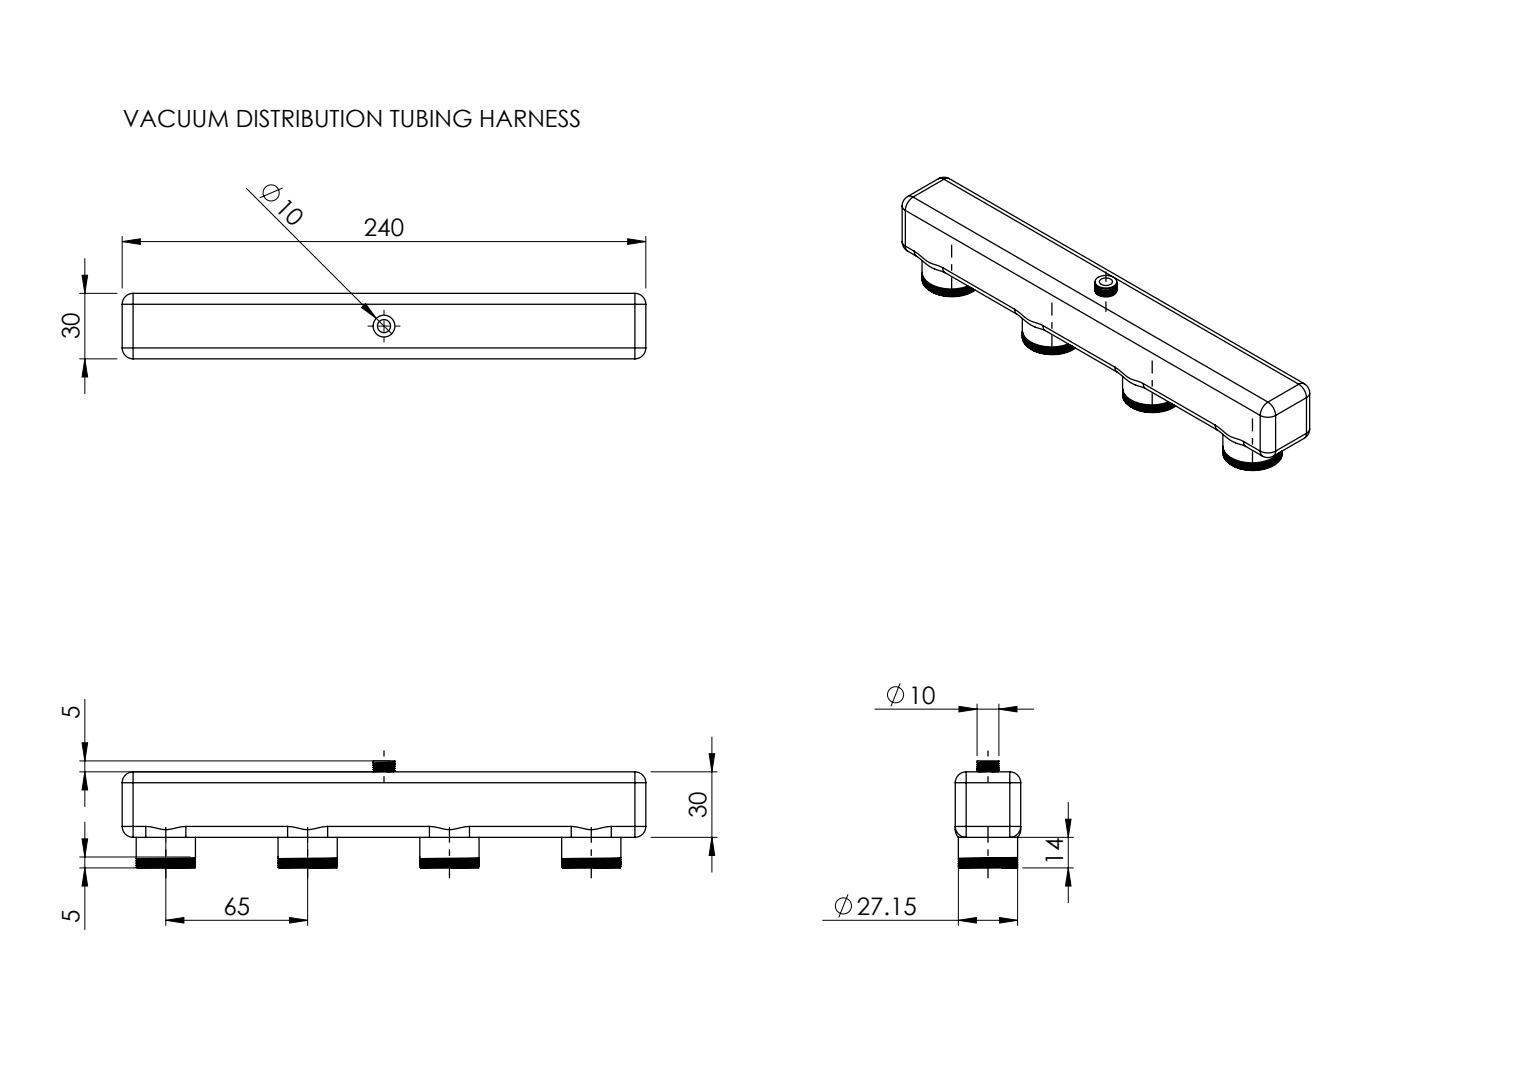
ISO-10303-21;
HEADER;
FILE_DESCRIPTION (('STEP AP214'),
    '1' );
FILE_NAME ('Vacuum Distribution Tubing Harness.step',
    '2026-10-01T14:18:43',
    ( '' ),
    ( '' ),
    'SwSTEP 2.0',
    'SolidWorks 2026',
    '' );
FILE_SCHEMA (( 'AUTOMOTIVE_DESIGN' ));
ENDSEC;

DATA;
#1=ORIENTED_EDGE ( 'NONE', *, *, #27439, .T. ) ;
#2=CARTESIAN_POINT ( 'NONE',  ( 94.99999999999995737, 83.93750000000001421, -2.071067811865491048 ) ) ;
#4=ORIENTED_EDGE ( 'NONE', *, *, #23222, .F. ) ;
#6=CARTESIAN_POINT ( 'NONE',  ( 59.55508561352770158, 34.55078125108393294, 13.14518615778179722 ) ) ;
#10=EDGE_CURVE ( 'NONE', #23304, #14872, #10315, .T. ) ;
#14=CARTESIAN_POINT ( 'NONE',  ( 185.4011555911795597, 37.22968750216787726, 9.598844408820459861 ) ) ;
#17=CARTESIAN_POINT ( 'NONE',  ( 198.0446094569239790, 53.89089363584123049, 14.99999999999994671 ) ) ;
#18=CARTESIAN_POINT ( 'NONE',  ( 143.1451861577818363, 36.43593750108394147, -5.444914386472297529 ) ) ;
#19=ORIENTED_EDGE ( 'NONE', *, *, #9159, .T. ) ;
#20=CARTESIAN_POINT ( 'NONE',  ( 13.14518615778179544, 37.97382812608393721, -1.609821015232357215E-15 ) ) ;
#22=CARTESIAN_POINT ( 'NONE',  ( 143.1451861577818079, 35.39414062608393152, -1.609821015232357215E-15 ) ) ;
#23=CARTESIAN_POINT ( 'NONE',  ( 65.00000000000000000, 34.84843749999999574, 13.57481594606304576 ) ) ;
#24=CARTESIAN_POINT ( 'NONE',  ( 130.0000000000000000, -7.395377635281828788, -1.503427012513233026E-14 ) ) ;
#29=CARTESIAN_POINT ( 'NONE',  ( -8.312177448680279460E-16, 39.31328125216787583, -13.57481594606304576 ) ) ;
#30=CARTESIAN_POINT ( 'NONE',  ( 99.99999999999995737, 80.00000000000000000, -1.387778780781445676E-14 ) ) ;
#32=CARTESIAN_POINT ( 'NONE',  ( -9.295050272127046043, 35.89023437608393152, -9.295050272127046043 ) ) ;
#39=CARTESIAN_POINT ( 'NONE',  ( 195.0000000000000000, 37.97382812608393721, -13.14518615778179544 ) ) ;
#40=ORIENTED_EDGE ( 'NONE', *, *, #17022, .F. ) ;
#50=CARTESIAN_POINT ( 'NONE',  ( 143.1451861577818079, 39.31328125108392868, 5.444914386472293977 ) ) ;
#54=CARTESIAN_POINT ( 'NONE',  ( 78.14518615778179367, 39.51171875108392584, 5.444914386472293977 ) ) ;
#55=FACE_OUTER_BOUND ( 'NONE', #22673, .T. ) ;
#56=CIRCLE ( 'NONE', #18273, 5.000000000000000000 ) ;
#57=CARTESIAN_POINT ( 'NONE',  ( 181.8548138422181921, 33.65781250108393152, 5.444914386472304635 ) ) ;
#59=ORIENTED_EDGE ( 'NONE', *, *, #2461, .T. ) ;
#62=CARTESIAN_POINT ( 'NONE',  ( 51.85481384221820633, 38.96601562608393721, 0.000000000000000000 ) ) ;
#63=CARTESIAN_POINT ( 'NONE',  ( 99.99999999999995737, 80.18750000136559208, -4.458734125000016313 ) ) ;
#64=CARTESIAN_POINT ( 'NONE',  ( 189.5550856135277229, 39.61093750108393152, -13.14518615778179722 ) ) ;
#66=CARTESIAN_POINT ( 'NONE',  ( 187.8845096081555823, 49.99999999945637796, 11.58166858714721492 ) ) ;
#70=ORIENTED_EDGE ( 'NONE', *, *, #20702, .F. ) ;
#75=CARTESIAN_POINT ( 'NONE',  ( 143.1451861577818079, 34.79882812608394005, -1.609821015232357215E-15 ) ) ;
#76=CARTESIAN_POINT ( 'NONE',  ( 59.55508561352770158, 32.76484375108393010, 13.14518615778179722 ) ) ;
#77=CARTESIAN_POINT ( 'NONE',  ( 208.1451861577817795, 38.71796875108393721, 5.444914386472293977 ) ) ;
#78=CARTESIAN_POINT ( 'NONE',  ( 9.295050272127047819, 32.91367187608393152, 9.295050272127046043 ) ) ;
#79=CARTESIAN_POINT ( 'NONE',  ( 134.5715916325255250, 51.44262710532316873, -14.99999999999934452 ) ) ;
#82=CARTESIAN_POINT ( 'NONE',  ( -9.180175813647991845, 50.00000000000000000, 9.999999999999998224 ) ) ;
#84=EDGE_CURVE ( 'NONE', #861, #22018, #1572, .T. ) ;
#85=CARTESIAN_POINT ( 'NONE',  ( 13.14518615778179544, 33.80664062608393294, -1.609821015232357215E-15 ) ) ;
#96=ADVANCED_FACE ( 'NONE', ( #24479 ), #13627, .T. ) ;
#98=CARTESIAN_POINT ( 'NONE',  ( 120.4011555911795455, 38.61875000216787157, -9.598844408820458085 ) ) ;
#99=CARTESIAN_POINT ( 'NONE',  ( 103.1528011352953342, 80.06250000136559208, 3.152801135295355106 ) ) ;
#100=CARTESIAN_POINT ( 'NONE',  ( 78.14518615778179367, 34.05468750108394005, -5.444914386472297529 ) ) ;
#103=CARTESIAN_POINT ( 'NONE',  ( 214.9999999999999716, 80.00000000000000000, 9.999999999999946709 ) ) ;
#105=CARTESIAN_POINT ( 'NONE',  ( 143.5748159460630404, 39.06523437499998863, -5.622872871577873077 ) ) ;
#110=CARTESIAN_POINT ( 'NONE',  ( 143.1451861577818079, 37.82500000108392868, -5.444914386472297529 ) ) ;
#111=CARTESIAN_POINT ( 'NONE',  ( 51.42518405393695957, 33.16171875216787868, 0.000000000000000000 ) ) ;
#112=EDGE_CURVE ( 'NONE', #21487, #10978, #25380, .T. ) ;
#114=CARTESIAN_POINT ( 'NONE',  ( 13.57481594606304931, 32.71523437716787441, 5.622872871577869525 ) ) ;
#117=CARTESIAN_POINT ( 'NONE',  ( 185.7049497278729575, 34.10429687608393579, -9.295050272127046043 ) ) ;
#121=CARTESIAN_POINT ( 'NONE',  ( 181.4251840539369596, 37.97382812716787726, 5.622872871577880183 ) ) ;
#122=LINE ( 'NONE', #8807, #24532 ) ;
#128=CARTESIAN_POINT ( 'NONE',  ( 195.0000000000000000, 35.24531249999999716, -13.57481594606304576 ) ) ;
#131=CARTESIAN_POINT ( 'NONE',  ( 59.55508561352770158, 35.14609375108393152, 13.14518615778179722 ) ) ;
#136=CARTESIAN_POINT ( 'NONE',  ( 13.57481594606304753, 36.68398437499999432, -5.622872871577873077 ) ) ;
#137=CARTESIAN_POINT ( 'NONE',  ( 130.0000000000000000, 36.58476562608393579, -13.14518615778179544 ) ) ;
#139=ORIENTED_EDGE ( 'NONE', *, *, #6013, .F. ) ;
#140=CARTESIAN_POINT ( 'NONE',  ( 99.99999999999995737, 84.75000000000000000, -5.000000000000018652 ) ) ;
#141=CARTESIAN_POINT ( 'NONE',  ( 94.99999999999995737, 82.06250000273119838, -2.071067811865491048 ) ) ;
#144=VERTEX_POINT ( 'NONE', #11771 ) ;
#145=AXIS2_PLACEMENT_3D ( 'NONE', #183, #21567, #25834 ) ;
#147=CARTESIAN_POINT ( 'NONE',  ( 70.44491438647230552, 33.85625000108393579, 13.14518615778179189 ) ) ;
#151=EDGE_CURVE ( 'NONE', #14316, #1074, #18349, .T. ) ;
#152=VERTEX_POINT ( 'NONE', #22777 ) ;
#153=CARTESIAN_POINT ( 'NONE',  ( 94.99999999999995737, 82.18750000273119838, 2.071067811865466624 ) ) ;
#156=CARTESIAN_POINT ( 'NONE',  ( 208.5748159460630120, 35.09648437716787583, 5.622872871577869525 ) ) ;
#157=( BOUNDED_CURVE ( )  B_SPLINE_CURVE ( 2, ( #25854, #26427, #8886, #8604, #23721, #4618, #22006, #19716, #2060, #6886, #24002, #4059, #2483, #19859, #12721, #10593, #17292, #17435, #26134, #346, #10730, #19438, #6600, #9033, #21447, #25994, #1925, #6465, #15139, #2204, #10868, #19578, #62, #5047, #2628, #15857, #775, #22576, #24851, #11571, #920, #7307, #13712, #7161, #13851, #491, #24419, #5188, #9172, #22433, #27146, #631, #15994, #4908, #9447, #11713, #24566, #3045, #9307, #11289, #17864, #20289, #22720, #26569, #9590, #18004, #2902, #24709, #20438, #7598, #18294, #7021, #27000, #7447, #16143, #22292, #24280, #5330, #4761, #13994, #3187, #13569, #11857, #20579, #2768, #26861, #18147, #1062, #15716, #9732, #18437, #13421, #11432 ),
 .UNSPECIFIED., .F., .F. ) 
 B_SPLINE_CURVE_WITH_KNOTS ( ( 3, 2, 2, 2, 2, 2, 2, 2, 2, 2, 2, 2, 2, 2, 2, 2, 2, 2, 2, 2, 2, 2, 2, 2, 2, 2, 2, 2, 2, 2, 2, 2, 2, 2, 2, 2, 2, 2, 2, 2, 2, 2, 2, 2, 2, 2, 3 ),
 ( 0.000000000000000000, 0.01041666666666666609, 0.02083333333333333218, 0.03125000000000000000, 0.04166666666666666435, 0.05208333333333333565, 0.06250000000000000000, 0.07291666666666667129, 0.08333333333333332871, 0.09375000000000000000, 0.1041666666666666713, 0.1145833333333333287, 0.1250000000000000000, 0.1354166666666666574, 0.1458333333333333426, 0.1562500000000000278, 0.1666666666666666574, 0.1770833333333333426, 0.1875000000000000000, 0.1979166666666666574, 0.2083333333333333426, 0.2187499999999999722, 0.2291666666666666574, 0.2395833333333333426, 0.2500000000000000000, 0.2604166666666666852, 0.2708333333333333148, 0.2812500000000000000, 0.2916666666666666852, 0.3020833333333333148, 0.3125000000000000555, 0.3229166666666666852, 0.3333333333333333148, 0.3437500000000000000, 0.3541666666666666852, 0.3645833333333333148, 0.3750000000000000000, 0.3854166666666666852, 0.3958333333333333148, 0.4062500000000000000, 0.4166666666666666852, 0.4270833333333333148, 0.4374999999999999445, 0.4479166666666666852, 0.4583333333333333148, 0.4687500000000000000, 0.4779971559588573893 ),
 .UNSPECIFIED. ) 
 CURVE ( )  GEOMETRIC_REPRESENTATION_ITEM ( )  RATIONAL_B_SPLINE_CURVE ( ( 1.000000000000000000, 0.9238795325112867385, 1.000000000000000000, 0.9238795325112867385, 1.000000000000000000, 0.9238795325112867385, 1.000000000000000000, 0.9238795325112867385, 1.000000000000000000, 0.9238795325112867385, 1.000000000000000000, 0.9238795325112867385, 1.000000000000000000, 0.9238795325112867385, 1.000000000000000000, 0.9238795325112867385, 1.000000000000000000, 0.9238795325112867385, 1.000000000000000000, 0.9238795325112867385, 1.000000000000000000, 0.9238795325112867385, 1.000000000000000000, 0.9238795325112867385, 1.000000000000000000, 0.9238795325112867385, 1.000000000000000000, 0.9238795325112867385, 1.000000000000000000, 0.9238795325112867385, 1.000000000000000000, 0.9238795325112867385, 1.000000000000000000, 0.9238795325112867385, 1.000000000000000000, 0.9238795325112867385, 1.000000000000000000, 0.9238795325112867385, 1.000000000000000000, 0.9238795325112867385, 1.000000000000000000, 0.9238795325112867385, 1.000000000000000000, 0.9238795325112867385, 1.000000000000000000, 0.9238795325112867385, 1.000000000000000000, 0.9238795325112867385, 1.000000000000000000, 0.9238795325112867385, 1.000000000000000000, 0.9238795325112867385, 1.000000000000000000, 0.9238795325112867385, 1.000000000000000000, 0.9238795325112867385, 1.000000000000000000, 0.9238795325112867385, 1.000000000000000000, 0.9238795325112867385, 1.000000000000000000, 0.9238795325112867385, 1.000000000000000000, 0.9238795325112867385, 1.000000000000000000, 0.9238795325112867385, 1.000000000000000000, 0.9238795325112867385, 1.000000000000000000, 0.9238795325112867385, 1.000000000000000000, 0.9238795325112867385, 1.000000000000000000, 0.9238795325112867385, 1.000000000000000000, 0.9238795325112867385, 1.000000000000000000, 0.9238795325112867385, 1.000000000000000000, 0.9238795325112867385, 1.000000000000000000, 0.9238795325112867385, 1.000000000000000000, 0.9238795325112867385, 1.000000000000000000, 0.9238795325112867385, 1.000000000000000000, 0.9238795325112867385, 1.000000000000000000, 0.9238795325112867385, 1.000000000000000000, 0.9324258078851906939, 0.9848264816800322841 ) ) 
 REPRESENTATION_ITEM ( '' )  );
#160=EDGE_CURVE ( 'NONE', #17655, #15436, #3245, .T. ) ;
#161=CARTESIAN_POINT ( 'NONE',  ( 204.5988444088204687, 39.80937500216786873, 9.598844408820456309 ) ) ;
#163=CARTESIAN_POINT ( 'NONE',  ( -13.14518615778179189, 36.83281250108393579, 5.444914386472304635 ) ) ;
#164=CARTESIAN_POINT ( 'NONE',  ( 130.0000000000000000, 36.38632812608393152, -13.14518615778179544 ) ) ;
#165=CARTESIAN_POINT ( 'NONE',  ( 65.00000000000000000, 35.64218749999999147, 13.57481594606304576 ) ) ;
#166=CARTESIAN_POINT ( 'NONE',  ( 9.598844408820456309, 38.42031250216787441, -9.598844408820458085 ) ) ;
#168=AXIS2_PLACEMENT_3D ( 'NONE', #6488, #12746, #4083 ) ;
#169=CARTESIAN_POINT ( 'NONE',  ( 195.0000000000000000, 37.22968749999999716, 13.57481594606304576 ) ) ;
#173=DIRECTION ( 'NONE',  ( 1.000000000000000000, 0.000000000000000000, 0.000000000000000000 ) ) ;
#175=CARTESIAN_POINT ( 'NONE',  ( -13.14518615778179900, 36.73359375108393010, -5.444914386472297529 ) ) ;
#180=LINE ( 'NONE', #8862, #20235 ) ;
#181=CARTESIAN_POINT ( 'NONE',  ( 185.7049497278729575, 38.27148437608393294, 9.295050272127047819 ) ) ;
#183=CARTESIAN_POINT ( 'NONE',  ( 0.000000000000000000, -7.395377635281828788, 0.000000000000000000 ) ) ;
#184=CARTESIAN_POINT ( 'NONE',  ( 189.6826484225240677, 54.47013368152370560, -15.00000000000000000 ) ) ;
#185=CARTESIAN_POINT ( 'NONE',  ( 143.5748159460630688, 39.85898437499999858, -5.622872871577873966 ) ) ;
#186=ORIENTED_EDGE ( 'NONE', *, *, #18586, .T. ) ;
#188=CARTESIAN_POINT ( 'NONE',  ( 130.0000000000000000, 37.62656249999999858, -13.57481594606304576 ) ) ;
#190=CARTESIAN_POINT ( 'NONE',  ( 130.0000000000000000, 31.37578125216787583, -13.57481594606304576 ) ) ;
#191=CARTESIAN_POINT ( 'NONE',  ( 13.14518615778179722, 40.30546875108393579, 5.444914386472293977 ) ) ;
#193=CARTESIAN_POINT ( 'NONE',  ( 51.85481384221820633, 37.57695312608393579, 0.000000000000000000 ) ) ;
#195=CARTESIAN_POINT ( 'NONE',  ( 189.5550856135277229, 36.13828125108393863, 13.14518615778179722 ) ) ;
#197=( BOUNDED_CURVE ( )  B_SPLINE_CURVE ( 2, ( #21878, #15145, #8893, #6748, #2489, #2066, #15434, #19866, #10736 ),
 .UNSPECIFIED., .F., .F. ) 
 B_SPLINE_CURVE_WITH_KNOTS ( ( 3, 2, 2, 2, 3 ),
 ( 0.1041666666666664909, 0.1145833333333332732, 0.1250000000000000833, 0.1354166666666668517, 0.1458333333333336757 ),
 .UNSPECIFIED. ) 
 CURVE ( )  GEOMETRIC_REPRESENTATION_ITEM ( )  RATIONAL_B_SPLINE_CURVE ( ( 1.000000000000001332, 0.9238795325112854062, 1.000000000000000000, 0.9238795325112867385, 1.000000000000000000, 0.9238795325112867385, 1.000000000000000000, 0.9238795325112842960, 1.000000000000002442 ) ) 
 REPRESENTATION_ITEM ( '' )  );
#198=ORIENTED_EDGE ( 'NONE', *, *, #2542, .F. ) ;
#202=CARTESIAN_POINT ( 'NONE',  ( 101.8468681455907046, 80.12500000136560629, -4.458734125000016313 ) ) ;
#203=CARTESIAN_POINT ( 'NONE',  ( 208.1451861577818079, 38.61875000108392442, -5.444914386472297529 ) ) ;
#206=CARTESIAN_POINT ( 'NONE',  ( 186.5976842187810973, 54.99999999484811752, 14.99999999999995026 ) ) ;
#208=DIRECTION ( 'NONE',  ( 0.000000000000000000, 0.000000000000000000, 1.000000000000000000 ) ) ;
#214=CARTESIAN_POINT ( 'NONE',  ( 116.8548138422182063, 35.93984375108393436, -5.444914386472297529 ) ) ;
#215=CARTESIAN_POINT ( 'NONE',  ( 78.14518615778179367, 33.75703125108393010, 5.444914386472293977 ) ) ;
#216=CARTESIAN_POINT ( 'NONE',  ( 189.5550856135277229, 35.84062500108394289, -13.14518615778179900 ) ) ;
#218=CARTESIAN_POINT ( 'NONE',  ( 66.13716782454086740, 35.99999999999998579, 13.09590655363602707 ) ) ;
#220=FACE_OUTER_BOUND ( 'NONE', #12562, .T. ) ;
#222=CARTESIAN_POINT ( 'NONE',  ( 65.00000000000000000, 40.40468749999999432, 13.57481594606304576 ) ) ;
#226=CARTESIAN_POINT ( 'NONE',  ( 61.88530225446237409, 53.90847045361019241, 14.99999999999997868 ) ) ;
#228=( NAMED_UNIT ( * ) PLANE_ANGLE_UNIT ( ) SI_UNIT ( $, .RADIAN. ) );
#232=CARTESIAN_POINT ( 'NONE',  ( 131.8143553545780264, 51.46618445021973542, 14.99999999999996625 ) ) ;
#234=PLANE ( 'NONE',  #26801 ) ;
#235=CARTESIAN_POINT ( 'NONE',  ( 95.54126587499995082, 80.62500000136559208, -1.846868145590750077 ) ) ;
#236=CARTESIAN_POINT ( 'NONE',  ( 65.00000000000000000, 35.39414062608393863, 13.14518615778179544 ) ) ;
#238=CARTESIAN_POINT ( 'NONE',  ( -5.444914386472297529, 36.43593750108394147, -13.14518615778179722 ) ) ;
#239=EDGE_CURVE ( 'NONE', #2183, #6189, #25460, .T. ) ;
#241=CARTESIAN_POINT ( 'NONE',  ( 116.4251840539369596, 40.65273437608393436, 0.000000000000000000 ) ) ;
#243=CARTESIAN_POINT ( 'NONE',  ( 130.0000000000000000, 38.81718749999999574, 13.57481594606304576 ) ) ;
#246=EDGE_CURVE ( 'NONE', #18432, #1781, #20836, .T. ) ;
#249=CARTESIAN_POINT ( 'NONE',  ( 143.1451861577818079, 36.93203125108394147, 5.444914386472293977 ) ) ;
#250=CARTESIAN_POINT ( 'NONE',  ( 74.59884440882045453, 34.45156250216787441, -9.598844408820458085 ) ) ;
#251=ORIENTED_EDGE ( 'NONE', *, *, #21153, .F. ) ;
#254=CARTESIAN_POINT ( 'NONE',  ( 2.493653234604083739E-15, 32.56640625216787299, 13.57481594606304576 ) ) ;
#258=CARTESIAN_POINT ( 'NONE',  ( 189.5550856135277229, 35.14609375108393152, 13.14518615778179722 ) ) ;
#260=AXIS2_PLACEMENT_3D ( 'NONE', #16112, #26536, #3014 ) ;
#262=CARTESIAN_POINT ( 'NONE',  ( 99.99999999999995737, 81.25000000000000000, 4.999999999999990230 ) ) ;
#267=CARTESIAN_POINT ( 'NONE',  ( 139.5988444088204403, 38.32109374999999574, -9.598844408820458085 ) ) ;
#270=CARTESIAN_POINT ( 'NONE',  ( 208.5748159460630120, 35.09648437499998863, -5.622872871577873077 ) ) ;
#271=CARTESIAN_POINT ( 'NONE',  ( 204.1801758136480203, 55.00000000000014211, 9.999999999999948486 ) ) ;
#272=CARTESIAN_POINT ( 'NONE',  ( 139.5988444088204403, 36.73359374999999716, -9.598844408820458085 ) ) ;
#273=CARTESIAN_POINT ( 'NONE',  ( 74.29505027212704249, 35.49335937608393010, -9.295050272127046043 ) ) ;
#277=ADVANCED_FACE ( 'NONE', ( #16895 ), #6077, .T. ) ;
#278=DIRECTION ( 'NONE',  ( 0.000000000000000000, -1.000000000000000000, 0.000000000000000000 ) ) ;
#279=CARTESIAN_POINT ( 'NONE',  ( 2.493653234604083739E-15, 35.64218749999999147, 13.57481594606304576 ) ) ;
#280=CARTESIAN_POINT ( 'NONE',  ( 139.2950502721270425, 37.27929687608394005, -9.295050272127046043 ) ) ;
#283=CARTESIAN_POINT ( 'NONE',  ( 104.9999999999999574, 83.56250000000002842, -2.071067811865491937 ) ) ;
#284=CARTESIAN_POINT ( 'NONE',  ( 96.46446609406721961, 80.25000000273119838, 3.535533905932727539 ) ) ;
#287=CARTESIAN_POINT ( 'NONE',  ( 51.85082601884828080, 35.99999999999999289, -1.058935892997133088 ) ) ;
#290=CARTESIAN_POINT ( 'NONE',  ( 59.37712712842213136, 40.85117187499999147, -13.57481594606304753 ) ) ;
#291=VERTEX_POINT ( 'NONE', #25731 ) ;
#292=CARTESIAN_POINT ( 'NONE',  ( 139.5988444088204403, 39.21406250216787015, -9.598844408820458085 ) ) ;
#294=EDGE_CURVE ( 'NONE', #22062, #7806, #16625, .T. ) ;
#296=CARTESIAN_POINT ( 'NONE',  ( 120.8198241863519939, 50.00000000000000000, -9.999999999999998224 ) ) ;
#298=CARTESIAN_POINT ( 'NONE',  ( 181.4251840539369596, 33.90585937716787868, -5.622872871577873077 ) ) ;
#299=AXIS2_PLACEMENT_3D ( 'NONE', #13990, #23131, #5887 ) ;
#302=CARTESIAN_POINT ( 'NONE',  ( 143.1451861577818363, 37.13046875108393863, 5.444914386472293977 ) ) ;
#303=ORIENTED_EDGE ( 'NONE', *, *, #24870, .F. ) ;
#304=CARTESIAN_POINT ( 'NONE',  ( 9.295050272127046043, 34.89804687608393863, -9.295050272127046043 ) ) ;
#305=CARTESIAN_POINT ( 'NONE',  ( 124.5550856135277087, 35.14609375108393152, 13.14518615778179722 ) ) ;
#306=CARTESIAN_POINT ( 'NONE',  ( 59.37712712842213136, 35.29492187500000000, -13.57481594606304753 ) ) ;
#310=DIRECTION ( 'NONE',  ( -0.000000000000000000, 1.000000000000000000, -0.000000000000000000 ) ) ;
#316=CARTESIAN_POINT ( 'NONE',  ( 5.444914386472302859, 37.82500000108392868, 13.14518615778179189 ) ) ;
#318=ORIENTED_EDGE ( 'NONE', *, *, #24476, .T. ) ;
#320=( BOUNDED_CURVE ( )  B_SPLINE_CURVE ( 2, ( #29, #14971, #10973, #15395, #28107, #8572, #17262, #24107, #13244 ),
 .UNSPECIFIED., .F., .T. ) 
 B_SPLINE_CURVE_WITH_KNOTS ( ( 3, 2, 2, 2, 3 ),
 ( 0.1041666666666664909, 0.1145833333333332732, 0.1250000000000000833, 0.1354166666666668517, 0.1458333333333336757 ),
 .UNSPECIFIED. ) 
 CURVE ( )  GEOMETRIC_REPRESENTATION_ITEM ( )  RATIONAL_B_SPLINE_CURVE ( ( 1.000000000000001332, 0.9238795325112854062, 1.000000000000000000, 0.9238795325112867385, 1.000000000000000000, 0.9238795325112867385, 1.000000000000000000, 0.9238795325112842960, 1.000000000000002442 ) ) 
 REPRESENTATION_ITEM ( '' )  );
#321=AXIS2_PLACEMENT_3D ( 'NONE', #9134, #9413, #17827 ) ;
#325=CARTESIAN_POINT ( 'NONE',  ( 181.8548138422181921, 39.01562500108393294, 5.444914386472304635 ) ) ;
#326=ORIENTED_EDGE ( 'NONE', *, *, #10011, .F. ) ;
#327=CARTESIAN_POINT ( 'NONE',  ( 135.6228728715780107, 36.08867187716787583, -13.57481594606290898 ) ) ;
#333=CARTESIAN_POINT ( 'NONE',  ( 143.5748159460630404, 31.92148437716787512, 5.622872871577869525 ) ) ;
#334=DIRECTION ( 'NONE',  ( -0.000000000000000000, 1.000000000000000000, -0.000000000000000000 ) ) ;
#337=CARTESIAN_POINT ( 'NONE',  ( 74.29505027212704249, 37.87460937608393863, 9.295050272127046043 ) ) ;
#338=CARTESIAN_POINT ( 'NONE',  ( 64.55395874322236693, 49.99999999978093257, -13.57776691409252656 ) ) ;
#339=CARTESIAN_POINT ( 'NONE',  ( 189.3771271284221314, 40.35507812499998437, 13.57481594606304753 ) ) ;
#340=CARTESIAN_POINT ( 'NONE',  ( 77.25119088044421289, 35.99999999999997158, 5.405483146088426061 ) ) ;
#346=CARTESIAN_POINT ( 'NONE',  ( 59.55508561352770158, 39.61093750108393152, -13.14518615778179722 ) ) ;
#347=CARTESIAN_POINT ( 'NONE',  ( 103.1528011352953342, 82.81250000136560629, 3.152801135295355106 ) ) ;
#348=CARTESIAN_POINT ( 'NONE',  ( 189.5550856135277229, 38.32109375108394289, 13.14518615778179722 ) ) ;
#350=CARTESIAN_POINT ( 'NONE',  ( 186.7886859848165102, 50.68678854790359622, 14.99999999999995737 ) ) ;
#351=DIRECTION ( 'NONE',  ( 0.000000000000000000, 0.000000000000000000, -1.000000000000000000 ) ) ;
#352=CARTESIAN_POINT ( 'NONE',  ( 208.1451861577818079, 40.40468750108393436, -5.444914386472297529 ) ) ;
#357=ORIENTED_EDGE ( 'NONE', *, *, #27287, .T. ) ;
#358=CARTESIAN_POINT ( 'NONE',  ( 116.8548138422182063, 34.35234375108393579, -5.444914386472297529 ) ) ;
#360=CARTESIAN_POINT ( 'NONE',  ( 74.29505027212704249, 34.69960937608393436, -9.295050272127046043 ) ) ;
#361=CARTESIAN_POINT ( 'NONE',  ( 181.8548138422182205, 38.37070312608393152, 0.000000000000000000 ) ) ;
#362=ORIENTED_EDGE ( 'NONE', *, *, #430, .T. ) ;
#363=CARTESIAN_POINT ( 'NONE',  ( 99.99999999999995737, 80.00000000000000000, -1.387778780781445676E-14 ) ) ;
#364=CARTESIAN_POINT ( 'NONE',  ( 5.444914386472302859, 32.07031250108393294, 13.14518615778179189 ) ) ;
#366=CARTESIAN_POINT ( 'NONE',  ( 78.57481594606305464, 40.65273437499999432, -5.622872871577873966 ) ) ;
#368=EDGE_CURVE ( 'NONE', #4636, #22369, #10615, .T. ) ;
#369=( BOUNDED_CURVE ( )  B_SPLINE_CURVE ( 2, ( #25306, #14184, #6305, #9907, #1384, #3231, #14981, #3653, #12315 ),
 .UNSPECIFIED., .F., .F. ) 
 B_SPLINE_CURVE_WITH_KNOTS ( ( 3, 2, 2, 2, 3 ),
 ( 0.05000000000000004441, 0.07500000000000006661, 0.1000000000000000888, 0.1250000000000001110, 0.1500000000000001332 ),
 .UNSPECIFIED. ) 
 CURVE ( )  GEOMETRIC_REPRESENTATION_ITEM ( )  RATIONAL_B_SPLINE_CURVE ( ( 0.9999999999999998890, 0.9238795325112868495, 1.000000000000000000, 0.9238795325112867385, 1.000000000000000000, 0.9238795325112867385, 1.000000000000000000, 0.9238795325112862944, 1.000000000000000444 ) ) 
 REPRESENTATION_ITEM ( '' )  );
#373=CARTESIAN_POINT ( 'NONE',  ( 57.88450960814756030, 49.99999999945625717, 11.58166858714126235 ) ) ;
#382=CARTESIAN_POINT ( 'NONE',  ( 95.54126587499995082, 82.75000000136560629, 1.846868145590724986 ) ) ;
#383=CARTESIAN_POINT ( 'NONE',  ( 65.00000000000000000, 36.18789062608393436, 13.14518615778179544 ) ) ;
#385=CARTESIAN_POINT ( 'NONE',  ( -13.14518615778179544, 36.58476562608393579, 0.000000000000000000 ) ) ;
#390=CARTESIAN_POINT ( 'NONE',  ( 116.4251840539369454, 37.77539062499999289, -5.622872871577873077 ) ) ;
#392=ORIENTED_EDGE ( 'NONE', *, *, #14583, .T. ) ;
#397=CARTESIAN_POINT ( 'NONE',  ( 124.5550856135277087, 37.52734375108393294, 13.14518615778179722 ) ) ;
#398=CARTESIAN_POINT ( 'NONE',  ( 51.42518405393695957, 33.11210937716786873, -5.622872871577873077 ) ) ;
#401=CARTESIAN_POINT ( 'NONE',  ( -13.57481594606304576, 33.95546875216787441, 0.000000000000000000 ) ) ;
#402=CIRCLE ( 'NONE', #16324, 11.57481594606304398 ) ;
#404=AXIS2_PLACEMENT_3D ( 'NONE', #9924, #14615, #3535 ) ;
#405=CARTESIAN_POINT ( 'NONE',  ( 181.8548138422182205, 34.99726562608393721, 0.000000000000000000 ) ) ;
#408=CARTESIAN_POINT ( 'NONE',  ( 189.3771271284220745, 40.05742187499998863, -13.57481594606297293 ) ) ;
#410=CARTESIAN_POINT ( 'NONE',  ( 120.8198241863519939, 55.00000000000000000, 14.99999999999996803 ) ) ;
#412=CARTESIAN_POINT ( 'NONE',  ( 135.6228728715778118, 38.07304687499999574, 13.57481594606313813 ) ) ;
#415=CARTESIAN_POINT ( 'NONE',  ( 181.4251840539369596, 33.11210937499999574, 5.622872871577880183 ) ) ;
#417=CARTESIAN_POINT ( 'NONE',  ( 70.44491438647230552, 36.83281250108392868, 13.14518615778179189 ) ) ;
#421=CARTESIAN_POINT ( 'NONE',  ( -9.598844408820454532, 34.74921874999999716, 9.598844408820459861 ) ) ;
#422=CARTESIAN_POINT ( 'NONE',  ( 143.1451861577818079, 38.76757812608393294, -1.609821015232357215E-15 ) ) ;
#423=ORIENTED_EDGE ( 'NONE', *, *, #17964, .T. ) ;
#424=CARTESIAN_POINT ( 'NONE',  ( 102.0710678118654329, 82.68750000000001421, -5.000000000000018652 ) ) ;
#425=CARTESIAN_POINT ( 'NONE',  ( 219.9999999999999716, 50.00000000000000000, -10.00000000000000000 ) ) ;
#426=CARTESIAN_POINT ( 'NONE',  ( 103.5355339059327093, 83.50000000273119838, 3.535533905932726206 ) ) ;
#430=EDGE_CURVE ( 'NONE', #1457, #22555, #4820, .T. ) ;
#432=CARTESIAN_POINT ( 'NONE',  ( 59.37712712842213136, 39.56132812499999574, 13.57481594606304753 ) ) ;
#436=EDGE_LOOP ( 'NONE', ( #17651, #5409, #22660, #15371, #2602 ) ) ;
#438=CARTESIAN_POINT ( 'NONE',  ( 189.3771271284221314, 33.31054687716787299, 13.57481594606304753 ) ) ;
#439=VERTEX_POINT ( 'NONE', #6346 ) ;
#440=EDGE_CURVE ( 'NONE', #5976, #21288, #23550, .T. ) ;
#443=CARTESIAN_POINT ( 'NONE',  ( 124.5550856135277087, 36.93203125108394147, 13.14518615778179722 ) ) ;
#444=VERTEX_POINT ( 'NONE', #16759 ) ;
#445=CARTESIAN_POINT ( 'NONE',  ( 13.14518615778179900, 33.95546875108393436, 5.444914386472293977 ) ) ;
#447=CARTESIAN_POINT ( 'NONE',  ( 120.7049497278729575, 32.51679687608393721, -9.295050272127046043 ) ) ;
#448=CARTESIAN_POINT ( 'NONE',  ( 78.57481594606304043, 34.30273437500000000, -5.622872871577873077 ) ) ;
#450=AXIS2_PLACEMENT_3D ( 'NONE', #25758, #24046, #13329 ) ;
#453=FACE_OUTER_BOUND ( 'NONE', #21146, .T. ) ;
#457=CARTESIAN_POINT ( 'NONE',  ( 102.0710678118654187, 83.81250000273119838, -5.000000000000015987 ) ) ;
#459=CARTESIAN_POINT ( 'NONE',  ( -5.444914386472299306, 36.13828125108393863, 13.14518615778179722 ) ) ;
#462=ORIENTED_EDGE ( 'NONE', *, *, #14982, .F. ) ;
#466=CARTESIAN_POINT ( 'NONE',  ( 189.5550856135277229, 37.22968750108393721, -13.14518615778179900 ) ) ;
#467=VERTEX_POINT ( 'NONE', #26304 ) ;
#468=CARTESIAN_POINT ( 'NONE',  ( 13.57481594606304753, 39.95820312716787726, -5.622872871577873966 ) ) ;
#477=CARTESIAN_POINT ( 'NONE',  ( 143.5748159460630688, 32.76484375216787015, -1.662435489736055892E-15 ) ) ;
#478=CARTESIAN_POINT ( 'NONE',  ( 9.295050272127047819, 39.46210937608393721, 9.295050272127046043 ) ) ;
#479=EDGE_CURVE ( 'NONE', #25975, #2330, #24301, .T. ) ;
#481=CARTESIAN_POINT ( 'NONE',  ( 55.70494972787295751, 38.27148437608393294, -9.295050272127046043 ) ) ;
#482=CARTESIAN_POINT ( 'NONE',  ( 62.97537227446170505, 50.00000000051003468, -13.43320860980927201 ) ) ;
#485=CARTESIAN_POINT ( 'NONE',  ( 189.5550856135277229, 31.87187500108393223, -13.14518615778179900 ) ) ;
#491=CARTESIAN_POINT ( 'NONE',  ( 59.55508561352770158, 38.32109375108394289, 13.14518615778179722 ) ) ;
#492=DIRECTION ( 'NONE',  ( -0.000000000000000000, 1.000000000000000000, -0.000000000000000000 ) ) ;
#494=AXIS2_PLACEMENT_3D ( 'NONE', #24, #21266, #25957 ) ;
#497=CARTESIAN_POINT ( 'NONE',  ( 200.4449143864723055, 36.53515625108394715, -13.14518615778179722 ) ) ;
#503=CARTESIAN_POINT ( 'NONE',  ( 116.8548138422182063, 32.07031250108393294, 5.444914386472304635 ) ) ;
#504=CARTESIAN_POINT ( 'NONE',  ( 51.85481384221820633, 35.04687500108393294, 5.444914386472304635 ) ) ;
#505=CARTESIAN_POINT ( 'NONE',  ( 208.1451861577818079, 36.38632812608393863, -1.609821015232357215E-15 ) ) ;
#506=VERTEX_POINT ( 'NONE', #11310 ) ;
#508=CARTESIAN_POINT ( 'NONE',  ( -9.295050272127044266, 33.50898437608393010, 9.295050272127047819 ) ) ;
#511=CARTESIAN_POINT ( 'NONE',  ( 124.3771271284221314, 39.36289062716787157, -13.57481594606304753 ) ) ;
#515=CARTESIAN_POINT ( 'NONE',  ( 208.1451861577817795, 39.61093750108393863, -5.444914386472297529 ) ) ;
#518=ORIENTED_EDGE ( 'NONE', *, *, #16489, .T. ) ;
#521=CARTESIAN_POINT ( 'NONE',  ( 139.1801758136480203, 50.00000000000000000, 9.999999999999953815 ) ) ;
#523=CARTESIAN_POINT ( 'NONE',  ( 74.59884440882045453, 39.01562500216787299, 9.598844408820456309 ) ) ;
#525=CARTESIAN_POINT ( 'NONE',  ( 59.55508561352770158, 35.34453125108393579, 13.14518615778179722 ) ) ;
#527=CARTESIAN_POINT ( 'NONE',  ( 5.444914386472297529, 38.71796875108393721, -13.14518615778179722 ) ) ;
#529=CARTESIAN_POINT ( 'NONE',  ( 6.085944215996224038, 54.65299103241510892, 14.99999999999999289 ) ) ;
#531=CARTESIAN_POINT ( 'NONE',  ( 139.5988444088204403, 37.52734375000000000, -9.598844408820458085 ) ) ;
#533=EDGE_LOOP ( 'NONE', ( #3888, #18754, #1481 ) ) ;
#534=DIRECTION ( 'NONE',  ( 0.000000000000000000, -1.000000000000000000, 0.000000000000000000 ) ) ;
#538=CARTESIAN_POINT ( 'NONE',  ( 124.5550856135277087, 33.55859375108393294, 13.14518615778179722 ) ) ;
#539=CARTESIAN_POINT ( 'NONE',  ( 51.42518405393695957, 34.69960937716787441, -5.622872871577873077 ) ) ;
#540=VERTEX_POINT ( 'NONE', #15739 ) ;
#541=( BOUNDED_CURVE ( )  B_SPLINE_CURVE ( 2, ( #6091, #14214, #10070, #8082, #18782 ),
 .UNSPECIFIED., .F., .F. ) 
 B_SPLINE_CURVE_WITH_KNOTS ( ( 3, 2, 3 ),
 ( 0.9500000000000009548, 0.9750000000000005329, 1.000000000000000000 ),
 .UNSPECIFIED. ) 
 CURVE ( )  GEOMETRIC_REPRESENTATION_ITEM ( )  RATIONAL_B_SPLINE_CURVE ( ( 0.9999999999999970024, 0.9238795325112897361, 1.000000000000000000, 0.9238795325112867385, 1.000000000000000000 ) ) 
 REPRESENTATION_ITEM ( '' )  );
#542=CARTESIAN_POINT ( 'NONE',  ( 219.9999999999999716, 55.00000000000000000, 14.99999999999994316 ) ) ;
#543=CARTESIAN_POINT ( 'NONE',  ( 13.57481594606304576, 32.76484375216787015, -1.662435489736055892E-15 ) ) ;
#547=CARTESIAN_POINT ( 'NONE',  ( 181.8548138422182205, 33.40976562608393863, 0.000000000000000000 ) ) ;
#552=CARTESIAN_POINT ( 'NONE',  ( 116.4251840539369596, 36.33671875216787583, 0.000000000000000000 ) ) ;
#553=FACE_OUTER_BOUND ( 'NONE', #16139, .T. ) ;
#558=CARTESIAN_POINT ( 'NONE',  ( 181.4251840539369596, 33.90585937500000568, 5.622872871577880183 ) ) ;
#562=CARTESIAN_POINT ( 'NONE',  ( 55.70494972787295751, 35.89023437608393152, 9.295050272127047819 ) ) ;
#563=CARTESIAN_POINT ( 'NONE',  ( 99.99999999999995737, 85.00000000000000000, -1.387778780781445676E-14 ) ) ;
#564=DIRECTION ( 'NONE',  ( -0.000000000000000000, 1.000000000000000000, -0.000000000000000000 ) ) ;
#567=CARTESIAN_POINT ( 'NONE',  ( -9.598844408820458085, 35.34453124999998863, -9.598844408820458085 ) ) ;
#568=CARTESIAN_POINT ( 'NONE',  ( 143.1451861577818079, 38.81718750108393579, -5.444914386472297529 ) ) ;
#569=ORIENTED_EDGE ( 'NONE', *, *, #14895, .T. ) ;
#570=CARTESIAN_POINT ( 'NONE',  ( 102.0710678118654329, 81.68750000000000000, -5.000000000000018652 ) ) ;
#573=CARTESIAN_POINT ( 'NONE',  ( 103.5355339059327093, 83.75000000273119838, -3.535533905932755072 ) ) ;
#577=CARTESIAN_POINT ( 'NONE',  ( 70.62287287157786864, 40.75195312500000711, -13.57481594606304753 ) ) ;
#585=CARTESIAN_POINT ( 'NONE',  ( 185.4011555911795313, 33.06250000216787299, -9.598844408820458085 ) ) ;
#587=CARTESIAN_POINT ( 'NONE',  ( 200.6228728715780107, 36.08867187716787583, -13.57481594606290898 ) ) ;
#589=CARTESIAN_POINT ( 'NONE',  ( 13.14518615778179900, 35.64218750108393152, -5.444914386472297529 ) ) ;
#590=CARTESIAN_POINT ( 'NONE',  ( 116.8548138422182205, 31.82226562608393650, 0.000000000000000000 ) ) ;
#591=CARTESIAN_POINT ( 'NONE',  ( 65.00000000000000000, 33.26093749999999716, 13.57481594606304576 ) ) ;
#593=CARTESIAN_POINT ( 'NONE',  ( 122.9316343120017194, 36.00000000000003553, 11.09140360074130705 ) ) ;
#595=CARTESIAN_POINT ( 'NONE',  ( 207.0772764098356049, 36.00000000000000000, -6.197985357349214297 ) ) ;
#601=CARTESIAN_POINT ( 'NONE',  ( 5.444914386472297529, 37.32890625108393579, -13.14518615778179900 ) ) ;
#608=EDGE_CURVE ( 'NONE', #15564, #13869, #4643, .T. ) ;
#609=CARTESIAN_POINT ( 'NONE',  ( 208.1451861577818079, 35.39414062608393152, -1.609821015232357215E-15 ) ) ;
#610=ORIENTED_EDGE ( 'NONE', *, *, #1683, .F. ) ;
#611=CARTESIAN_POINT ( 'NONE',  ( 203.4023157812191300, 54.99999999485618929, -14.99999999999999645 ) ) ;
#618=EDGE_CURVE ( 'NONE', #28009, #5791, #13088, .T. ) ;
#619=CARTESIAN_POINT ( 'NONE',  ( 120.7049497278729575, 38.86679687608393863, -9.295050272127046043 ) ) ;
#620=LINE ( 'NONE', #26269, #12057 ) ;
#621=CARTESIAN_POINT ( 'NONE',  ( 5.444914386472297529, 35.54296875108393294, -13.14518615778179900 ) ) ;
#624=CARTESIAN_POINT ( 'NONE',  ( 78.14518615778179367, 38.02343750108395426, -5.444914386472297529 ) ) ;
#625=CARTESIAN_POINT ( 'NONE',  ( 55.81982418635199394, 49.99999999999999289, -14.99999999999999822 ) ) ;
#627=CARTESIAN_POINT ( 'NONE',  ( 181.8548138422182205, 32.81445312608393294, 0.000000000000000000 ) ) ;
#631=CARTESIAN_POINT ( 'NONE',  ( 59.55508561352770158, 38.02343750108394005, -13.14518615778179722 ) ) ;
#633=CARTESIAN_POINT ( 'NONE',  ( 65.00000000000000000, 38.81718749999999574, 13.57481594606304576 ) ) ;
#634=CARTESIAN_POINT ( 'NONE',  ( 208.1451861577818079, 36.18789062608393436, -1.609821015232357215E-15 ) ) ;
#635=EDGE_LOOP ( 'NONE', ( #198, #4757, #6902, #2298 ) ) ;
#639=CARTESIAN_POINT ( 'NONE',  ( 181.8548138422182205, 38.32109375108394289, -5.444914386472297529 ) ) ;
#646=CARTESIAN_POINT ( 'NONE',  ( 130.0000000000000000, 33.80664062608393294, 13.14518615778179544 ) ) ;
#647=CARTESIAN_POINT ( 'NONE',  ( 70.44491438647230552, 32.07031250108393294, 13.14518615778179189 ) ) ;
#648=EDGE_CURVE ( 'NONE', #24292, #15569, #2303, .T. ) ;
#649=CARTESIAN_POINT ( 'NONE',  ( 195.0000000000000000, 33.80664062608393294, 13.14518615778179544 ) ) ;
#652=CARTESIAN_POINT ( 'NONE',  ( -0.3969994146497772824, 51.45716825712459297, -15.00000000000033573 ) ) ;
#654=CARTESIAN_POINT ( 'NONE',  ( 65.00000000000000000, 36.00000000000000000, -7.517135062566165128E-15 ) ) ;
#656=( BOUNDED_CURVE ( )  B_SPLINE_CURVE ( 2, ( #15903, #27198, #9360, #11907, #14190, #4961, #20631, #9782, #7650 ),
 .UNSPECIFIED., .F., .T. ) 
 B_SPLINE_CURVE_WITH_KNOTS ( ( 3, 2, 2, 2, 3 ),
 ( 0.2708333333333330928, 0.2812499999999998890, 0.2916666666666666852, 0.3020833333333334259, 0.3125000000000002220 ),
 .UNSPECIFIED. ) 
 CURVE ( )  GEOMETRIC_REPRESENTATION_ITEM ( )  RATIONAL_B_SPLINE_CURVE ( ( 1.000000000000001554, 0.9238795325112850731, 1.000000000000000000, 0.9238795325112867385, 1.000000000000000000, 0.9238795325112867385, 1.000000000000000000, 0.9238795325112850731, 1.000000000000001554 ) ) 
 REPRESENTATION_ITEM ( '' )  );
#657=FACE_OUTER_BOUND ( 'NONE', #19869, .T. ) ;
#659=CARTESIAN_POINT ( 'NONE',  ( 208.1451861577818079, 40.35507812608393863, -1.609821015232357215E-15 ) ) ;
#663=EDGE_LOOP ( 'NONE', ( #12558, #2041, #9546, #25011 ) ) ;
#666=CARTESIAN_POINT ( 'NONE',  ( 138.3959387413077593, 54.99999999495823744, 14.99999999999996092 ) ) ;
#669=CARTESIAN_POINT ( 'NONE',  ( 78.14518615778179367, 33.21132812608393436, -1.609821015232357215E-15 ) ) ;
#672=CARTESIAN_POINT ( 'NONE',  ( -8.049105076161786076E-16, 37.97382812608393721, -13.14518615778179544 ) ) ;
#673=CIRCLE ( 'NONE', #4302, 5.000000000000000888 ) ;
#675=CARTESIAN_POINT ( 'NONE',  ( -3.863925265120440322, 54.10645156200380512, 14.99999999999999645 ) ) ;
#676=CARTESIAN_POINT ( 'NONE',  ( 135.6228728715778971, 40.45429687500001137, 13.57481594606306174 ) ) ;
#677=CARTESIAN_POINT ( 'NONE',  ( 143.5748159460630688, 37.42812499999999432, -1.662435489736055892E-15 ) ) ;
#683=CARTESIAN_POINT ( 'NONE',  ( 116.8548138422182063, 31.87187500108393223, 5.444914386472304635 ) ) ;
#684=CARTESIAN_POINT ( 'NONE',  ( 59.55508561352770158, 38.81718750108393579, -13.14518615778179900 ) ) ;
#686=CARTESIAN_POINT ( 'NONE',  ( -9.598844408820458085, 32.26875000216787726, -9.598844408820458085 ) ) ;
#691=CARTESIAN_POINT ( 'NONE',  ( 195.0000000000000000, 35.19570312608392726, 13.14518615778179544 ) ) ;
#692=DIRECTION ( 'NONE',  ( 0.000000000000000000, -1.000000000000000000, 0.000000000000000000 ) ) ;
#705=CARTESIAN_POINT ( 'NONE',  ( 70.44491438647230552, 32.86406250108392868, 13.14518615778179189 ) ) ;
#708=CARTESIAN_POINT ( 'NONE',  ( 195.0000000000000000, 36.93203125216787441, -13.57481594606304576 ) ) ;
#709=CARTESIAN_POINT ( 'NONE',  ( 13.57481594606304753, 32.71523437500000142, -5.622872871577873077 ) ) ;
#710=CARTESIAN_POINT ( 'NONE',  ( 116.8548138422182063, 36.73359375108393010, -5.444914386472297529 ) ) ;
#711=ORIENTED_EDGE ( 'NONE', *, *, #4617, .T. ) ;
#712=CARTESIAN_POINT ( 'NONE',  ( 97.92893218813451028, 80.18750000000000000, 4.999999999999989342 ) ) ;
#713=CIRCLE ( 'NONE', #17080, 5.000000000000004441 ) ;
#715=CARTESIAN_POINT ( 'NONE',  ( 104.4587341249999781, 84.00000000136560629, -1.846868145590750299 ) ) ;
#719=CARTESIAN_POINT ( 'NONE',  ( 55.70494972787295751, 32.11992187608393579, 9.295050272127047819 ) ) ;
#720=AXIS2_PLACEMENT_3D ( 'NONE', #7150, #15417, #19999 ) ;
#726=EDGE_LOOP ( 'NONE', ( #26515, #6676, #7045, #6065, #18961, #16121, #12170, #2779, #21665, #14808, #18012, #26164 ) ) ;
#728=CARTESIAN_POINT ( 'NONE',  ( 189.3771271284221314, 35.69179687716786731, 13.57481594606304753 ) ) ;
#731=CARTESIAN_POINT ( 'NONE',  ( 116.8548138422182205, 40.55351562608393579, 0.000000000000000000 ) ) ;
#732=CARTESIAN_POINT ( 'NONE',  ( 5.444914386472297529, 36.53515625108393294, -13.14518615778179900 ) ) ;
#736=DIRECTION ( 'NONE',  ( 0.000000000000000000, 0.000000000000000000, 1.000000000000000000 ) ) ;
#737=CARTESIAN_POINT ( 'NONE',  ( 117.6241215996508060, 35.99999999999999289, 4.513979326318619201 ) ) ;
#739=CARTESIAN_POINT ( 'NONE',  ( 208.0198548647683197, 36.00000000000000711, 3.369129432478914055 ) ) ;
#742=CARTESIAN_POINT ( 'NONE',  ( 0.000000000000000000, 50.00000000000000000, 0.000000000000000000 ) ) ;
#745=CYLINDRICAL_SURFACE ( 'NONE', #13433, 11.57481594606304398 ) ;
#746=CARTESIAN_POINT ( 'NONE',  ( -9.295050272127044266, 34.50117187608393721, 9.295050272127047819 ) ) ;
#747=VERTEX_POINT ( 'NONE', #25950 ) ;
#752=CARTESIAN_POINT ( 'NONE',  ( 208.1451861577817795, 35.34453125108392868, 5.444914386472293977 ) ) ;
#753=ORIENTED_EDGE ( 'NONE', *, *, #18439, .F. ) ;
#754=CARTESIAN_POINT ( 'NONE',  ( 193.4989808756949685, 53.60014735326986113, -15.00000000000000000 ) ) ;
#762=CARTESIAN_POINT ( 'NONE',  ( 120.7049497278729575, 37.27929687608393294, -9.295050272127046043 ) ) ;
#763=CARTESIAN_POINT ( 'NONE',  ( -5.444914386472299306, 37.72578125108394431, 13.14518615778179722 ) ) ;
#764=CARTESIAN_POINT ( 'NONE',  ( -9.295050272127044266, 34.30273437608393294, 9.295050272127047819 ) ) ;
#766=CARTESIAN_POINT ( 'NONE',  ( 57.37803646580599093, 54.91641323977226818, -14.99999999999999822 ) ) ;
#768=CARTESIAN_POINT ( 'NONE',  ( 208.5748159460630120, 39.85898437499999858, -5.622872871577873077 ) ) ;
#769=EDGE_CURVE ( 'NONE', #10253, #21981, #23538, .T. ) ;
#770=CARTESIAN_POINT ( 'NONE',  ( 69.85997726958113674, 35.99999999999999289, 12.29462155906316134 ) ) ;
#771=ORIENTED_EDGE ( 'NONE', *, *, #15560, .F. ) ;
#775=CARTESIAN_POINT ( 'NONE',  ( 65.00000000000000000, 38.76757812608393294, -13.14518615778179544 ) ) ;
#778=VERTEX_POINT ( 'NONE', #4290 ) ;
#780=EDGE_LOOP ( 'NONE', ( #22014, #25520, #18027, #26838 ) ) ;
#781=AXIS2_PLACEMENT_3D ( 'NONE', #19737, #5175, #18568 ) ;
#784=CARTESIAN_POINT ( 'NONE',  ( 204.2950502721270425, 37.08085937608393579, 9.295050272127046043 ) ) ;
#786=EDGE_LOOP ( 'NONE', ( #13335, #26038, #5279, #4137, #3777, #6140, #22751, #12521, #6165, #4758, #19712, #15028, #12709, #11189, #23225, #569, #24661 ) ) ;
#790=CARTESIAN_POINT ( 'NONE',  ( 135.4449143864723055, 32.26875000108393721, 13.14518615778179189 ) ) ;
#791=CARTESIAN_POINT ( 'NONE',  ( 55.70494972787295751, 40.65273437608393436, -9.295050272127046043 ) ) ;
#792=CARTESIAN_POINT ( 'NONE',  ( 189.5550856135277229, 34.25312500108393010, -13.14518615778179900 ) ) ;
#793=ADVANCED_FACE ( 'NONE', ( #6282, #1743 ), #6424, .F. ) ;
#795=ORIENTED_EDGE ( 'NONE', *, *, #15778, .F. ) ;
#799=CARTESIAN_POINT ( 'NONE',  ( 143.5748159460630404, 39.06523437716786873, 5.622872871577869525 ) ) ;
#801=CARTESIAN_POINT ( 'NONE',  ( -18.00000000000000711, 80.00000000000000000, -12.99999999999999645 ) ) ;
#804=FACE_OUTER_BOUND ( 'NONE', #18856, .T. ) ;
#805=ORIENTED_EDGE ( 'NONE', *, *, #10321, .T. ) ;
#808=EDGE_LOOP ( 'NONE', ( #10115, #14859, #2478, #8132 ) ) ;
#809=CARTESIAN_POINT ( 'NONE',  ( -13.15267690958718205, 36.00000000000000711, 0.5874252385153145850 ) ) ;
#811=CARTESIAN_POINT ( 'NONE',  ( 138.2014461876379983, 50.69246985422729779, 14.99999999999717382 ) ) ;
#812=ADVANCED_FACE ( 'NONE', ( #14959 ), #15093, .T. ) ;
#814=CARTESIAN_POINT ( 'NONE',  ( 185.4011555911795313, 40.20625000216787726, -9.598844408820458085 ) ) ;
#815=CARTESIAN_POINT ( 'NONE',  ( 70.44491438647230552, 32.56640625108394005, -13.14518615778179900 ) ) ;
#817=CARTESIAN_POINT ( 'NONE',  ( -5.622872871577947684, 39.36289062716787157, -13.57481594606297293 ) ) ;
#819=CARTESIAN_POINT ( 'NONE',  ( 55.81982418635200816, 50.00000000000000000, -10.00000000000000000 ) ) ;
#820=CARTESIAN_POINT ( 'NONE',  ( -4.925026783666235808, 49.99999999893053371, 12.67776588291678408 ) ) ;
#822=CARTESIAN_POINT ( 'NONE',  ( 143.5748159460630688, 35.84062499999999574, -1.662435489736055892E-15 ) ) ;
#826=DIRECTION ( 'NONE',  ( -1.156482317317871478E-16, 0.000000000000000000, -1.000000000000000000 ) ) ;
#830=CARTESIAN_POINT ( 'NONE',  ( 116.8548138422182063, 34.25312500108393010, 5.444914386472304635 ) ) ;
#832=CARTESIAN_POINT ( 'NONE',  ( 78.14518615778179367, 38.56914062608393579, -1.609821015232357215E-15 ) ) ;
#833=CARTESIAN_POINT ( 'NONE',  ( 2.414731522848535132E-15, 39.16445312608392726, 13.14518615778179544 ) ) ;
#834=CARTESIAN_POINT ( 'NONE',  ( -14.99999999999999822, 55.00000000000000000, 15.00000000000000000 ) ) ;
#838=CARTESIAN_POINT ( 'NONE',  ( 0.000000000000000000, 36.00000000000000000, 0.000000000000000000 ) ) ;
#842=CARTESIAN_POINT ( 'NONE',  ( 122.6059679576636796, 35.99999999999999289, -11.20317769887070547 ) ) ;
#853=CARTESIAN_POINT ( 'NONE',  ( 96.84719886470459471, 83.56250000136560629, 3.152801135295355994 ) ) ;
#854=CARTESIAN_POINT ( 'NONE',  ( 74.29505027212704249, 33.11210937608393579, -9.295050272127046043 ) ) ;
#860=CARTESIAN_POINT ( 'NONE',  ( 143.1451861577818079, 35.59257812608393579, -1.609821015232357215E-15 ) ) ;
#861=VERTEX_POINT ( 'NONE', #19534 ) ;
#864=CARTESIAN_POINT ( 'NONE',  ( 99.99999999999995737, 82.68750000136560629, 4.458734124999988779 ) ) ;
#866=CARTESIAN_POINT ( 'NONE',  ( 70.62287287157788285, 38.96601562716787015, 13.57481594606304576 ) ) ;
#869=CARTESIAN_POINT ( 'NONE',  ( 65.00000000000000000, 33.01289062608393721, 13.14518615778179544 ) ) ;
#871=CARTESIAN_POINT ( 'NONE',  ( -13.57481594606304576, 37.97382812716787726, 5.622872871577880183 ) ) ;
#872=ORIENTED_EDGE ( 'NONE', *, *, #6518, .F. ) ;
#873=CARTESIAN_POINT ( 'NONE',  ( 192.9130013513680808, 36.00000000000000711, -13.31420566034936392 ) ) ;
#877=CARTESIAN_POINT ( 'NONE',  ( 200.6228728715778686, 32.11992187716787583, -13.57481594606304753 ) ) ;
#879=DIRECTION ( 'NONE',  ( 0.000000000000000000, 0.000000000000000000, 1.000000000000000000 ) ) ;
#880=CARTESIAN_POINT ( 'NONE',  ( 135.4449143864723339, 40.30546875108393579, -13.14518615778179722 ) ) ;
#881=CARTESIAN_POINT ( 'NONE',  ( 13.14518615778179544, 35.59257812608393579, -1.609821015232357215E-15 ) ) ;
#883=CARTESIAN_POINT ( 'NONE',  ( 51.42518405393695957, 32.31835937499999289, 5.622872871577880183 ) ) ;
#888=CARTESIAN_POINT ( 'NONE',  ( 0.000000000000000000, 52.00000000000000711, 11.57481594606304398 ) ) ;
#893=FACE_OUTER_BOUND ( 'NONE', #12108, .T. ) ;
#894=DIRECTION ( 'NONE',  ( 0.000000000000000000, 1.000000000000000000, 0.000000000000000000 ) ) ;
#895=CARTESIAN_POINT ( 'NONE',  ( 13.14518615778179900, 33.95546875108393436, 5.444914386472293977 ) ) ;
#898=FACE_OUTER_BOUND ( 'NONE', #11315, .T. ) ;
#899=EDGE_CURVE ( 'NONE', #6096, #2435, #10963, .T. ) ;
#900=CARTESIAN_POINT ( 'NONE',  ( 185.7049497278729575, 35.89023437608393152, 9.295050272127047819 ) ) ;
#902=CARTESIAN_POINT ( 'NONE',  ( 195.8389268692911571, 53.50081894914646341, -15.00000000000000000 ) ) ;
#907=DIRECTION ( 'NONE',  ( 0.000000000000000000, 0.000000000000000000, 1.000000000000000000 ) ) ;
#910=CARTESIAN_POINT ( 'NONE',  ( 120.7049497278729575, 38.07304687608393579, -9.295050272127046043 ) ) ;
#911=CARTESIAN_POINT ( 'NONE',  ( -13.14518615778179189, 38.42031250108393436, 5.444914386472304635 ) ) ;
#912=CARTESIAN_POINT ( 'NONE',  ( 13.14518615778179544, 34.60039062608392868, -1.609821015232357215E-15 ) ) ;
#914=CARTESIAN_POINT ( 'NONE',  ( 73.77260924613699444, 50.37415326813934513, -15.00000000000000000 ) ) ;
#916=CARTESIAN_POINT ( 'NONE',  ( 130.0000000000000000, -7.395377635281828788, -13.57481594606305997 ) ) ;
#920=CARTESIAN_POINT ( 'NONE',  ( 78.14518615778179367, 38.56914062608393579, -1.609821015232357215E-15 ) ) ;
#921=CARTESIAN_POINT ( 'NONE',  ( 59.37712712842228058, 36.18789062716787441, -13.57481594606318254 ) ) ;
#922=LINE ( 'NONE', #9735, #12130 ) ;
#927=CARTESIAN_POINT ( 'NONE',  ( 195.0000000000000000, 39.36289062608393152, 13.14518615778179544 ) ) ;
#933=ORIENTED_EDGE ( 'NONE', *, *, #20510, .T. ) ;
#934=CARTESIAN_POINT ( 'NONE',  ( 124.5550856135277087, 33.45937500108394147, -13.14518615778179900 ) ) ;
#935=CARTESIAN_POINT ( 'NONE',  ( 59.55508561352770158, 40.60312500108393863, -13.14518615778179722 ) ) ;
#936=CARTESIAN_POINT ( 'NONE',  ( 208.1451861577817795, 34.74921875108395142, 5.444914386472293977 ) ) ;
#940=CARTESIAN_POINT ( 'NONE',  ( 121.2306103278992850, 50.37710889404841197, -14.99999999999737454 ) ) ;
#941=CARTESIAN_POINT ( 'NONE',  ( 120.4011555911795455, 36.43593750216787441, 9.598844408820459861 ) ) ;
#945=CARTESIAN_POINT ( 'NONE',  ( 65.87652626536205958, 51.45968077935079066, 15.00000000000066258 ) ) ;
#950=CARTESIAN_POINT ( 'NONE',  ( -4.459473413638155748, 36.00000000000000711, -12.68347323196786114 ) ) ;
#954=CARTESIAN_POINT ( 'NONE',  ( 51.85481384221819923, 33.55859375108393294, -5.444914386472297529 ) ) ;
#959=CARTESIAN_POINT ( 'NONE',  ( 13.57481594606304931, 40.55351562499999574, 5.622872871577868636 ) ) ;
#961=CARTESIAN_POINT ( 'NONE',  ( 3.979814445815163193, 50.00000000123243638, 13.01613927312660834 ) ) ;
#962=CARTESIAN_POINT ( 'NONE',  ( 116.4251840539369596, 35.49335937499999005, 5.622872871577880183 ) ) ;
#970=CARTESIAN_POINT ( 'NONE',  ( 139.2950502721270425, 34.50117187608393010, 9.295050272127046043 ) ) ;
#971=EDGE_CURVE ( 'NONE', #15569, #6096, #15953, .T. ) ;
#972=CARTESIAN_POINT ( 'NONE',  ( 74.59884440882045453, 32.07031250216787299, -9.598844408820458085 ) ) ;
#973=EDGE_CURVE ( 'NONE', #20261, #12084, #4861, .T. ) ;
#974=ORIENTED_EDGE ( 'NONE', *, *, #24272, .F. ) ;
#976=CARTESIAN_POINT ( 'NONE',  ( 2.414731522848535132E-15, 39.95820312608393010, 13.14518615778179544 ) ) ;
#978=CARTESIAN_POINT ( 'NONE',  ( 182.9434479702998146, 35.99999999999997868, 5.307619621752330374 ) ) ;
#981=CARTESIAN_POINT ( 'NONE',  ( 104.9999999999999716, 82.62500000273119838, -1.449011120738813565E-14 ) ) ;
#983=DIRECTION ( 'NONE',  ( -0.000000000000000000, 1.000000000000000000, -0.000000000000000000 ) ) ;
#985=CARTESIAN_POINT ( 'NONE',  ( 120.9219080773008557, 36.00000000000001421, -9.794392408848658249 ) ) ;
#987=CARTESIAN_POINT ( 'NONE',  ( 130.0000000000000000, 36.43593749999999432, 13.57481594606304576 ) ) ;
#996=CARTESIAN_POINT ( 'NONE',  ( 68.75563991928589758, 31.58960996655074993, -13.14518615778179544 ) ) ;
#999=CARTESIAN_POINT ( 'NONE',  ( 116.4251840539369596, 37.92421875216787441, 0.000000000000000000 ) ) ;
#1000=CARTESIAN_POINT ( 'NONE',  ( -13.57481594606304576, 33.90585937500000568, 5.622872871577880183 ) ) ;
#1002=CARTESIAN_POINT ( 'NONE',  ( 139.2950502721270425, 33.11210937608393579, 9.295050272127046043 ) ) ;
#1006=CARTESIAN_POINT ( 'NONE',  ( 78.57481594606305464, 38.37070312716787157, -5.622872871577873966 ) ) ;
#1007=CARTESIAN_POINT ( 'NONE',  ( 99.99999999999995737, 79.37500000273119838, 4.999999999999990230 ) ) ;
#1010=EDGE_CURVE ( 'NONE', #26975, #16918, #24120, .T. ) ;
#1012=CARTESIAN_POINT ( 'NONE',  ( 181.8548138422181921, 39.90859375108394147, -5.444914386472297529 ) ) ;
#1013=CARTESIAN_POINT ( 'NONE',  ( -5.622872871577873077, 39.66054687716786731, 13.57481594606304753 ) ) ;
#1016=EDGE_CURVE ( 'NONE', #2438, #16078, #2443, .T. ) ;
#1018=ORIENTED_EDGE ( 'NONE', *, *, #19485, .F. ) ;
#1020=CARTESIAN_POINT ( 'NONE',  ( 208.1451861577817795, 40.10703125108393152, 5.444914386472293977 ) ) ;
#1025=CARTESIAN_POINT ( 'NONE',  ( 116.8548138422182063, 31.77265625108393365, -5.444914386472297529 ) ) ;
#1031=CARTESIAN_POINT ( 'NONE',  ( 65.00000000000000000, 40.35507812608393152, -13.14518615778179544 ) ) ;
#1037=CARTESIAN_POINT ( 'NONE',  ( 5.444914386472297529, 33.36015625108393579, -13.14518615778179900 ) ) ;
#1039=FACE_OUTER_BOUND ( 'NONE', #4312, .T. ) ;
#1040=CARTESIAN_POINT ( 'NONE',  ( -8.312177448680279460E-16, 36.03906250000000000, -13.57481594606304576 ) ) ;
#1041=EDGE_CURVE ( 'NONE', #19008, #5192, #8486, .T. ) ;
#1042=CARTESIAN_POINT ( 'NONE',  ( 208.1451861577817795, 36.13828125108393863, 5.444914386472293977 ) ) ;
#1044=CARTESIAN_POINT ( 'NONE',  ( 191.1969456267529779, 54.09082899096177499, -15.00000000000000000 ) ) ;
#1049=CARTESIAN_POINT ( 'NONE',  ( 189.3771271284221314, 40.15664062716787441, -13.57481594606304753 ) ) ;
#1050=DIRECTION ( 'NONE',  ( -0.000000000000000000, 1.000000000000000000, -0.000000000000000000 ) ) ;
#1051=CARTESIAN_POINT ( 'NONE',  ( 135.4449143864723055, 38.42031250108393436, 13.14518615778179189 ) ) ;
#1052=CARTESIAN_POINT ( 'NONE',  ( -13.14518615778179722, 38.32109375108394289, -5.444914386472297529 ) ) ;
#1053=CARTESIAN_POINT ( 'NONE',  ( 13.14518615778179900, 33.06250000108393294, -5.444914386472297529 ) ) ;
#1058=EDGE_LOOP ( 'NONE', ( #11036, #3352, #21158, #7142 ) ) ;
#1062=CARTESIAN_POINT ( 'NONE',  ( 78.14518615778180788, 36.23750000108393010, -5.444914386472297529 ) ) ;
#1063=DIRECTION ( 'NONE',  ( 0.000000000000000000, 1.000000000000000000, 0.000000000000000000 ) ) ;
#1064=CARTESIAN_POINT ( 'NONE',  ( 51.42518405393695957, 38.61874999999999147, 0.000000000000000000 ) ) ;
#1065=CARTESIAN_POINT ( 'NONE',  ( 204.2950502721270425, 37.08085937608393579, -9.295050272127046043 ) ) ;
#1070=CARTESIAN_POINT ( 'NONE',  ( 181.8548138422182205, 36.78320312608393294, 0.000000000000000000 ) ) ;
#1074=VERTEX_POINT ( 'NONE', #26671 ) ;
#1076=CARTESIAN_POINT ( 'NONE',  ( 59.55508561352770158, 39.80937500108393579, -13.14518615778179722 ) ) ;
#1079=CARTESIAN_POINT ( 'NONE',  ( 189.5550856135277229, 35.04687500108393294, -13.14518615778179900 ) ) ;
#1080=VERTEX_POINT ( 'NONE', #2586 ) ;
#1083=DIRECTION ( 'NONE',  ( -0.000000000000000000, 0.000000000000000000, -1.000000000000000000 ) ) ;
#1084=CARTESIAN_POINT ( 'NONE',  ( 120.4011555911795455, 37.22968750216787726, 9.598844408820459861 ) ) ;
#1085=( BOUNDED_SURFACE ( )  B_SPLINE_SURFACE ( 1, 2, ( 
 ( #6719, #2182, #19557, #17555, #23979, #15404, #4457, #14983, #25832, #13112, #6445, #17414, #21984, #23837, #17129, #24119, #10709, #21850, #10573, #4039, #12703, #6306, #4316, #4593, #19838, #19282, #23700, #23561, #17271, #8441, #10843, #325, #27981, #21428, #4176, #9010, #19695, #28117, #12838, #26260, #8863, #2326, #21565, #26404, #15260, #6862, #181, #13253, #1907, #2040, #8582, #8722, #39, #11123, #19415, #2462, #17702, #25974, #15116, #12973, #21707, #26112, #6578, #10982, #5166, #2606, #13829, #466, #4886, #11268, #26981, #13693, #3166, #22127, #20266, #20414, #26837, #5027, #7426, #7285, #15975, #16119, #24689, #19988, #22409, #18416, #22554, #15549, #9149, #1042, #11691, #20128, #17843, #18275, #900, #3021, #13549, #27122, #9570, #24258, #24825, #5310, #4740, #26546, #609, #752, #9424, #11838, #22273, #13971, #22699, #9285, #7140, #13400, #2878, #18124, #7001, #20561, #9715, #15695, #24398, #2747, #11410, #17981, #26690, #11550, #15835, #24543, #25106, #20839, #5594, #27262, #9985, #14260, #22980, #18694, #3447, #5450, #7718, #25243, #12112, #27397, #7857, #14117, #9851, #7571, #16268, #1316, #22841, #16551, #24966, #3308, #18557, #11979, #20703, #1185, #16410, #6209, #18384, #17023, #27739, #11807, #3935, #22951, #25078, #1155, #22810, #10608, #25588, #7540, #19315, #16889, #21461, #8199, #27876, #4075, #3278, #7686, #27089, #14878, #16238, #25726, #12454 ),
 ( #24935, #23458, #16378, #6072, #12737, #5566, #5422, #23593, #20671, #12594, #20530, #13941, #22667, #14091, #14229, #1939, #28016, #1012, #11947, #5275, #27232, #9820, #21179, #8482, #9681, #18527, #21319, #3413, #1660, #10320, #19027, #17171, #14738, #1801, #3139, #10466, #19174, #8338, #19875, #24295, #23873, #77, #10744, #26441, #8620, #9048, #4494, #21890, #361, #26298, #17740, #6759, #17308, #28154, #15443, #8759, #19731, #4776, #26149, #19456, #6901, #13006, #24158, #12869, #6341, #15015, #26008, #6616, #15589, #22164, #21599, #6480, #25872, #19594, #15154, #13152, #2642, #2076, #23737, #4352, #11304, #22021, #2222, #21746, #13437, #11160, #4635, #10886, #505, #17591, #9186, #2498, #20026, #4211, #17450, #15300, #11019, #2363, #24016, #216, #8903, #13293, #22449, #9462, #17880, #16011, #22595, #2782, #18457, #7464, #4923, #16159, #11446, #7174, #13586, #1079, #24725, #5486, #24436, #3064, #22736, #936, #7322, #9747, #9607, #18310, #27163, #27018, #22308, #5204, #20736, #792, #26586, #3202, #25009, #5347, #18165, #24866, #2916, #20167, #649, #14013, #11872, #20595, #13868, #20307, #7034, #7615, #11728, #16308, #9322, #14156, #20454, #22876, #3343, #12012, #1221, #15871, #26877, #18018, #15732, #26729, #24581, #5063, #13727, #11587, #10291, #21287, #18998, #1358, #12147, #27708, #21013, #3766, #8304, #10147, #3483, #1771, #25278, #8171, #25139, #18594, #27299 ) ),
 .UNSPECIFIED., .F., .F., .T. ) 
 B_SPLINE_SURFACE_WITH_KNOTS ( ( 2, 2 ),
 ( 3, 2, 2, 2, 2, 2, 2, 2, 2, 2, 2, 2, 2, 2, 2, 2, 2, 2, 2, 2, 2, 2, 2, 2, 2, 2, 2, 2, 2, 2, 2, 2, 2, 2, 2, 2, 2, 2, 2, 2, 2, 2, 2, 2, 2, 2, 2, 2, 2, 2, 2, 2, 2, 2, 2, 2, 2, 2, 2, 2, 2, 2, 2, 2, 2, 2, 2, 2, 2, 2, 2, 2, 2, 2, 2, 2, 2, 2, 2, 2, 2, 2, 2, 2, 2, 2, 2, 2, 2, 2, 2, 3 ),
 ( 0.000000000000000000, 1.000000000000000000 ),
 ( 0.000000000000000000, 0.01041666666666666609, 0.02083333333333333218, 0.03125000000000000000, 0.04166666666666666435, 0.05208333333333333565, 0.06250000000000000000, 0.07291666666666667129, 0.08333333333333332871, 0.09375000000000000000, 0.1041666666666666713, 0.1145833333333333287, 0.1250000000000000000, 0.1354166666666666574, 0.1458333333333333426, 0.1562500000000000000, 0.1666666666666666574, 0.1770833333333333426, 0.1875000000000000000, 0.1979166666666666574, 0.2083333333333333426, 0.2187500000000000000, 0.2291666666666666574, 0.2395833333333333426, 0.2500000000000000000, 0.2604166666666666852, 0.2708333333333333148, 0.2812500000000000000, 0.2916666666666666852, 0.3020833333333333148, 0.3125000000000000000, 0.3229166666666666852, 0.3333333333333333148, 0.3437500000000000000, 0.3541666666666666852, 0.3645833333333333148, 0.3750000000000000000, 0.3854166666666666852, 0.3958333333333333148, 0.4062500000000000000, 0.4166666666666666852, 0.4270833333333333148, 0.4375000000000000000, 0.4479166666666666852, 0.4583333333333333148, 0.4687500000000000000, 0.4791666666666666852, 0.4895833333333333148, 0.5000000000000000000, 0.5104166666666666297, 0.5208333333333333703, 0.5312500000000000000, 0.5416666666666666297, 0.5520833333333333703, 0.5625000000000000000, 0.5729166666666666297, 0.5833333333333333703, 0.5937500000000000000, 0.6041666666666666297, 0.6145833333333333703, 0.6250000000000000000, 0.6354166666666666297, 0.6458333333333333703, 0.6562500000000000000, 0.6666666666666666297, 0.6770833333333333703, 0.6875000000000000000, 0.6979166666666666297, 0.7083333333333333703, 0.7187500000000000000, 0.7291666666666666297, 0.7395833333333333703, 0.7500000000000000000, 0.7604166666666666297, 0.7708333333333333703, 0.7812500000000000000, 0.7916666666666666297, 0.8020833333333333703, 0.8125000000000000000, 0.8229166666666666297, 0.8333333333333333703, 0.8437500000000000000, 0.8541666666666666297, 0.8645833333333333703, 0.8750000000000000000, 0.8854166666666666297, 0.8958333333333333703, 0.9062500000000000000, 0.9166666666666666297, 0.9270833333333333703, 0.9375000000000000000, 0.9448587001587775980 ),
 .UNSPECIFIED. ) 
 GEOMETRIC_REPRESENTATION_ITEM ( )  RATIONAL_B_SPLINE_SURFACE ( (
 ( 1.000000000000000000, 0.9238795325112867385, 1.000000000000000000, 0.9238795325112867385, 1.000000000000000000, 0.9238795325112867385, 1.000000000000000000, 0.9238795325112867385, 1.000000000000000000, 0.9238795325112867385, 1.000000000000000000, 0.9238795325112867385, 1.000000000000000000, 0.9238795325112867385, 1.000000000000000000, 0.9238795325112867385, 1.000000000000000000, 0.9238795325112867385, 1.000000000000000000, 0.9238795325112867385, 1.000000000000000000, 0.9238795325112867385, 1.000000000000000000, 0.9238795325112867385, 1.000000000000000000, 0.9238795325112867385, 1.000000000000000000, 0.9238795325112867385, 1.000000000000000000, 0.9238795325112867385, 1.000000000000000000, 0.9238795325112867385, 1.000000000000000000, 0.9238795325112867385, 1.000000000000000000, 0.9238795325112867385, 1.000000000000000000, 0.9238795325112867385, 1.000000000000000000, 0.9238795325112867385, 1.000000000000000000, 0.9238795325112867385, 1.000000000000000000, 0.9238795325112867385, 1.000000000000000000, 0.9238795325112867385, 1.000000000000000000, 0.9238795325112867385, 1.000000000000000000, 0.9238795325112867385, 1.000000000000000000, 0.9238795325112867385, 1.000000000000000000, 0.9238795325112867385, 1.000000000000000000, 0.9238795325112867385, 1.000000000000000000, 0.9238795325112867385, 1.000000000000000000, 0.9238795325112867385, 1.000000000000000000, 0.9238795325112867385, 1.000000000000000000, 0.9238795325112867385, 1.000000000000000000, 0.9238795325112867385, 1.000000000000000000, 0.9238795325112867385, 1.000000000000000000, 0.9238795325112867385, 1.000000000000000000, 0.9238795325112867385, 1.000000000000000000, 0.9238795325112867385, 1.000000000000000000, 0.9238795325112867385, 1.000000000000000000, 0.9238795325112867385, 1.000000000000000000, 0.9238795325112867385, 1.000000000000000000, 0.9238795325112867385, 1.000000000000000000, 0.9238795325112867385, 1.000000000000000000, 0.9238795325112867385, 1.000000000000000000, 0.9238795325112867385, 1.000000000000000000, 0.9238795325112867385, 1.000000000000000000, 0.9238795325112867385, 1.000000000000000000, 0.9238795325112867385, 1.000000000000000000, 0.9238795325112867385, 1.000000000000000000, 0.9238795325112867385, 1.000000000000000000, 0.9238795325112867385, 1.000000000000000000, 0.9238795325112867385, 1.000000000000000000, 0.9238795325112867385, 1.000000000000000000, 0.9238795325112867385, 1.000000000000000000, 0.9238795325112867385, 1.000000000000000000, 0.9238795325112867385, 1.000000000000000000, 0.9238795325112867385, 1.000000000000000000, 0.9238795325112867385, 1.000000000000000000, 0.9238795325112867385, 1.000000000000000000, 0.9238795325112867385, 1.000000000000000000, 0.9238795325112867385, 1.000000000000000000, 0.9238795325112867385, 1.000000000000000000, 0.9238795325112867385, 1.000000000000000000, 0.9238795325112867385, 1.000000000000000000, 0.9238795325112867385, 1.000000000000000000, 0.9238795325112867385, 1.000000000000000000, 0.9238795325112867385, 1.000000000000000000, 0.9238795325112867385, 1.000000000000000000, 0.9238795325112867385, 1.000000000000000000, 0.9238795325112867385, 1.000000000000000000, 0.9238795325112867385, 1.000000000000000000, 0.9238795325112867385, 1.000000000000000000, 0.9238795325112867385, 1.000000000000000000, 0.9238795325112867385, 1.000000000000000000, 0.9238795325112867385, 1.000000000000000000, 0.9238795325112867385, 1.000000000000000000, 0.9238795325112867385, 1.000000000000000000, 0.9238795325112867385, 1.000000000000000000, 0.9238795325112867385, 1.000000000000000000, 0.9238795325112867385, 1.000000000000000000, 0.9238795325112867385, 1.000000000000000000, 0.9238795325112867385, 1.000000000000000000, 0.9238795325112867385, 1.000000000000000000, 0.9238795325112867385, 1.000000000000000000, 0.9238795325112867385, 1.000000000000000000, 0.9238795325112867385, 1.000000000000000000, 0.9238795325112867385, 1.000000000000000000, 0.9238795325112867385, 1.000000000000000000, 0.9238795325112867385, 1.000000000000000000, 0.9238795325112867385, 1.000000000000000000, 0.9238795325112867385, 1.000000000000000000, 0.9462258211652395667, 0.9684275895297407288),
 ( 1.000000000000000000, 0.9238795325112867385, 1.000000000000000000, 0.9238795325112867385, 1.000000000000000000, 0.9238795325112867385, 1.000000000000000000, 0.9238795325112867385, 1.000000000000000000, 0.9238795325112867385, 1.000000000000000000, 0.9238795325112867385, 1.000000000000000000, 0.9238795325112867385, 1.000000000000000000, 0.9238795325112867385, 1.000000000000000000, 0.9238795325112867385, 1.000000000000000000, 0.9238795325112867385, 1.000000000000000000, 0.9238795325112867385, 1.000000000000000000, 0.9238795325112867385, 1.000000000000000000, 0.9238795325112867385, 1.000000000000000000, 0.9238795325112867385, 1.000000000000000000, 0.9238795325112867385, 1.000000000000000000, 0.9238795325112867385, 1.000000000000000000, 0.9238795325112867385, 1.000000000000000000, 0.9238795325112867385, 1.000000000000000000, 0.9238795325112867385, 1.000000000000000000, 0.9238795325112867385, 1.000000000000000000, 0.9238795325112867385, 1.000000000000000000, 0.9238795325112867385, 1.000000000000000000, 0.9238795325112867385, 1.000000000000000000, 0.9238795325112867385, 1.000000000000000000, 0.9238795325112867385, 1.000000000000000000, 0.9238795325112867385, 1.000000000000000000, 0.9238795325112867385, 1.000000000000000000, 0.9238795325112867385, 1.000000000000000000, 0.9238795325112867385, 1.000000000000000000, 0.9238795325112867385, 1.000000000000000000, 0.9238795325112867385, 1.000000000000000000, 0.9238795325112867385, 1.000000000000000000, 0.9238795325112867385, 1.000000000000000000, 0.9238795325112867385, 1.000000000000000000, 0.9238795325112867385, 1.000000000000000000, 0.9238795325112867385, 1.000000000000000000, 0.9238795325112867385, 1.000000000000000000, 0.9238795325112867385, 1.000000000000000000, 0.9238795325112867385, 1.000000000000000000, 0.9238795325112867385, 1.000000000000000000, 0.9238795325112867385, 1.000000000000000000, 0.9238795325112867385, 1.000000000000000000, 0.9238795325112867385, 1.000000000000000000, 0.9238795325112867385, 1.000000000000000000, 0.9238795325112867385, 1.000000000000000000, 0.9238795325112867385, 1.000000000000000000, 0.9238795325112867385, 1.000000000000000000, 0.9238795325112867385, 1.000000000000000000, 0.9238795325112867385, 1.000000000000000000, 0.9238795325112867385, 1.000000000000000000, 0.9238795325112867385, 1.000000000000000000, 0.9238795325112867385, 1.000000000000000000, 0.9238795325112867385, 1.000000000000000000, 0.9238795325112867385, 1.000000000000000000, 0.9238795325112867385, 1.000000000000000000, 0.9238795325112867385, 1.000000000000000000, 0.9238795325112867385, 1.000000000000000000, 0.9238795325112867385, 1.000000000000000000, 0.9238795325112867385, 1.000000000000000000, 0.9238795325112867385, 1.000000000000000000, 0.9238795325112867385, 1.000000000000000000, 0.9238795325112867385, 1.000000000000000000, 0.9238795325112867385, 1.000000000000000000, 0.9238795325112867385, 1.000000000000000000, 0.9238795325112867385, 1.000000000000000000, 0.9238795325112867385, 1.000000000000000000, 0.9238795325112867385, 1.000000000000000000, 0.9238795325112867385, 1.000000000000000000, 0.9238795325112867385, 1.000000000000000000, 0.9238795325112867385, 1.000000000000000000, 0.9238795325112867385, 1.000000000000000000, 0.9238795325112867385, 1.000000000000000000, 0.9238795325112867385, 1.000000000000000000, 0.9238795325112867385, 1.000000000000000000, 0.9238795325112867385, 1.000000000000000000, 0.9238795325112867385, 1.000000000000000000, 0.9238795325112867385, 1.000000000000000000, 0.9238795325112867385, 1.000000000000000000, 0.9238795325112867385, 1.000000000000000000, 0.9238795325112867385, 1.000000000000000000, 0.9238795325112867385, 1.000000000000000000, 0.9238795325112867385, 1.000000000000000000, 0.9238795325112867385, 1.000000000000000000, 0.9238795325112867385, 1.000000000000000000, 0.9238795325112867385, 1.000000000000000000, 0.9238795325112867385, 1.000000000000000000, 0.9238795325112867385, 1.000000000000000000, 0.9238795325112867385, 1.000000000000000000, 0.9238795325112867385, 1.000000000000000000, 0.9238795325112867385, 1.000000000000000000, 0.9462258211652395667, 0.9684275895297407288) ) ) 
 REPRESENTATION_ITEM ( '' )  SURFACE ( )  );
#1086=CARTESIAN_POINT ( 'NONE',  ( 51.42518405393695957, 40.30546875216787583, 0.000000000000000000 ) ) ;
#1088=CARTESIAN_POINT ( 'NONE',  ( 66.89218335708966379, 53.66387243067953960, 14.99999999999997868 ) ) ;
#1089=VERTEX_POINT ( 'NONE', #18103 ) ;
#1090=EDGE_CURVE ( 'NONE', #17873, #18589, #5904, .T. ) ;
#1095=CARTESIAN_POINT ( 'NONE',  ( 132.2761468445512776, 51.46995505939284499, 15.00000000000097700 ) ) ;
#1096=CARTESIAN_POINT ( 'NONE',  ( -6.338290792350127489, 36.00000000000002132, 11.53992004314986453 ) ) ;
#1097=CARTESIAN_POINT ( 'NONE',  ( 65.00000000000000000, 33.01289062608393721, 13.14518615778179544 ) ) ;
#1098=CIRCLE ( 'NONE', #168, 5.000000000000000888 ) ;
#1099=CARTESIAN_POINT ( 'NONE',  ( -9.598844408820458085, 40.20625000216787726, -9.598844408820458085 ) ) ;
#1100=CARTESIAN_POINT ( 'NONE',  ( 189.3771271284220177, 37.97382812499999716, 13.57481594606295161 ) ) ;
#1101=CARTESIAN_POINT ( 'NONE',  ( 94.99999999999995737, 80.93750000000001421, -2.071067811865491493 ) ) ;
#1102=CARTESIAN_POINT ( 'NONE',  ( 99.99999999999995737, 80.00000000000000000, 4.999999999999990230 ) ) ;
#1103=CARTESIAN_POINT ( 'NONE',  ( -3.716534113788169336, 51.46663580899896573, 15.00000000000068212 ) ) ;
#1105=CARTESIAN_POINT ( 'NONE',  ( 143.5748159460630404, 35.89023437499999858, -5.622872871577873077 ) ) ;
#1106=ORIENTED_EDGE ( 'NONE', *, *, #23640, .F. ) ;
#1108=FACE_OUTER_BOUND ( 'NONE', #23717, .T. ) ;
#1112=CARTESIAN_POINT ( 'NONE',  ( 130.0000000000000000, 34.40195312608393152, 13.14518615778179544 ) ) ;
#1113=CARTESIAN_POINT ( 'NONE',  ( 65.00000000000000000, 38.76757812608393294, -13.14518615778179544 ) ) ;
#1115=CARTESIAN_POINT ( 'NONE',  ( -13.14518615778179544, 38.96601562608393721, 0.000000000000000000 ) ) ;
#1117=CARTESIAN_POINT ( 'NONE',  ( 182.6241215996508629, 36.00000000000000711, 4.513979326318628971 ) ) ;
#1122=CARTESIAN_POINT ( 'NONE',  ( 134.8599772695820889, 36.00000000000000000, 12.29462155906280252 ) ) ;
#1125=CARTESIAN_POINT ( 'NONE',  ( 120.1606183911117114, 36.00000000000001421, -9.004033604612676100 ) ) ;
#1126=CARTESIAN_POINT ( 'NONE',  ( 99.99999999999995737, 85.00000000000000000, -1.387778780781445676E-14 ) ) ;
#1136=LINE ( 'NONE', #16219, #13292 ) ;
#1137=CARTESIAN_POINT ( 'NONE',  ( 74.29505027212704249, 32.91367187608393152, 9.295050272127046043 ) ) ;
#1143=CARTESIAN_POINT ( 'NONE',  ( -8.312177448680279460E-16, 33.65781249999999147, -13.57481594606304576 ) ) ;
#1145=CARTESIAN_POINT ( 'NONE',  ( 116.8548138422182063, 35.93984375108393436, -5.444914386472297529 ) ) ;
#1147=CARTESIAN_POINT ( 'NONE',  ( 96.46446609406721961, 82.12500000000000000, 3.535533905932727539 ) ) ;
#1149=CARTESIAN_POINT ( 'NONE',  ( 98.15313185440925281, 83.62500000136560629, 4.458734124999987891 ) ) ;
#1151=CARTESIAN_POINT ( 'NONE',  ( 124.3771271284220319, 38.46992187499999005, -13.57481594606295339 ) ) ;
#1153=CIRCLE ( 'NONE', #25254, 13.57481594606304398 ) ;
#1155=CARTESIAN_POINT ( 'NONE',  ( 200.4449143864723055, 32.36796875108393579, -13.14518615778179900 ) ) ;
#1156=CARTESIAN_POINT ( 'NONE',  ( 9.598844408820459861, 39.80937500216786873, 9.598844408820456309 ) ) ;
#1159=ORIENTED_EDGE ( 'NONE', *, *, #479, .F. ) ;
#1161=CARTESIAN_POINT ( 'NONE',  ( 208.5748159460630688, 32.76484375216787015, -1.662435489736055892E-15 ) ) ;
#1166=CARTESIAN_POINT ( 'NONE',  ( 219.9999999999999716, 50.00000000000000000, -10.00000000000000000 ) ) ;
#1177=CARTESIAN_POINT ( 'NONE',  ( 208.5748159460630688, 39.80937499999999574, -1.662435489736055892E-15 ) ) ;
#1179=CARTESIAN_POINT ( 'NONE',  ( -13.14518615778179900, 33.55859375108393294, -5.444914386472297529 ) ) ;
#1182=DIRECTION ( 'NONE',  ( -0.000000000000000000, 1.000000000000000000, -0.000000000000000000 ) ) ;
#1184=EDGE_CURVE ( 'NONE', #21487, #8092, #26713, .T. ) ;
#1185=CARTESIAN_POINT ( 'NONE',  ( 200.4449143864723055, 32.86406250108392868, 13.14518615778179189 ) ) ;
#1186=ORIENTED_EDGE ( 'NONE', *, *, #27057, .T. ) ;
#1187=CARTESIAN_POINT ( 'NONE',  ( -9.598844408820454532, 37.13046874999999147, 9.598844408820459861 ) ) ;
#1193=FACE_OUTER_BOUND ( 'NONE', #18306, .T. ) ;
#1194=CARTESIAN_POINT ( 'NONE',  ( 143.1451861577818079, 36.93203125108394147, 5.444914386472293977 ) ) ;
#1195=CARTESIAN_POINT ( 'NONE',  ( -9.295050272127044266, 36.88242187608393152, 9.295050272127047819 ) ) ;
#1196=CARTESIAN_POINT ( 'NONE',  ( 5.444914386472302859, 33.65781250108393152, 13.14518615778179189 ) ) ;
#1198=CIRCLE ( 'NONE', #17089, 5.000000000000000000 ) ;
#1200=CARTESIAN_POINT ( 'NONE',  ( -9.598844408820454532, 37.22968750216787726, 9.598844408820459861 ) ) ;
#1203=CARTESIAN_POINT ( 'NONE',  ( 95.54126587499996504, 84.62500000136560629, -1.846868145590750077 ) ) ;
#1205=ADVANCED_FACE ( 'NONE', ( #5406 ), #3396, .T. ) ;
#1206=CARTESIAN_POINT ( 'NONE',  ( 195.0000000000000000, 38.81718749999999574, 13.57481594606304576 ) ) ;
#1207=DIRECTION ( 'NONE',  ( 0.000000000000000000, -1.000000000000000000, 0.000000000000000000 ) ) ;
#1218=CARTESIAN_POINT ( 'NONE',  ( 130.0000000000000000, 38.81718749999999574, 13.57481594606304576 ) ) ;
#1221=CARTESIAN_POINT ( 'NONE',  ( 195.0000000000000000, 33.01289062608393721, 13.14518615778179544 ) ) ;
#1222=EDGE_LOOP ( 'NONE', ( #15278, #5218, #11333, #3911 ) ) ;
#1223=DIRECTION ( 'NONE',  ( 0.000000000000000000, 0.000000000000000000, -1.000000000000000000 ) ) ;
#1224=CARTESIAN_POINT ( 'NONE',  ( 9.180175813647991845, 50.00000000000000711, -15.00000000000000000 ) ) ;
#1226=CARTESIAN_POINT ( 'NONE',  ( 124.3771271284221314, 36.48554687716787015, 13.57481594606304753 ) ) ;
#1228=DIRECTION ( 'NONE',  ( 0.000000000000000000, 1.000000000000000000, 0.000000000000000000 ) ) ;
#1229=DIRECTION ( 'NONE',  ( 6.938893903907232322E-16, -1.000000000000000000, 0.000000000000000000 ) ) ;
#1230=CARTESIAN_POINT ( 'NONE',  ( 195.0000000000000000, 36.98164062608393721, 13.14518615778179544 ) ) ;
#1234=CARTESIAN_POINT ( 'NONE',  ( -7.394032042335738630, 36.00000000000004263, -11.20317769887113180 ) ) ;
#1235=CARTESIAN_POINT ( 'NONE',  ( 95.54126587499996504, 84.43750000136560629, -1.387778780781445676E-14 ) ) ;
#1236=CARTESIAN_POINT ( 'NONE',  ( 59.55508561352770158, 32.66562500108393863, -13.14518615778179900 ) ) ;
#1237=( NAMED_UNIT ( * ) PLANE_ANGLE_UNIT ( ) SI_UNIT ( $, .RADIAN. ) );
#1240=CARTESIAN_POINT ( 'NONE',  ( 2.232327155337096691, 35.99999999999998579, 12.98409812936892926 ) ) ;
#1241=DIRECTION ( 'NONE',  ( -0.000000000000000000, 1.000000000000000000, 0.000000000000000000 ) ) ;
#1242=CARTESIAN_POINT ( 'NONE',  ( 135.6228728715778971, 34.89804687499999147, 13.57481594606304576 ) ) ;
#1244=CARTESIAN_POINT ( 'NONE',  ( 195.0000000000000000, 38.12265625216787157, 13.57481594606304576 ) ) ;
#1247=( BOUNDED_CURVE ( )  B_SPLINE_CURVE ( 2, ( #18921, #23073, #10495, #20933, #21351, #16784, #5961, #3965, #10350 ),
 .UNSPECIFIED., .F., .F. ) 
 B_SPLINE_CURVE_WITH_KNOTS ( ( 3, 2, 2, 2, 3 ),
 ( 0.1458333333333336757, 0.1562500000000002776, 0.1666666666666669072, 0.1770833333333335369, 0.1875000000000001388 ),
 .UNSPECIFIED. ) 
 CURVE ( )  GEOMETRIC_REPRESENTATION_ITEM ( )  RATIONAL_B_SPLINE_CURVE ( ( 0.9999999999999975575, 0.9238795325112891810, 1.000000000000000000, 0.9238795325112867385, 1.000000000000000000, 0.9238795325112867385, 1.000000000000000000, 0.9238795325112857393, 1.000000000000001110 ) ) 
 REPRESENTATION_ITEM ( '' )  );
#1249=CARTESIAN_POINT ( 'NONE',  ( 124.5550856135277087, 40.60312500108393863, -13.14518615778179900 ) ) ;
#1250=CARTESIAN_POINT ( 'NONE',  ( 59.55508561352770158, 39.90859375108393436, 13.14518615778179722 ) ) ;
#1253=CARTESIAN_POINT ( 'NONE',  ( -9.295050272127046043, 39.66054687608393436, -9.295050272127046043 ) ) ;
#1255=DIRECTION ( 'NONE',  ( 0.000000000000000000, -1.000000000000000000, 0.000000000000000000 ) ) ;
#1257=CARTESIAN_POINT ( 'NONE',  ( 207.0772764098356049, 36.00000000000000000, -6.197985357349214297 ) ) ;
#1258=CARTESIAN_POINT ( 'NONE',  ( 181.8548138422181921, 32.66562500108393863, 5.444914386472304635 ) ) ;
#1261=CARTESIAN_POINT ( 'NONE',  ( 117.1404900439224974, 36.00000000000000000, -3.245221471866906349 ) ) ;
#1262=DIRECTION ( 'NONE',  ( 0.000000000000000000, 0.000000000000000000, -1.000000000000000000 ) ) ;
#1268=CARTESIAN_POINT ( 'NONE',  ( 189.3771271284221314, 32.11992187499999574, -13.57481594606304753 ) ) ;
#1271=CARTESIAN_POINT ( 'NONE',  ( 99.99999999999995737, 82.68750000136560629, 4.458734124999988779 ) ) ;
#1272=CARTESIAN_POINT ( 'NONE',  ( 65.00000000000000000, 32.02070312608393010, 13.14518615778179544 ) ) ;
#1276=CARTESIAN_POINT ( 'NONE',  ( 9.598844408820456309, 34.35234374999999574, -9.598844408820458085 ) ) ;
#1278=CARTESIAN_POINT ( 'NONE',  ( 124.5550856135277087, 33.75703125108393721, 13.14518615778179722 ) ) ;
#1279=ORIENTED_EDGE ( 'NONE', *, *, #27941, .T. ) ;
#1280=CARTESIAN_POINT ( 'NONE',  ( -3.039397050802532529, 53.88964894337312472, -15.00000000000000533 ) ) ;
#1282=CARTESIAN_POINT ( 'NONE',  ( 104.9999999999999574, 79.56250000273121259, 2.071067811865462627 ) ) ;
#1283=CARTESIAN_POINT ( 'NONE',  ( 120.7049497278729575, 39.66054687608393436, -9.295050272127046043 ) ) ;
#1286=CARTESIAN_POINT ( 'NONE',  ( 9.598844408820459861, 38.22187500216787015, 9.598844408820456309 ) ) ;
#1291=CARTESIAN_POINT ( 'NONE',  ( 181.8548138422181921, 39.80937500108392868, 5.444914386472304635 ) ) ;
#1294=CARTESIAN_POINT ( 'NONE',  ( 116.8548138422182205, 39.75976562608393294, 0.000000000000000000 ) ) ;
#1295=CARTESIAN_POINT ( 'NONE',  ( -8.049105076161786076E-16, 33.40976562608393863, -13.14518615778179544 ) ) ;
#1298=CARTESIAN_POINT ( 'NONE',  ( 78.57481594606305464, 32.66562499999999858, -1.662435489736055892E-15 ) ) ;
#1300=CARTESIAN_POINT ( 'NONE',  ( 195.0000000000000000, 32.21914062608393436, 13.14518615778179544 ) ) ;
#1301=CARTESIAN_POINT ( 'NONE',  ( 129.4067442974502171, 35.99999999999998579, 13.13889047851776226 ) ) ;
#1303=DIRECTION ( 'NONE',  ( 0.000000000000000000, 0.000000000000000000, -1.000000000000000000 ) ) ;
#1309=CARTESIAN_POINT ( 'NONE',  ( 13.14518615778179900, 32.46718750108393436, -5.444914386472297529 ) ) ;
#1312=CARTESIAN_POINT ( 'NONE',  ( 95.54126587499995082, 83.75000000136560629, 1.846868145590724986 ) ) ;
#1316=CARTESIAN_POINT ( 'NONE',  ( 189.5550856135277229, 33.26093750108393721, -13.14518615778179900 ) ) ;
#1325=FACE_OUTER_BOUND ( 'NONE', #808, .T. ) ;
#1327=EDGE_CURVE ( 'NONE', #13666, #8880, #3265, .T. ) ;
#1328=VECTOR ( 'NONE', #13463, 1000.000000000000000 ) ;
#1329=CARTESIAN_POINT ( 'NONE',  ( 13.14518615778179722, 37.92421875108393436, 5.444914386472293977 ) ) ;
#1330=CARTESIAN_POINT ( 'NONE',  ( 13.14518615778179900, 40.40468750108393436, -5.444914386472297529 ) ) ;
#1336=( BOUNDED_CURVE ( )  B_SPLINE_CURVE ( 2, ( #22643, #11635, #15781, #20357, #552, #4972, #19926, #13916, #22073 ),
 .UNSPECIFIED., .F., .F. ) 
 B_SPLINE_CURVE_WITH_KNOTS ( ( 3, 2, 2, 2, 3 ),
 ( 0.3958333333333331483, 0.4062499999999999445, 0.4166666666666667407, 0.4270833333333335369, 0.4375000000000003331 ),
 .UNSPECIFIED. ) 
 CURVE ( )  GEOMETRIC_REPRESENTATION_ITEM ( )  RATIONAL_B_SPLINE_CURVE ( ( 1.000000000000001110, 0.9238795325112855172, 1.000000000000000000, 0.9238795325112867385, 1.000000000000000000, 0.9238795325112867385, 1.000000000000000000, 0.9238795325112842960, 1.000000000000002442 ) ) 
 REPRESENTATION_ITEM ( '' )  );
#1339=CARTESIAN_POINT ( 'NONE',  ( 101.8468681455907046, 83.37500000136563472, -4.458734125000016313 ) ) ;
#1341=CARTESIAN_POINT ( 'NONE',  ( 70.62287287157778337, 39.26367187716788010, -13.57481594606312036 ) ) ;
#1342=CARTESIAN_POINT ( 'NONE',  ( 70.31735157747590392, 54.47013368152370560, 14.99999999999998224 ) ) ;
#1343=ORIENTED_EDGE ( 'NONE', *, *, #14706, .F. ) ;
#1346=DIRECTION ( 'NONE',  ( 0.000000000000000000, 0.000000000000000000, 1.000000000000000000 ) ) ;
#1353=CARTESIAN_POINT ( 'NONE',  ( 65.00000000000000000, 39.36289062608393152, 13.14518615778179544 ) ) ;
#1357=ADVANCED_FACE ( 'NONE', ( #5225 ), #7343, .T. ) ;
#1358=CARTESIAN_POINT ( 'NONE',  ( 208.1451861577817795, 32.36796875108393579, 5.444914386472293977 ) ) ;
#1361=EDGE_CURVE ( 'NONE', #13666, #4294, #9219, .T. ) ;
#1363=CARTESIAN_POINT ( 'NONE',  ( 200.3173515774759608, 54.47013368152369139, 14.99999999999995026 ) ) ;
#1365=CARTESIAN_POINT ( 'NONE',  ( 124.3771271284221314, 38.07304687716787583, 13.57481594606304753 ) ) ;
#1366=DIRECTION ( 'NONE',  ( 0.000000000000000000, 1.000000000000000000, 0.000000000000000000 ) ) ;
#1367=CARTESIAN_POINT ( 'NONE',  ( -9.180175813647997174, 55.00000000000000000, 10.00000000000000000 ) ) ;
#1368=CARTESIAN_POINT ( 'NONE',  ( 204.2950502721270425, 38.66835937608393436, 9.295050272127046043 ) ) ;
#1369=VERTEX_POINT ( 'NONE', #14342 ) ;
#1371=CARTESIAN_POINT ( 'NONE',  ( -15.00000000000000355, 75.00000000000000000, -10.00000000000000000 ) ) ;
#1372=VECTOR ( 'NONE', #4847, 1000.000000000000227 ) ;
#1379=CARTESIAN_POINT ( 'NONE',  ( 97.92893218813449607, 83.18750000000001421, 4.999999999999968914 ) ) ;
#1384=CARTESIAN_POINT ( 'NONE',  ( 104.9999999999999716, 84.50000000000000000, -1.449011120738813565E-14 ) ) ;
#1388=CARTESIAN_POINT ( 'NONE',  ( 116.8548138422182205, 31.82226562608393650, 0.000000000000000000 ) ) ;
#1389=CARTESIAN_POINT ( 'NONE',  ( 51.85481384221819923, 36.53515625108392584, -5.444914386472297529 ) ) ;
#1390=CARTESIAN_POINT ( 'NONE',  ( 65.00000000000000000, -7.395377635281828788, -13.57481594606305109 ) ) ;
#1391=CARTESIAN_POINT ( 'NONE',  ( -8.049105076161786076E-16, 37.97382812608393721, -13.14518615778179544 ) ) ;
#1392=CARTESIAN_POINT ( 'NONE',  ( 214.9999999999999716, 80.00000000000000000, 0.000000000000000000 ) ) ;
#1395=CARTESIAN_POINT ( 'NONE',  ( 94.99999999999995737, 81.93750000000001421, -2.071067811865491493 ) ) ;
#1397=DIRECTION ( 'NONE',  ( 0.000000000000000000, 1.000000000000000000, 0.000000000000000000 ) ) ;
#1398=DIRECTION ( 'NONE',  ( -0.000000000000000000, -1.000000000000000000, -0.000000000000000000 ) ) ;
#1401=CARTESIAN_POINT ( 'NONE',  ( 131.4643377203195485, 35.99999999999999289, -13.46163418879038076 ) ) ;
#1412=CARTESIAN_POINT ( 'NONE',  ( 103.1528011352953342, 81.81250000136559208, 3.152801135295355106 ) ) ;
#1413=CARTESIAN_POINT ( 'NONE',  ( 78.14518615778179367, 37.13046875108393863, 5.444914386472293977 ) ) ;
#1416=( BOUNDED_CURVE ( )  B_SPLINE_CURVE ( 2, ( #25405, #18575, #1200, #26997, #3608, #14557, #27278, #18707, #25120 ),
 .UNSPECIFIED., .F., .F. ) 
 B_SPLINE_CURVE_WITH_KNOTS ( ( 3, 2, 2, 2, 3 ),
 ( 0.3125000000000002220, 0.3229166666666668517, 0.3333333333333334259, 0.3437500000000000555, 0.3541666666666666852 ),
 .UNSPECIFIED. ) 
 CURVE ( )  GEOMETRIC_REPRESENTATION_ITEM ( )  RATIONAL_B_SPLINE_CURVE ( ( 0.9999999999999983347, 0.9238795325112884038, 1.000000000000000000, 0.9238795325112867385, 1.000000000000000000, 0.9238795325112867385, 1.000000000000000000, 0.9238795325112867385, 1.000000000000000000 ) ) 
 REPRESENTATION_ITEM ( '' )  );
#1419=CARTESIAN_POINT ( 'NONE',  ( 116.8548138422182063, 33.55859375108393294, -5.444914386472297529 ) ) ;
#1420=VERTEX_POINT ( 'NONE', #3951 ) ;
#1421=CARTESIAN_POINT ( 'NONE',  ( 135.6228728715778118, 37.37851562716787157, 13.57481594606313813 ) ) ;
#1422=FACE_OUTER_BOUND ( 'NONE', #15581, .T. ) ;
#1423=CARTESIAN_POINT ( 'NONE',  ( 101.8468681455906903, 79.75000000136560629, 4.458734124999987891 ) ) ;
#1424=CARTESIAN_POINT ( 'NONE',  ( 143.1451861577818079, 40.20625000108393010, -5.444914386472297529 ) ) ;
#1425=CARTESIAN_POINT ( 'NONE',  ( 78.57481594606304043, 37.47773437716787726, 5.622872871577869525 ) ) ;
#1426=VECTOR ( 'NONE', #983, 1000.000000000000000 ) ;
#1427=CARTESIAN_POINT ( 'NONE',  ( 120.8198241863519939, 55.00000000000000000, 14.99999999999996803 ) ) ;
#1432=CARTESIAN_POINT ( 'NONE',  ( 204.5988444088204687, 32.66562500216787157, 9.598844408820456309 ) ) ;
#1433=B_SPLINE_CURVE_WITH_KNOTS ( 'NONE', 3,
 ( #17705, #15552, #13832, #5029, #15697, #4888, #2608, #22275, #26839, #754, #13695, #2749, #2329, #184, #15977, #15408, #24691, #20132 ),
 .UNSPECIFIED., .F., .F.,
 ( 4, 2, 2, 2, 2, 2, 2, 2, 4 ),
 ( 0.000000000000000000, 0.004618502246277256425, 0.006927753369415884203, 0.009237004492554512849, 0.01039163005412378597, 0.01154625561569305736, 0.01385550673883160361, 0.01616475786197014985, 0.01847400898510869610 ),
 .UNSPECIFIED. ) ;
#1434=CARTESIAN_POINT ( 'NONE',  ( 9.598844408820459861, 36.63437500216787157, 9.598844408820456309 ) ) ;
#1437=CARTESIAN_POINT ( 'NONE',  ( 135.4449143864723339, 38.71796875108393721, -13.14518615778179722 ) ) ;
#1442=CARTESIAN_POINT ( 'NONE',  ( 204.5988444088204687, 37.32890624999999574, 9.598844408820456309 ) ) ;
#1446=FACE_OUTER_BOUND ( 'NONE', #17803, .T. ) ;
#1451=CARTESIAN_POINT ( 'NONE',  ( 204.5988444088204403, 39.90859374999999432, -9.598844408820458085 ) ) ;
#1453=CARTESIAN_POINT ( 'NONE',  ( -5.622872871577873077, 40.85117187499999147, -13.57481594606304753 ) ) ;
#1455=CARTESIAN_POINT ( 'NONE',  ( 95.54126587499995082, 84.62500000136560629, -1.846868145590750077 ) ) ;
#1457=VERTEX_POINT ( 'NONE', #5814 ) ;
#1459=CARTESIAN_POINT ( 'NONE',  ( 199.9250267836615649, 49.99999999893046976, -12.67776588291885176 ) ) ;
#1461=EDGE_LOOP ( 'NONE', ( #5171, #21822, #933, #7782 ) ) ;
#1468=CARTESIAN_POINT ( 'NONE',  ( 116.8548138422182205, 39.90859375108393436, -5.444914386472297529 ) ) ;
#1469=CARTESIAN_POINT ( 'NONE',  ( -8.049105076161786076E-16, 32.41757812608393863, -13.14518615778179544 ) ) ;
#1470=ORIENTED_EDGE ( 'NONE', *, *, #4634, .F. ) ;
#1471=CARTESIAN_POINT ( 'NONE',  ( 59.37712712842213136, 37.18007812500000853, 13.57481594606304753 ) ) ;
#1477=CARTESIAN_POINT ( 'NONE',  ( 103.1528011352953342, 83.31250000136560629, -3.152801135295383084 ) ) ;
#1479=CARTESIAN_POINT ( 'NONE',  ( -5.444914386472297529, 40.60312500108393863, -13.14518615778179900 ) ) ;
#1480=CARTESIAN_POINT ( 'NONE',  ( 189.3771271284221598, 38.76757812499998579, 13.57481594606308128 ) ) ;
#1481=ORIENTED_EDGE ( 'NONE', *, *, #18913, .F. ) ;
#1483=CYLINDRICAL_SURFACE ( 'NONE', #6331, 5.000000000000000888 ) ;
#1486=CARTESIAN_POINT ( 'NONE',  ( 99.99999999999995737, 84.75000000000000000, -5.000000000000018652 ) ) ;
#1488=DIRECTION ( 'NONE',  ( -0.000000000000000000, 1.000000000000000000, -0.000000000000000000 ) ) ;
#1490=CARTESIAN_POINT ( 'NONE',  ( 70.44491438647229131, 39.71015625108393010, -13.14518615778179722 ) ) ;
#1491=CARTESIAN_POINT ( 'NONE',  ( 65.00000000000000000, -7.395377635281828788, -7.517135062566165128E-15 ) ) ;
#1493=DIRECTION ( 'NONE',  ( 0.000000000000000000, 0.000000000000000000, 1.000000000000000000 ) ) ;
#1495=CARTESIAN_POINT ( 'NONE',  ( 78.57481594606305464, 37.47773437500001137, -5.622872871577873966 ) ) ;
#1496=CARTESIAN_POINT ( 'NONE',  ( -6.119843627700299216, 51.28708186914936817, -15.00000000000000178 ) ) ;
#1497=CARTESIAN_POINT ( 'NONE',  ( 99.99999999999995737, 79.37500000273119838, 4.999999999999990230 ) ) ;
#1498=( BOUNDED_SURFACE ( )  B_SPLINE_SURFACE ( 1, 2, ( 
 ( #23433, #8595, #1778, #1639, #19293, #25842, #27993, #10298, #12848, #25703, #2196, #27854, #21723, #17427, #6317, #3907, #12569, #10858, #2051, #10443, #21576, #10721, #19430, #19150, #17285, #54, #8734, #14852, #26125, #6592, #27717, #19004, #8178, #4470, #26272, #26418, #2337, #9024, #13413, #26560, #11424, #24271, #24410, #4899, #17716, #2761, #13562, #15419, #17855, #10995, #481, #5040, #24133, #20143, #2474, #624, #9299, #19709, #337, #24558, #23992, #2618, #21863, #22285, #193, #15708, #4753, #6877, #11135, #13266, #15849, #9163, #6733, #13128, #8875, #15562, #17995, #17567, #4609, #22139, #7012, #11281, #21998, #20001, #19850, #26704, #7153, #15227, #21671, #4425, #2148, #12671, #23527, #10810, #4143, #15083, #19664, #21528, #14804, #13079, #8404, #19525, #10953, #10397, #23803, #10538, #2005, #21818, #17522, #16955, #4005, #21251, #14949, #6138, #28085, #26225, #25656, #1733, #21396, #6684, #17381, #25795, #1874, #23945, #6547, #6, #19245, #24087, #12938, #4561, #26079, #2294, #19105, #27812, #6272, #6414, #25940, #8832, #27945, #147, #15370, #23668, #12806, #8267, #19381, #4281, #17093, #10672, #8691, #8548, #17237, #26370, #2575, #8975, #24659, #11379, #869, #19806, #17951, #18091, #24511, #2718, #5132, #4999, #13662, #13798, #22377, #17664, #20100, #16087, #24365, #21955, #26803, #20383, #719, #13518, #20237, #26514, #17811, #19954, #11518, #7108, #9394 ),
 ( #2434, #6971, #6829, #290, #24793, #577, #22522, #9541, #22097, #9258, #4853, #15806, #11236, #13223, #11094, #2849, #2987, #15519, #15943, #7253, #11661, #22239, #18242, #24227, #4708, #13368, #26950, #7393, #15666, #432, #26661, #9116, #16842, #12538, #16705, #5744, #27685, #18840, #21265, #10689, #10128, #14414, #27548, #19396, #1890, #10267, #8004, #8419, #19262, #6154, #3742, #8565, #25671, #17255, #10553, #14964, #23129, #12264, #18977, #19121, #10414, #21545, #23269, #17108, #27962, #8149, #25539, #3605, #3878, #27828, #25403, #6287, #23543, #20990, #4019, #5885, #12402, #1471, #25813, #1748, #2020, #14554, #8281, #23684, #16972, #23403, #4161, #14820, #12685, #12821, #21411, #21124, #28101, #1610, #6019, #14682, #11252, #4869, #13383, #26241, #4723, #10967, #2310, #4440, #24241, #19822, #22111, #24100, #165, #25956, #2590, #15386, #26529, #10825, #9131, #306, #4297, #19969, #4578, #17537, #21833, #15241, #2730, #17682, #23, #11395, #13533, #13092, #8992, #6985, #24381, #6699, #8705, #6561, #17824, #448, #26096, #26388, #13238, #21970, #19541, #11108, #15680, #6843, #17398, #15533, #23961, #21688, #19679, #9270, #6429, #8847, #2447, #12955, #22253, #20114, #591, #15098, #23819, #2163, #22824, #9555, #9833, #3292, #26820, #16250, #13676, #18397, #1298, #7267, #18540, #22535, #7700, #27244, #22392, #883, #20820, #17966, #22682, #7122, #11962, #26675, #3003 ) ),
 .UNSPECIFIED., .F., .F., .F. ) 
 B_SPLINE_SURFACE_WITH_KNOTS ( ( 2, 2 ),
 ( 3, 2, 2, 2, 2, 2, 2, 2, 2, 2, 2, 2, 2, 2, 2, 2, 2, 2, 2, 2, 2, 2, 2, 2, 2, 2, 2, 2, 2, 2, 2, 2, 2, 2, 2, 2, 2, 2, 2, 2, 2, 2, 2, 2, 2, 2, 2, 2, 2, 2, 2, 2, 2, 2, 2, 2, 2, 2, 2, 2, 2, 2, 2, 2, 2, 2, 2, 2, 2, 2, 2, 2, 2, 2, 2, 2, 2, 2, 2, 2, 2, 2, 2, 2, 2, 2, 2, 2, 2, 2, 2, 3 ),
 ( 0.000000000000000000, 1.000000000000000000 ),
 ( 0.000000000000000000, 0.01041666666666666609, 0.02083333333333333218, 0.03125000000000000000, 0.04166666666666666435, 0.05208333333333333565, 0.06250000000000000000, 0.07291666666666667129, 0.08333333333333332871, 0.09375000000000000000, 0.1041666666666666713, 0.1145833333333333287, 0.1250000000000000000, 0.1354166666666666574, 0.1458333333333333426, 0.1562500000000000000, 0.1666666666666666574, 0.1770833333333333426, 0.1875000000000000000, 0.1979166666666666574, 0.2083333333333333426, 0.2187500000000000000, 0.2291666666666666574, 0.2395833333333333426, 0.2500000000000000000, 0.2604166666666666852, 0.2708333333333333148, 0.2812500000000000000, 0.2916666666666666852, 0.3020833333333333148, 0.3125000000000000000, 0.3229166666666666852, 0.3333333333333333148, 0.3437500000000000000, 0.3541666666666666852, 0.3645833333333333148, 0.3750000000000000000, 0.3854166666666666852, 0.3958333333333333148, 0.4062500000000000000, 0.4166666666666666852, 0.4270833333333333148, 0.4375000000000000000, 0.4479166666666666852, 0.4583333333333333148, 0.4687500000000000000, 0.4791666666666666852, 0.4895833333333333148, 0.5000000000000000000, 0.5104166666666666297, 0.5208333333333333703, 0.5312500000000000000, 0.5416666666666666297, 0.5520833333333333703, 0.5625000000000000000, 0.5729166666666666297, 0.5833333333333333703, 0.5937500000000000000, 0.6041666666666666297, 0.6145833333333333703, 0.6250000000000000000, 0.6354166666666666297, 0.6458333333333333703, 0.6562500000000000000, 0.6666666666666666297, 0.6770833333333333703, 0.6875000000000000000, 0.6979166666666666297, 0.7083333333333333703, 0.7187500000000000000, 0.7291666666666666297, 0.7395833333333333703, 0.7500000000000000000, 0.7604166666666666297, 0.7708333333333333703, 0.7812500000000000000, 0.7916666666666666297, 0.8020833333333333703, 0.8125000000000000000, 0.8229166666666666297, 0.8333333333333333703, 0.8437500000000000000, 0.8541666666666666297, 0.8645833333333333703, 0.8750000000000000000, 0.8854166666666666297, 0.8958333333333333703, 0.9062500000000000000, 0.9166666666666666297, 0.9270833333333333703, 0.9375000000000000000, 0.9448586968893691873 ),
 .UNSPECIFIED. ) 
 GEOMETRIC_REPRESENTATION_ITEM ( )  RATIONAL_B_SPLINE_SURFACE ( (
 ( 1.000000000000000000, 0.9238795325112867385, 1.000000000000000000, 0.9238795325112867385, 1.000000000000000000, 0.9238795325112867385, 1.000000000000000000, 0.9238795325112867385, 1.000000000000000000, 0.9238795325112867385, 1.000000000000000000, 0.9238795325112867385, 1.000000000000000000, 0.9238795325112867385, 1.000000000000000000, 0.9238795325112867385, 1.000000000000000000, 0.9238795325112867385, 1.000000000000000000, 0.9238795325112867385, 1.000000000000000000, 0.9238795325112867385, 1.000000000000000000, 0.9238795325112867385, 1.000000000000000000, 0.9238795325112867385, 1.000000000000000000, 0.9238795325112867385, 1.000000000000000000, 0.9238795325112867385, 1.000000000000000000, 0.9238795325112867385, 1.000000000000000000, 0.9238795325112867385, 1.000000000000000000, 0.9238795325112867385, 1.000000000000000000, 0.9238795325112867385, 1.000000000000000000, 0.9238795325112867385, 1.000000000000000000, 0.9238795325112867385, 1.000000000000000000, 0.9238795325112867385, 1.000000000000000000, 0.9238795325112867385, 1.000000000000000000, 0.9238795325112867385, 1.000000000000000000, 0.9238795325112867385, 1.000000000000000000, 0.9238795325112867385, 1.000000000000000000, 0.9238795325112867385, 1.000000000000000000, 0.9238795325112867385, 1.000000000000000000, 0.9238795325112867385, 1.000000000000000000, 0.9238795325112867385, 1.000000000000000000, 0.9238795325112867385, 1.000000000000000000, 0.9238795325112867385, 1.000000000000000000, 0.9238795325112867385, 1.000000000000000000, 0.9238795325112867385, 1.000000000000000000, 0.9238795325112867385, 1.000000000000000000, 0.9238795325112867385, 1.000000000000000000, 0.9238795325112867385, 1.000000000000000000, 0.9238795325112867385, 1.000000000000000000, 0.9238795325112867385, 1.000000000000000000, 0.9238795325112867385, 1.000000000000000000, 0.9238795325112867385, 1.000000000000000000, 0.9238795325112867385, 1.000000000000000000, 0.9238795325112867385, 1.000000000000000000, 0.9238795325112867385, 1.000000000000000000, 0.9238795325112867385, 1.000000000000000000, 0.9238795325112867385, 1.000000000000000000, 0.9238795325112867385, 1.000000000000000000, 0.9238795325112867385, 1.000000000000000000, 0.9238795325112867385, 1.000000000000000000, 0.9238795325112867385, 1.000000000000000000, 0.9238795325112867385, 1.000000000000000000, 0.9238795325112867385, 1.000000000000000000, 0.9238795325112867385, 1.000000000000000000, 0.9238795325112867385, 1.000000000000000000, 0.9238795325112867385, 1.000000000000000000, 0.9238795325112867385, 1.000000000000000000, 0.9238795325112867385, 1.000000000000000000, 0.9238795325112867385, 1.000000000000000000, 0.9238795325112867385, 1.000000000000000000, 0.9238795325112867385, 1.000000000000000000, 0.9238795325112867385, 1.000000000000000000, 0.9238795325112867385, 1.000000000000000000, 0.9238795325112867385, 1.000000000000000000, 0.9238795325112867385, 1.000000000000000000, 0.9238795325112867385, 1.000000000000000000, 0.9238795325112867385, 1.000000000000000000, 0.9238795325112867385, 1.000000000000000000, 0.9238795325112867385, 1.000000000000000000, 0.9238795325112867385, 1.000000000000000000, 0.9238795325112867385, 1.000000000000000000, 0.9238795325112867385, 1.000000000000000000, 0.9238795325112867385, 1.000000000000000000, 0.9238795325112867385, 1.000000000000000000, 0.9238795325112867385, 1.000000000000000000, 0.9238795325112867385, 1.000000000000000000, 0.9238795325112867385, 1.000000000000000000, 0.9238795325112867385, 1.000000000000000000, 0.9238795325112867385, 1.000000000000000000, 0.9238795325112867385, 1.000000000000000000, 0.9238795325112867385, 1.000000000000000000, 0.9238795325112867385, 1.000000000000000000, 0.9238795325112867385, 1.000000000000000000, 0.9238795325112867385, 1.000000000000000000, 0.9238795325112867385, 1.000000000000000000, 0.9238795325112867385, 1.000000000000000000, 0.9238795325112867385, 1.000000000000000000, 0.9238795325112867385, 1.000000000000000000, 0.9238795325112867385, 1.000000000000000000, 0.9238795325112867385, 1.000000000000000000, 0.9238795325112867385, 1.000000000000000000, 0.9462258450566536361, 0.9684275698016389100),
 ( 1.000000000000000000, 0.9238795325112867385, 1.000000000000000000, 0.9238795325112867385, 1.000000000000000000, 0.9238795325112867385, 1.000000000000000000, 0.9238795325112867385, 1.000000000000000000, 0.9238795325112867385, 1.000000000000000000, 0.9238795325112867385, 1.000000000000000000, 0.9238795325112867385, 1.000000000000000000, 0.9238795325112867385, 1.000000000000000000, 0.9238795325112867385, 1.000000000000000000, 0.9238795325112867385, 1.000000000000000000, 0.9238795325112867385, 1.000000000000000000, 0.9238795325112867385, 1.000000000000000000, 0.9238795325112867385, 1.000000000000000000, 0.9238795325112867385, 1.000000000000000000, 0.9238795325112867385, 1.000000000000000000, 0.9238795325112867385, 1.000000000000000000, 0.9238795325112867385, 1.000000000000000000, 0.9238795325112867385, 1.000000000000000000, 0.9238795325112867385, 1.000000000000000000, 0.9238795325112867385, 1.000000000000000000, 0.9238795325112867385, 1.000000000000000000, 0.9238795325112867385, 1.000000000000000000, 0.9238795325112867385, 1.000000000000000000, 0.9238795325112867385, 1.000000000000000000, 0.9238795325112867385, 1.000000000000000000, 0.9238795325112867385, 1.000000000000000000, 0.9238795325112867385, 1.000000000000000000, 0.9238795325112867385, 1.000000000000000000, 0.9238795325112867385, 1.000000000000000000, 0.9238795325112867385, 1.000000000000000000, 0.9238795325112867385, 1.000000000000000000, 0.9238795325112867385, 1.000000000000000000, 0.9238795325112867385, 1.000000000000000000, 0.9238795325112867385, 1.000000000000000000, 0.9238795325112867385, 1.000000000000000000, 0.9238795325112867385, 1.000000000000000000, 0.9238795325112867385, 1.000000000000000000, 0.9238795325112867385, 1.000000000000000000, 0.9238795325112867385, 1.000000000000000000, 0.9238795325112867385, 1.000000000000000000, 0.9238795325112867385, 1.000000000000000000, 0.9238795325112867385, 1.000000000000000000, 0.9238795325112867385, 1.000000000000000000, 0.9238795325112867385, 1.000000000000000000, 0.9238795325112867385, 1.000000000000000000, 0.9238795325112867385, 1.000000000000000000, 0.9238795325112867385, 1.000000000000000000, 0.9238795325112867385, 1.000000000000000000, 0.9238795325112867385, 1.000000000000000000, 0.9238795325112867385, 1.000000000000000000, 0.9238795325112867385, 1.000000000000000000, 0.9238795325112867385, 1.000000000000000000, 0.9238795325112867385, 1.000000000000000000, 0.9238795325112867385, 1.000000000000000000, 0.9238795325112867385, 1.000000000000000000, 0.9238795325112867385, 1.000000000000000000, 0.9238795325112867385, 1.000000000000000000, 0.9238795325112867385, 1.000000000000000000, 0.9238795325112867385, 1.000000000000000000, 0.9238795325112867385, 1.000000000000000000, 0.9238795325112867385, 1.000000000000000000, 0.9238795325112867385, 1.000000000000000000, 0.9238795325112867385, 1.000000000000000000, 0.9238795325112867385, 1.000000000000000000, 0.9238795325112867385, 1.000000000000000000, 0.9238795325112867385, 1.000000000000000000, 0.9238795325112867385, 1.000000000000000000, 0.9238795325112867385, 1.000000000000000000, 0.9238795325112867385, 1.000000000000000000, 0.9238795325112867385, 1.000000000000000000, 0.9238795325112867385, 1.000000000000000000, 0.9238795325112867385, 1.000000000000000000, 0.9238795325112867385, 1.000000000000000000, 0.9238795325112867385, 1.000000000000000000, 0.9238795325112867385, 1.000000000000000000, 0.9238795325112867385, 1.000000000000000000, 0.9238795325112867385, 1.000000000000000000, 0.9238795325112867385, 1.000000000000000000, 0.9238795325112867385, 1.000000000000000000, 0.9238795325112867385, 1.000000000000000000, 0.9238795325112867385, 1.000000000000000000, 0.9238795325112867385, 1.000000000000000000, 0.9238795325112867385, 1.000000000000000000, 0.9238795325112867385, 1.000000000000000000, 0.9238795325112867385, 1.000000000000000000, 0.9238795325112867385, 1.000000000000000000, 0.9238795325112867385, 1.000000000000000000, 0.9238795325112867385, 1.000000000000000000, 0.9238795325112867385, 1.000000000000000000, 0.9238795325112867385, 1.000000000000000000, 0.9462258450566536361, 0.9684275698016389100) ) ) 
 REPRESENTATION_ITEM ( '' )  SURFACE ( )  );
#1500=CARTESIAN_POINT ( 'NONE',  ( 135.6228728715778686, 33.70742187716787441, -13.57481594606304753 ) ) ;
#1504=CARTESIAN_POINT ( 'NONE',  ( 200.4449143864723055, 36.53515625108393294, -13.14518615778179900 ) ) ;
#1508=CARTESIAN_POINT ( 'NONE',  ( 94.99999999999995737, 83.93750000000001421, -2.071067811865491493 ) ) ;
#1511=CARTESIAN_POINT ( 'NONE',  ( 104.4587341249999639, 82.93750000136560629, -1.442382525525748735E-14 ) ) ;
#1515=CARTESIAN_POINT ( 'NONE',  ( 3.829562757991920474, 36.00000000000001421, 12.63428651647591749 ) ) ;
#1517=CARTESIAN_POINT ( 'NONE',  ( 139.5988444088204687, 32.56640625000000000, 9.598844408820456309 ) ) ;
#1520=EDGE_LOOP ( 'NONE', ( #5314, #1279, #18882, #7280 ) ) ;
#1526=CARTESIAN_POINT ( 'NONE',  ( 139.2950502721270425, 38.66835937608393436, 9.295050272127046043 ) ) ;
#1527=CARTESIAN_POINT ( 'NONE',  ( 78.14518615778179367, 35.39414062608393152, -1.609821015232357215E-15 ) ) ;
#1528=LINE ( 'NONE', #1390, #19800 ) ;
#1529=CARTESIAN_POINT ( 'NONE',  ( -13.14518615778179900, 34.94765625108392726, -5.444914386472297529 ) ) ;
#1530=CARTESIAN_POINT ( 'NONE',  ( 194.8277102352230941, 36.00000000000000000, -13.51468191220837056 ) ) ;
#1531=DIRECTION ( 'NONE',  ( 0.000000000000000000, 0.000000000000000000, -1.000000000000000000 ) ) ;
#1533=CARTESIAN_POINT ( 'NONE',  ( 96.46446609406721961, 82.12500000000000000, 3.535533905932727539 ) ) ;
#1534=ORIENTED_EDGE ( 'NONE', *, *, #25184, .T. ) ;
#1535=FACE_OUTER_BOUND ( 'NONE', #27394, .T. ) ;
#1536=CARTESIAN_POINT ( 'NONE',  ( -13.14518615778179900, 39.71015625108393010, -5.444914386472297529 ) ) ;
#1537=CARTESIAN_POINT ( 'NONE',  ( 132.2323271553379698, 35.99999999999999289, 12.98409812936879426 ) ) ;
#1543=DIRECTION ( 'NONE',  ( -0.000000000000000000, -1.000000000000000000, -0.000000000000000000 ) ) ;
#1547=ORIENTED_EDGE ( 'NONE', *, *, #18203, .T. ) ;
#1553=CARTESIAN_POINT ( 'NONE',  ( 103.1528011352953342, 84.06250000136560629, 3.152801135295355106 ) ) ;
#1554=CARTESIAN_POINT ( 'NONE',  ( 65.00000000000000000, 38.96601562608393721, -13.14518615778179544 ) ) ;
#1560=CARTESIAN_POINT ( 'NONE',  ( 139.5988444088204403, 39.90859374999999432, -9.598844408820458085 ) ) ;
#1561=ADVANCED_FACE ( 'NONE', ( #20006 ), #6356, .F. ) ;
#1565=CARTESIAN_POINT ( 'NONE',  ( 101.8468681455906903, 80.75000000136560629, 4.458734124999987891 ) ) ;
#1566=CARTESIAN_POINT ( 'NONE',  ( 135.4449143864723055, 38.42031250108393436, 13.14518615778179189 ) ) ;
#1567=CARTESIAN_POINT ( 'NONE',  ( 51.42518405393695957, 35.54296875216788010, 0.000000000000000000 ) ) ;
#1569=CARTESIAN_POINT ( 'NONE',  ( -13.57481594606304576, 37.18007812716787441, 5.622872871577880183 ) ) ;
#1572=LINE ( 'NONE', #17352, #10785 ) ;
#1574=CARTESIAN_POINT ( 'NONE',  ( 200.4449143864723055, 37.62656250108393863, 13.14518615778179189 ) ) ;
#1576=CARTESIAN_POINT ( 'NONE',  ( 143.1451861577818363, 37.72578125108393010, 5.444914386472293977 ) ) ;
#1581=CARTESIAN_POINT ( 'NONE',  ( 55.40115559117954547, 36.93203124999999432, -9.598844408820458085 ) ) ;
#1583=CARTESIAN_POINT ( 'NONE',  ( 195.0000000000000000, 38.02343749999999289, 13.57481594606304576 ) ) ;
#1584=CARTESIAN_POINT ( 'NONE',  ( 130.7050241099688606, 36.00000000000000711, 13.13343125082108465 ) ) ;
#1586=CARTESIAN_POINT ( 'NONE',  ( 70.44491438647230552, 37.62656250108393863, 13.14518615778179189 ) ) ;
#1592=CARTESIAN_POINT ( 'NONE',  ( 9.598844408820456309, 38.32109374999999574, -9.598844408820458085 ) ) ;
#1593=ORIENTED_EDGE ( 'NONE', *, *, #14238, .T. ) ;
#1594=CARTESIAN_POINT ( 'NONE',  ( 99.99999999999995737, 83.93750000136560629, 4.458734124999988779 ) ) ;
#1598=CARTESIAN_POINT ( 'NONE',  ( 133.1165920804657787, 53.90895096933309105, -15.00000000000000178 ) ) ;
#1601=ORIENTED_EDGE ( 'NONE', *, *, #2716, .F. ) ;
#1604=CARTESIAN_POINT ( 'NONE',  ( 181.4251840539369596, 39.51171875216787299, 0.000000000000000000 ) ) ;
#1607=CARTESIAN_POINT ( 'NONE',  ( 2.414731522848535132E-15, 32.02070312608393010, 13.14518615778179544 ) ) ;
#1610=CARTESIAN_POINT ( 'NONE',  ( 59.37712712842213136, 36.38632812499999858, 13.57481594606304753 ) ) ;
#1612=CARTESIAN_POINT ( 'NONE',  ( 202.7541239759955829, 36.00000000000001421, 10.77549638133708676 ) ) ;
#1616=CARTESIAN_POINT ( 'NONE',  ( 99.99999999999995737, 83.93750000136560629, 4.458734124999988779 ) ) ;
#1618=CARTESIAN_POINT ( 'NONE',  ( -5.444914386472297529, 39.01562500108394005, -13.14518615778179900 ) ) ;
#1623=CYLINDRICAL_SURFACE ( 'NONE', #4366, 13.57481594606304398 ) ;
#1626=AXIS2_PLACEMENT_3D ( 'NONE', #4454, #2324, #10980 ) ;
#1629=CARTESIAN_POINT ( 'NONE',  ( 78.14518615778180788, 39.51171875108393294, 5.444914386472293977 ) ) ;
#1630=DIRECTION ( 'NONE',  ( 0.000000000000000000, 0.000000000000000000, 1.000000000000000000 ) ) ;
#1631=CARTESIAN_POINT ( 'NONE',  ( 72.62394196192546758, 55.00000000000000000, -14.99999999999999822 ) ) ;
#1632=ORIENTED_EDGE ( 'NONE', *, *, #20818, .T. ) ;
#1633=CARTESIAN_POINT ( 'NONE',  ( -6.873508243570724652, 51.14166184781385027, -15.00000000000000000 ) ) ;
#1635=CIRCLE ( 'NONE', #17545, 11.57481594606304398 ) ;
#1636=CARTESIAN_POINT ( 'NONE',  ( 198.7974518689581203, 54.08938259242987101, 14.99999999999995204 ) ) ;
#1637=CARTESIAN_POINT ( 'NONE',  ( 120.4011555911795455, 33.06250000216787299, -9.598844408820458085 ) ) ;
#1638=EDGE_CURVE ( 'NONE', #13131, #13869, #14467, .T. ) ;
#1639=CARTESIAN_POINT ( 'NONE',  ( 59.55508561352770158, 40.60312500108393863, -13.14518615778179900 ) ) ;
#1641=CARTESIAN_POINT ( 'NONE',  ( 181.8548138422181921, 37.62656250108393863, 5.444914386472304635 ) ) ;
#1642=ORIENTED_EDGE ( 'NONE', *, *, #5660, .T. ) ;
#1645=CARTESIAN_POINT ( 'NONE',  ( 1.662435489736055498E-15, -7.395377635281828788, -13.57481594606304398 ) ) ;
#1646=CARTESIAN_POINT ( 'NONE',  ( 143.5748159460630688, 39.90859375216787441, -1.662435489736055892E-15 ) ) ;
#1648=AXIS2_PLACEMENT_3D ( 'NONE', #12860, #351, #11008 ) ;
#1649=CARTESIAN_POINT ( 'NONE',  ( 13.40642364673431786, 36.00000000000000000, 1.227293221036820592 ) ) ;
#1656=( BOUNDED_CURVE ( )  B_SPLINE_CURVE ( 2, ( #6524, #26347, #15202, #4832, #23922, #4400, #13055, #13492, #1985 ),
 .UNSPECIFIED., .F., .F. ) 
 B_SPLINE_CURVE_WITH_KNOTS ( ( 3, 2, 2, 2, 3 ),
 ( 0.4375000000000003331, 0.4479166666666669627, 0.4583333333333335369, 0.4687500000000001665, 0.4791666666666667962 ),
 .UNSPECIFIED. ) 
 CURVE ( )  GEOMETRIC_REPRESENTATION_ITEM ( )  RATIONAL_B_SPLINE_CURVE ( ( 0.9999999999999975575, 0.9238795325112891810, 1.000000000000000000, 0.9238795325112867385, 1.000000000000000000, 0.9238795325112867385, 1.000000000000000000, 0.9238795325112859613, 1.000000000000000888 ) ) 
 REPRESENTATION_ITEM ( '' )  );
#1658=CARTESIAN_POINT ( 'NONE',  ( 130.0000000000000000, 38.96601562608393721, -13.14518615778179544 ) ) ;
#1659=CARTESIAN_POINT ( 'NONE',  ( 74.29505027212704249, 36.88242187608393152, 9.295050272127046043 ) ) ;
#1660=CARTESIAN_POINT ( 'NONE',  ( 195.0000000000000000, 39.36289062608393152, 13.14518615778179544 ) ) ;
#1661=ORIENTED_EDGE ( 'NONE', *, *, #20702, .T. ) ;
#1662=DIRECTION ( 'NONE',  ( 0.000000000000000000, 1.000000000000000000, 0.000000000000000000 ) ) ;
#1663=CARTESIAN_POINT ( 'NONE',  ( -5.444914386472297529, 34.05468750108393294, -13.14518615778179900 ) ) ;
#1664=CARTESIAN_POINT ( 'NONE',  ( 59.37712712842208873, 36.08867187500000284, -13.57481594606300135 ) ) ;
#1666=ADVANCED_FACE ( 'NONE', ( #9303 ), #6880, .T. ) ;
#1667=CARTESIAN_POINT ( 'NONE',  ( 195.0000000000000000, 36.00000000000000000, 11.57481594606302266 ) ) ;
#1668=CARTESIAN_POINT ( 'NONE',  ( 0.000000000000000000, 50.00000000000000000, 0.000000000000000000 ) ) ;
#1669=EDGE_CURVE ( 'NONE', #22877, #13724, #8295, .T. ) ;
#1671=CARTESIAN_POINT ( 'NONE',  ( -5.444914386472299306, 37.52734375108393294, 13.14518615778179722 ) ) ;
#1677=CARTESIAN_POINT ( 'NONE',  ( 195.0000000000000000, 39.31328125216787583, -13.57481594606304576 ) ) ;
#1680=ORIENTED_EDGE ( 'NONE', *, *, #8274, .T. ) ;
#1683=EDGE_CURVE ( 'NONE', #22301, #23304, #28064, .T. ) ;
#1686=CARTESIAN_POINT ( 'NONE',  ( 95.54126587499995082, 81.50000000136560629, 1.846868145590724986 ) ) ;
#1687=CARTESIAN_POINT ( 'NONE',  ( 59.55508561352770158, 39.01562500108394005, -13.14518615778179900 ) ) ;
#1693=CARTESIAN_POINT ( 'NONE',  ( 65.00000000000000000, -7.395377635281828788, 13.57481594606303688 ) ) ;
#1695=CARTESIAN_POINT ( 'NONE',  ( 116.8548138422182063, 32.86406250108393579, 5.444914386472304635 ) ) ;
#1696=VERTEX_POINT ( 'NONE', #3462 ) ;
#1697=CARTESIAN_POINT ( 'NONE',  ( -5.317351577475888824, 54.47013368152369850, -14.99999999999999822 ) ) ;
#1699=CARTESIAN_POINT ( 'NONE',  ( 98.15313185440925281, 80.62500000136559208, 4.458734124999987891 ) ) ;
#1701=CARTESIAN_POINT ( 'NONE',  ( 55.40115559117954547, 37.03125000216787299, -9.598844408820458085 ) ) ;
#1703=CARTESIAN_POINT ( 'NONE',  ( 2.493653234604083739E-15, 34.94765625216787441, 13.57481594606304576 ) ) ;
#1704=ORIENTED_EDGE ( 'NONE', *, *, #25691, .F. ) ;
#1705=EDGE_CURVE ( 'NONE', #14872, #27029, #26233, .T. ) ;
#1709=CARTESIAN_POINT ( 'NONE',  ( 204.2950502721270425, 37.67617187608393436, 9.295050272127046043 ) ) ;
#1711=CARTESIAN_POINT ( 'NONE',  ( 120.7049497278729575, 36.68398437608392726, 9.295050272127047819 ) ) ;
#1712=CARTESIAN_POINT ( 'NONE',  ( 185.4011555911795313, 37.82500000216787583, -9.598844408820458085 ) ) ;
#1715=DIRECTION ( 'NONE',  ( 0.000000000000000000, 0.000000000000000000, -1.000000000000000000 ) ) ;
#1717=CARTESIAN_POINT ( 'NONE',  ( 189.3771271284221314, 37.67617187499999432, -13.57481594606304753 ) ) ;
#1720=CARTESIAN_POINT ( 'NONE',  ( 74.29505027212704249, 38.66835937608393436, -9.295050272127046043 ) ) ;
#1724=CARTESIAN_POINT ( 'NONE',  ( 124.3771271284219893, 39.56132812500000284, 13.57481594606290720 ) ) ;
#1725=CARTESIAN_POINT ( 'NONE',  ( 9.598844408820459861, 39.71015624999999716, 9.598844408820456309 ) ) ;
#1728=CARTESIAN_POINT ( 'NONE',  ( 98.15313185440925281, 81.50000000136560629, -4.458734125000016313 ) ) ;
#1729=VECTOR ( 'NONE', #17391, 1000.000000000000000 ) ;
#1733=CARTESIAN_POINT ( 'NONE',  ( 70.44491438647230552, 34.94765625108394147, -13.14518615778179900 ) ) ;
#1735=CARTESIAN_POINT ( 'NONE',  ( -9.598844408820458085, 36.93203124999999432, -9.598844408820458085 ) ) ;
#1737=ORIENTED_EDGE ( 'NONE', *, *, #3048, .T. ) ;
#1738=DIRECTION ( 'NONE',  ( 1.000000000000000000, 0.000000000000000000, -7.228014483236696740E-18 ) ) ;
#1740=CARTESIAN_POINT ( 'NONE',  ( 200.6228728715778686, 36.88242187716787157, -13.57481594606304753 ) ) ;
#1743=FACE_OUTER_BOUND ( 'NONE', #8237, .T. ) ;
#1744=CARTESIAN_POINT ( 'NONE',  ( 201.4128666762415492, 50.00000000108515508, 11.99502265408284707 ) ) ;
#1745=CARTESIAN_POINT ( 'NONE',  ( 120.7049497278729575, 40.05742187608393579, 9.295050272127047819 ) ) ;
#1746=CARTESIAN_POINT ( 'NONE',  ( -5.444914386472299306, 38.51953125108393294, 13.14518615778179722 ) ) ;
#1747=ORIENTED_EDGE ( 'NONE', *, *, #23271, .F. ) ;
#1748=CARTESIAN_POINT ( 'NONE',  ( 51.42518405393695957, 37.08085937499999574, 5.622872871577880183 ) ) ;
#1750=VECTOR ( 'NONE', #2106, 1000.000000000000000 ) ;
#1755=CARTESIAN_POINT ( 'NONE',  ( 104.4587341249999781, 84.25000000136559208, -1.846868145590750521 ) ) ;
#1757=CARTESIAN_POINT ( 'NONE',  ( 13.14518615778179900, 38.81718750108393579, -5.444914386472297529 ) ) ;
#1758=CARTESIAN_POINT ( 'NONE',  ( 185.4011555911795597, 38.71796874999999716, 9.598844408820459861 ) ) ;
#1761=CARTESIAN_POINT ( 'NONE',  ( 1.417506129906585004E-15, -7.395377635281828788, -11.57481594606304398 ) ) ;
#1767=CARTESIAN_POINT ( 'NONE',  ( 78.14518615778180788, 38.81718750108393579, -5.444914386472297529 ) ) ;
#1769=AXIS2_PLACEMENT_3D ( 'NONE', #11651, #14079, #22799 ) ;
#1770=VECTOR ( 'NONE', #15736, 1000.000000000000227 ) ;
#1771=CARTESIAN_POINT ( 'NONE',  ( 181.8548138422181921, 31.97109375108393436, -5.444914386472297529 ) ) ;
#1773=CARTESIAN_POINT ( 'NONE',  ( 74.59884440882045453, 37.32890624999999574, 9.598844408820456309 ) ) ;
#1776=CARTESIAN_POINT ( 'NONE',  ( 96.46446609406721961, 81.25000000273119838, 3.535533905932727539 ) ) ;
#1777=CARTESIAN_POINT ( 'NONE',  ( 139.5988444088204687, 34.25312500216787015, 9.598844408820456309 ) ) ;
#1778=CARTESIAN_POINT ( 'NONE',  ( 55.70494972787295751, 40.65273437608393436, -9.295050272127046043 ) ) ;
#1780=CARTESIAN_POINT ( 'NONE',  ( 204.2950502721270425, 37.27929687608394005, -9.295050272127046043 ) ) ;
#1781=VERTEX_POINT ( 'NONE', #8007 ) ;
#1782=ORIENTED_EDGE ( 'NONE', *, *, #17385, .T. ) ;
#1785=CARTESIAN_POINT ( 'NONE',  ( 2.493653234604083739E-15, 38.02343749999999289, 13.57481594606304576 ) ) ;
#1786=CARTESIAN_POINT ( 'NONE',  ( 101.8468681455907046, 84.12500000136560629, -4.458734125000016313 ) ) ;
#1787=DIRECTION ( 'NONE',  ( -1.000000000000000000, 0.000000000000000000, 2.385244779468110248E-16 ) ) ;
#1788=EDGE_CURVE ( 'NONE', #12549, #24077, #12551, .T. ) ;
#1790=VECTOR ( 'NONE', #15167, 1000.000000000000000 ) ;
#1792=COLOUR_RGB ( '', 0.09019608, 0.27058824, 0.51372549) ;
#1793=CARTESIAN_POINT ( 'NONE',  ( 97.92893218813452449, 82.81250000000001421, -5.000000000000043521 ) ) ;
#1794=CARTESIAN_POINT ( 'NONE',  ( 116.4251840539369454, 32.21914062500000142, -5.622872871577873077 ) ) ;
#1795=ORIENTED_EDGE ( 'NONE', *, *, #9386, .F. ) ;
#1799=CARTESIAN_POINT ( 'NONE',  ( 139.2950502721270425, 36.48554687608393721, -9.295050272127046043 ) ) ;
#1800=CARTESIAN_POINT ( 'NONE',  ( 70.44491438647230552, 36.83281250108392868, 13.14518615778179189 ) ) ;
#1801=CARTESIAN_POINT ( 'NONE',  ( 181.8548138422181921, 39.11484375108394573, -5.444914386472297529 ) ) ;
#1803=CARTESIAN_POINT ( 'NONE',  ( 5.444914386472302859, 36.03906250108394005, 13.14518615778179189 ) ) ;
#1804=FACE_OUTER_BOUND ( 'NONE', #3387, .T. ) ;
#1806=CARTESIAN_POINT ( 'NONE',  ( 99.99999999999995737, 82.25000000000000000, 4.999999999999990230 ) ) ;
#1807=ORIENTED_EDGE ( 'NONE', *, *, #16489, .F. ) ;
#1808=CARTESIAN_POINT ( 'NONE',  ( -5.444914386472299306, 39.11484375108394573, 13.14518615778179722 ) ) ;
#1814=EDGE_CURVE ( 'NONE', #4816, #9474, #1416, .T. ) ;
#1822=CARTESIAN_POINT ( 'NONE',  ( 65.00000000000000000, 37.72578125216787726, -13.57481594606304576 ) ) ;
#1823=CARTESIAN_POINT ( 'NONE',  ( 95.54126587499996504, 84.68750000136560629, -1.387778780781445676E-14 ) ) ;
#1824=CARTESIAN_POINT ( 'NONE',  ( 55.70494972787295751, 39.85898437608393152, -9.295050272127046043 ) ) ;
#1826=CARTESIAN_POINT ( 'NONE',  ( 13.14518615778179722, 40.10703125108393152, 5.444914386472293977 ) ) ;
#1828=ORIENTED_EDGE ( 'NONE', *, *, #13179, .F. ) ;
#1831=CARTESIAN_POINT ( 'NONE',  ( 143.5748159460630688, 39.01562500000000000, -1.662435489736055892E-15 ) ) ;
#1833=CARTESIAN_POINT ( 'NONE',  ( 120.4011555911795455, 40.30546874999999574, 9.598844408820459861 ) ) ;
#1835=CARTESIAN_POINT ( 'NONE',  ( -0.3247243111960383954, 53.49346745874647979, -15.00000000000000533 ) ) ;
#1839=CARTESIAN_POINT ( 'NONE',  ( 116.8548138422182063, 39.71015625108393010, -5.444914386472297529 ) ) ;
#1840=CARTESIAN_POINT ( 'NONE',  ( 51.42518405393695957, 37.97382812716787726, 5.622872871577880183 ) ) ;
#1843=CARTESIAN_POINT ( 'NONE',  ( 13.57481594606304931, 35.09648437716787583, 5.622872871577869525 ) ) ;
#1844=ORIENTED_EDGE ( 'NONE', *, *, #3092, .T. ) ;
#1848=CARTESIAN_POINT ( 'NONE',  ( 208.1451861577818079, 37.77539062608393294, -1.609821015232357215E-15 ) ) ;
#1850=CARTESIAN_POINT ( 'NONE',  ( 120.7049497278729575, 37.27929687608393294, -9.295050272127046043 ) ) ;
#1855=CARTESIAN_POINT ( 'NONE',  ( 181.4251840539369596, 36.23749999999999005, 0.000000000000000000 ) ) ;
#1856=EDGE_CURVE ( 'NONE', #24599, #1420, #20434, .T. ) ;
#1860=CARTESIAN_POINT ( 'NONE',  ( 51.85481384221819923, 38.12265625108393152, -5.444914386472297529 ) ) ;
#1865=CARTESIAN_POINT ( 'NONE',  ( 5.622872871577878406, 38.07304687499998863, 13.57481594606304576 ) ) ;
#1868=CARTESIAN_POINT ( 'NONE',  ( 95.54126587499996504, 83.68750000136560629, -1.387778780781445676E-14 ) ) ;
#1872=( BOUNDED_CURVE ( )  B_SPLINE_CURVE ( 2, ( #24453, #20324, #14172, #14029, #9479, #27179, #22466, #4939, #7481 ),
 .UNSPECIFIED., .F., .F. ) 
 B_SPLINE_CURVE_WITH_KNOTS ( ( 3, 2, 2, 2, 3 ),
 ( 0.2708333333333330928, 0.2812499999999998890, 0.2916666666666666852, 0.3020833333333334259, 0.3125000000000002220 ),
 .UNSPECIFIED. ) 
 CURVE ( )  GEOMETRIC_REPRESENTATION_ITEM ( )  RATIONAL_B_SPLINE_CURVE ( ( 1.000000000000001554, 0.9238795325112850731, 1.000000000000000000, 0.9238795325112867385, 1.000000000000000000, 0.9238795325112867385, 1.000000000000000000, 0.9238795325112850731, 1.000000000000001554 ) ) 
 REPRESENTATION_ITEM ( '' )  );
#1874=CARTESIAN_POINT ( 'NONE',  ( 74.29505027212704249, 34.69960937608393436, 9.295050272127046043 ) ) ;
#1880=CARTESIAN_POINT ( 'NONE',  ( 99.99999999999995737, 82.37500000273119838, 4.999999999999990230 ) ) ;
#1882=CARTESIAN_POINT ( 'NONE',  ( 181.4251840539369596, 36.38632812716788578, 5.622872871577880183 ) ) ;
#1884=CARTESIAN_POINT ( 'NONE',  ( 70.62287287157801074, 36.08867187716787583, -13.57481594606290898 ) ) ;
#1886=CARTESIAN_POINT ( 'NONE',  ( 143.1451861577818363, 40.30546875108393579, 5.444914386472293977 ) ) ;
#1887=CARTESIAN_POINT ( 'NONE',  ( -13.14518615778179189, 37.62656250108393863, 5.444914386472304635 ) ) ;
#1890=CARTESIAN_POINT ( 'NONE',  ( 65.00000000000000000, 38.81718749999999574, 13.57481594606304576 ) ) ;
#1896=CARTESIAN_POINT ( 'NONE',  ( 95.54126587499996504, 80.62500000136559208, -1.846868145590750077 ) ) ;
#1898=CARTESIAN_POINT ( 'NONE',  ( -5.444914386472299306, 38.51953125108393294, 13.14518615778179722 ) ) ;
#1899=EDGE_CURVE ( 'NONE', #27401, #26813, #6301, .T. ) ;
#1901=ORIENTED_EDGE ( 'NONE', *, *, #9674, .T. ) ;
#1902=FACE_OUTER_BOUND ( 'NONE', #14942, .T. ) ;
#1905=CARTESIAN_POINT ( 'NONE',  ( -5.622872871577947684, 40.05742187499998863, -13.57481594606297293 ) ) ;
#1907=CARTESIAN_POINT ( 'NONE',  ( 181.8548138422182205, 38.17226562608393436, 0.000000000000000000 ) ) ;
#1909=VERTEX_POINT ( 'NONE', #12689 ) ;
#1910=CARTESIAN_POINT ( 'NONE',  ( 52.31840720293882185, 36.04503594658365984, 5.908507747192915716 ) ) ;
#1913=ORIENTED_EDGE ( 'NONE', *, *, #9353, .T. ) ;
#1915=CARTESIAN_POINT ( 'NONE',  ( -8.395938741299726615, 54.99999999495823033, -15.00000000000000000 ) ) ;
#1917=CARTESIAN_POINT ( 'NONE',  ( 130.0000000000000000, 36.13828125216787157, -13.57481594606304576 ) ) ;
#1918=CARTESIAN_POINT ( 'NONE',  ( 181.4251840539369596, 40.99999999999999289, 0.000000000000000000 ) ) ;
#1920=CARTESIAN_POINT ( 'NONE',  ( 204.2950502721270425, 34.69960937608393436, 9.295050272127046043 ) ) ;
#1925=CARTESIAN_POINT ( 'NONE',  ( 74.29505027212704249, 39.26367187608393294, 9.295050272127046043 ) ) ;
#1926=CARTESIAN_POINT ( 'NONE',  ( 98.15313185440923860, 80.25000000136559208, -4.458734125000016313 ) ) ;
#1927=CARTESIAN_POINT ( 'NONE',  ( 70.62287287157788285, 39.75976562716787299, 13.57481594606306174 ) ) ;
#1930=DIRECTION ( 'NONE',  ( -0.000000000000000000, 1.000000000000000000, -0.000000000000000000 ) ) ;
#1931=CARTESIAN_POINT ( 'NONE',  ( 185.7049497278729575, 39.85898437608393152, -9.295050272127046043 ) ) ;
#1937=CARTESIAN_POINT ( 'NONE',  ( 135.4449143864723055, 35.74140625108393721, -13.14518615778179900 ) ) ;
#1938=CARTESIAN_POINT ( 'NONE',  ( 51.85481384221820633, 36.58476562608393579, 0.000000000000000000 ) ) ;
#1939=CARTESIAN_POINT ( 'NONE',  ( 181.8548138422181921, 40.00781250108393294, 5.444914386472304635 ) ) ;
#1940=DIRECTION ( 'NONE',  ( -0.000000000000000000, -1.000000000000000000, -0.000000000000000000 ) ) ;
#1941=CARTESIAN_POINT ( 'NONE',  ( -13.14518615778179189, 35.04687500108393294, 5.444914386472304635 ) ) ;
#1942=CARTESIAN_POINT ( 'NONE',  ( 124.6762090360452504, 54.47170356488336296, -14.99999999999999645 ) ) ;
#1943=LINE ( 'NONE', #2081, #9860 ) ;
#1944=CARTESIAN_POINT ( 'NONE',  ( 94.99999999999995737, 82.00000000000000000, -1.387778780781445676E-14 ) ) ;
#1946=CARTESIAN_POINT ( 'NONE',  ( -9.295050272127044266, 39.85898437608393152, 9.295050272127047819 ) ) ;
#1947=CARTESIAN_POINT ( 'NONE',  ( 9.180175813647995398, 55.00000000000000000, 14.99999999999999467 ) ) ;
#1956=AXIS2_PLACEMENT_3D ( 'NONE', #3228, #16186, #13751 ) ;
#1958=CARTESIAN_POINT ( 'NONE',  ( 99.99999999999995737, 85.00000000000000000, -1.387778780781445676E-14 ) ) ;
#1959=CARTESIAN_POINT ( 'NONE',  ( 98.15313185440925281, 83.50000000136560629, -4.458734125000016313 ) ) ;
#1960=CARTESIAN_POINT ( 'NONE',  ( 51.85481384221819923, 38.32109375108394289, -5.444914386472297529 ) ) ;
#1962=CARTESIAN_POINT ( 'NONE',  ( 2.414731522848535132E-15, 39.95820312608393010, 13.14518615778179544 ) ) ;
#1967=CARTESIAN_POINT ( 'NONE',  ( 135.6228728715778686, 40.75195312500000711, -13.57481594606304753 ) ) ;
#1971=CARTESIAN_POINT ( 'NONE',  ( 104.4587341249999781, 79.87500000136559208, 1.846868145590721655 ) ) ;
#1972=CARTESIAN_POINT ( 'NONE',  ( 135.4449143864723055, 36.33671875108394289, -13.14518615778179900 ) ) ;
#1973=CARTESIAN_POINT ( 'NONE',  ( 55.40115559117954547, 37.82500000216787583, -9.598844408820458085 ) ) ;
#1975=CARTESIAN_POINT ( 'NONE',  ( -8.312177448680279460E-16, 35.34453125216787583, -13.57481594606304576 ) ) ;
#1976=AXIS2_PLACEMENT_3D ( 'NONE', #26715, #492, #16144 ) ;
#1979=CARTESIAN_POINT ( 'NONE',  ( 189.5550856135277229, 36.73359375108393010, 13.14518615778179722 ) ) ;
#1980=CARTESIAN_POINT ( 'NONE',  ( 74.59884440882045453, 39.11484374999999858, -9.598844408820458085 ) ) ;
#1981=CARTESIAN_POINT ( 'NONE',  ( 120.7049497278729575, 38.07304687608393579, -9.295050272127046043 ) ) ;
#1982=CARTESIAN_POINT ( 'NONE',  ( 185.4011555911795597, 38.02343750216788010, 9.598844408820459861 ) ) ;
#1983=ADVANCED_FACE ( 'NONE', ( #14968 ), #6432, .T. ) ;
#1985=CARTESIAN_POINT ( 'NONE',  ( 195.0000000000000000, 36.43593749999999432, 13.57481594606304576 ) ) ;
#1986=CARTESIAN_POINT ( 'NONE',  ( 214.9999999999999716, 80.00000000000000000, -10.00000000000000000 ) ) ;
#1990=CARTESIAN_POINT ( 'NONE',  ( 208.5748159460630120, 38.17226562499999432, 5.622872871577869525 ) ) ;
#1993=CARTESIAN_POINT ( 'NONE',  ( 59.55508561352770158, 39.90859375108393436, 13.14518615778179722 ) ) ;
#1998=CARTESIAN_POINT ( 'NONE',  ( 13.57481594606304576, 39.01562500000000000, -1.662435489736055892E-15 ) ) ;
#1999=LINE ( 'NONE', #19096, #21722 ) ;
#2001=CARTESIAN_POINT ( 'NONE',  ( 103.5355339059327093, 83.62500000000000000, -3.535533905932755072 ) ) ;
#2002=VECTOR ( 'NONE', #11775, 1000.000000000000000 ) ;
#2005=CARTESIAN_POINT ( 'NONE',  ( 74.29505027212704249, 35.49335937608393721, 9.295050272127046043 ) ) ;
#2007=CARTESIAN_POINT ( 'NONE',  ( -8.312177448680279460E-16, 36.83281249999999574, -13.57481594606304576 ) ) ;
#2009=ORIENTED_EDGE ( 'NONE', *, *, #16296, .F. ) ;
#2010=CARTESIAN_POINT ( 'NONE',  ( 96.46446609406721961, 82.25000000273119838, 3.535533905932727539 ) ) ;
#2012=CARTESIAN_POINT ( 'NONE',  ( 204.5988444088204687, 37.42812500216787441, 9.598844408820456309 ) ) ;
#2017=CARTESIAN_POINT ( 'NONE',  ( 143.1451861577818363, 40.40468750108393436, -5.444914386472297529 ) ) ;
#2018=CARTESIAN_POINT ( 'NONE',  ( -13.14518615778179900, 37.52734375108393294, -5.444914386472297529 ) ) ;
#2019=CARTESIAN_POINT ( 'NONE',  ( 130.0000000000000000, 34.79882812608393294, -13.14518615778179544 ) ) ;
#2020=CARTESIAN_POINT ( 'NONE',  ( 51.42518405393695957, 37.03124999999999289, 0.000000000000000000 ) ) ;
#2037=LINE ( 'NONE', #1761, #7534 ) ;
#2040=CARTESIAN_POINT ( 'NONE',  ( 181.8548138422181921, 38.12265625108393152, -5.444914386472297529 ) ) ;
#2041=ORIENTED_EDGE ( 'NONE', *, *, #24047, .F. ) ;
#2044=CARTESIAN_POINT ( 'NONE',  ( 57.38347467451918504, 54.91574374957784954, -14.99999999999999822 ) ) ;
#2045=VERTEX_POINT ( 'NONE', #10416 ) ;
#2049=CARTESIAN_POINT ( 'NONE',  ( 94.99999999999995737, 81.06250000273119838, -2.071067811865491493 ) ) ;
#2050=CARTESIAN_POINT ( 'NONE',  ( 143.5748159460630404, 33.50898437716787015, 5.622872871577869525 ) ) ;
#2051=CARTESIAN_POINT ( 'NONE',  ( 55.70494972787295751, 39.85898437608393152, -9.295050272127046043 ) ) ;
#2052=LINE ( 'NONE', #21864, #24111 ) ;
#2053=EDGE_CURVE ( 'NONE', #16548, #16918, #28122, .T. ) ;
#2054=CARTESIAN_POINT ( 'NONE',  ( 208.1451861577817795, 33.95546875108393436, 5.444914386472293977 ) ) ;
#2055=EDGE_LOOP ( 'NONE', ( #9944, #7722, #18909, #19495 ) ) ;
#2060=CARTESIAN_POINT ( 'NONE',  ( 78.14518615778179367, 40.15664062608393436, -1.609821015232357215E-15 ) ) ;
#2061=CARTESIAN_POINT ( 'NONE',  ( 96.84719886470459471, 80.56250000136559208, 3.152801135295355994 ) ) ;
#2062=CARTESIAN_POINT ( 'NONE',  ( 181.8548138422182205, 37.32890625108393579, -5.444914386472297529 ) ) ;
#2066=CARTESIAN_POINT ( 'NONE',  ( 78.57481594606305464, 39.75976562499999289, 5.622872871577868636 ) ) ;
#2071=CIRCLE ( 'NONE', #5730, 5.000000000000000000 ) ;
#2072=CIRCLE ( 'NONE', #4825, 13.57481594606304398 ) ;
#2074=CARTESIAN_POINT ( 'NONE',  ( 143.1451861577818079, 35.59257812608393579, -1.609821015232357215E-15 ) ) ;
#2075=CARTESIAN_POINT ( 'NONE',  ( 55.70494972787295751, 33.31054687608393294, -9.295050272127046043 ) ) ;
#2076=CARTESIAN_POINT ( 'NONE',  ( 189.5550856135277229, 36.93203125108394147, 13.14518615778179722 ) ) ;
#2079=CARTESIAN_POINT ( 'NONE',  ( -5.444914386472297529, 36.43593750108392726, -13.14518615778179900 ) ) ;
#2080=CARTESIAN_POINT ( 'NONE',  ( 136.1177599455525069, 54.65941425415165611, -14.99999999999999645 ) ) ;
#2081=CARTESIAN_POINT ( 'NONE',  ( 130.0000000000000000, -7.395377635281828788, 13.57481594606302799 ) ) ;
#2084=CARTESIAN_POINT ( 'NONE',  ( 5.444914386472297529, 37.92421875108392726, -13.14518615778179900 ) ) ;
#2087=CARTESIAN_POINT ( 'NONE',  ( 58.09762142622420811, 51.13402819306927682, 15.00000000000063238 ) ) ;
#2093=CARTESIAN_POINT ( 'NONE',  ( 123.8389378251455639, 51.27996893916988341, 14.99999999999790745 ) ) ;
#2095=CARTESIAN_POINT ( 'NONE',  ( 130.0000000000000000, 38.91640625216786731, 13.57481594606304576 ) ) ;
#2096=CARTESIAN_POINT ( 'NONE',  ( 95.54126587499995082, 81.62500000136560629, -1.846868145590750077 ) ) ;
#2097=CARTESIAN_POINT ( 'NONE',  ( 78.14518615778179367, 35.54296875108394715, 5.444914386472293977 ) ) ;
#2099=CARTESIAN_POINT ( 'NONE',  ( -9.295050272127044266, 39.85898437608393152, 9.295050272127047819 ) ) ;
#2100=VERTEX_POINT ( 'NONE', #11255 ) ;
#2104=CARTESIAN_POINT ( 'NONE',  ( 135.6228728715778971, 39.66054687500000142, 13.57481594606304576 ) ) ;
#2105=VERTEX_POINT ( 'NONE', #22397 ) ;
#2106=DIRECTION ( 'NONE',  ( -0.000000000000000000, 1.000000000000000000, -0.000000000000000000 ) ) ;
#2107=ADVANCED_FACE ( 'NONE', ( #4727 ), #7272, .T. ) ;
#2110=CARTESIAN_POINT ( 'NONE',  ( 124.5550856135277087, 35.14609375108393152, 13.14518615778179722 ) ) ;
#2111=CARTESIAN_POINT ( 'NONE',  ( 55.40115559117954547, 35.44375000216787441, -9.598844408820458085 ) ) ;
#2112=B_SPLINE_CURVE_WITH_KNOTS ( 'NONE', 3,
 ( #27313, #27033, #24738, #16025, #20471, #7629, #26744, #15884, #14171, #3498, #7479, #16321, #5361, #950, #9477, #9621, #1234, #22889, #26890, #11745, #12026, #7186, #20750, #5219, #12161, #9337, #16174, #14027, #7336, #809, #9897 ),
 .UNSPECIFIED., .F., .F.,
 ( 4, 2, 2, 2, 2, 2, 2, 2, 2, 2, 1, 2, 2, 2, 2, 4 ),
 ( 0.000000000000000000, 0.001656255954913781435, 0.003312511909827562870, 0.004968767864741344305, 0.005796895842198234589, 0.006625023819655125740, 0.008281279774568908042, 0.009937535729482686875, 0.01325004763931025148, 0.01490630359422403031, 0.01656255954913780915, 0.01821881550405159145, 0.01987507145896537028, 0.02318758336879293835, 0.02484383932370672066, 0.02650009527862050296 ),
 .UNSPECIFIED. ) ;
#2113=CARTESIAN_POINT ( 'NONE',  ( 9.598844408820456309, 36.03906250216787299, -9.598844408820458085 ) ) ;
#2117=CARTESIAN_POINT ( 'NONE',  ( 208.1451861577817795, 38.61875000108393152, -5.444914386472297529 ) ) ;
#2119=CARTESIAN_POINT ( 'NONE',  ( 102.0710678118653618, 81.31250000000000000, 5.000000000000031086 ) ) ;
#2121=DIRECTION ( 'NONE',  ( -1.000000000000000000, 8.275480229788910625E-32, 2.385244779468109755E-16 ) ) ;
#2126=VECTOR ( 'NONE', #11389, 1000.000000000000000 ) ;
#2129=CARTESIAN_POINT ( 'NONE',  ( 185.4011555911795597, 34.74921874999999716, 9.598844408820459861 ) ) ;
#2130=B_SPLINE_CURVE_WITH_KNOTS ( 'NONE', 3,
 ( #24885, #11465, #4941, #2933, #22891, #20045, #20184, #9482, #9341, #26893, #24741, #11887, #20612, #13887, #1096, #9763, #22613, #7631, #16325, #26749, #25024, #5506, #7191, #3083, #14174 ),
 .UNSPECIFIED., .F., .F.,
 ( 4, 2, 2, 2, 2, 2, 2, 1, 2, 2, 2, 2, 4 ),
 ( 0.000000000000000000, 0.001301161269048799630, 0.002602322538097599260, 0.005204645076195198519, 0.007806967614292798646, 0.01040929015239039704, 0.01171045142143919970, 0.01301161269048800063, 0.01431277395953680330, 0.01561393522858560597, 0.01821625776668320262, 0.01951741903573200529, 0.02081858030478080449 ),
 .UNSPECIFIED. ) ;
#2132=CARTESIAN_POINT ( 'NONE',  ( 195.0000000000000000, -7.395377635281828788, -13.57481594606306707 ) ) ;
#2133=CARTESIAN_POINT ( 'NONE',  ( 70.44491438647230552, 37.13046875108393152, -13.14518615778179900 ) ) ;
#2139=CARTESIAN_POINT ( 'NONE',  ( -9.598844408820454532, 35.54296874999999289, 9.598844408820459861 ) ) ;
#2142=ORIENTED_EDGE ( 'NONE', *, *, #10358, .T. ) ;
#2143=CARTESIAN_POINT ( 'NONE',  ( 94.99999999999995737, 85.00000000000000000, -1.387778780781445676E-14 ) ) ;
#2144=ADVANCED_FACE ( 'NONE', ( #17970 ), #17688, .T. ) ;
#2146=ORIENTED_EDGE ( 'NONE', *, *, #10490, .T. ) ;
#2148=CARTESIAN_POINT ( 'NONE',  ( 74.29505027212704249, 36.28710937608393294, 9.295050272127046043 ) ) ;
#2156=CARTESIAN_POINT ( 'NONE',  ( 195.0000000000000000, 37.72578125216787726, -13.57481594606304576 ) ) ;
#2159=CARTESIAN_POINT ( 'NONE',  ( 191.1360747348882398, 54.10645156200111927, 14.99999999999995026 ) ) ;
#2160=CARTESIAN_POINT ( 'NONE',  ( 143.1451861577818363, 36.33671875108393579, 5.444914386472293977 ) ) ;
#2161=CARTESIAN_POINT ( 'NONE',  ( -5.444914386472299306, 37.72578125108395142, 13.14518615778179722 ) ) ;
#2162=CARTESIAN_POINT ( 'NONE',  ( 116.8548138422182063, 33.36015625108393579, -5.444914386472297529 ) ) ;
#2163=CARTESIAN_POINT ( 'NONE',  ( 51.42518405393695957, 33.11210937499999574, 5.622872871577880183 ) ) ;
#2167=ADVANCED_FACE ( 'NONE', ( #453 ), #4873, .F. ) ;
#2171=AXIS2_PLACEMENT_3D ( 'NONE', #12525, #14541, #6274 ) ;
#2172=CARTESIAN_POINT ( 'NONE',  ( 104.4587341249999639, 80.18750000136559208, -1.442382525525748735E-14 ) ) ;
#2174=CARTESIAN_POINT ( 'NONE',  ( -13.14518615778179189, 37.62656250108393863, 5.444914386472304635 ) ) ;
#2176=ORIENTED_EDGE ( 'NONE', *, *, #19611, .T. ) ;
#2179=ADVANCED_FACE ( 'NONE', ( #2450 ), #15683, .T. ) ;
#2180=CARTESIAN_POINT ( 'NONE',  ( 189.3771271284220745, 36.08867187500000284, -13.57481594606300135 ) ) ;
#2182=CARTESIAN_POINT ( 'NONE',  ( 181.8548138422181921, 40.50390625108394005, -5.444914386472297529 ) ) ;
#2183=VERTEX_POINT ( 'NONE', #8850 ) ;
#2185=EDGE_CURVE ( 'NONE', #540, #11153, #11537, .T. ) ;
#2186=CYLINDRICAL_SURFACE ( 'NONE', #13412, 4.999999999999999112 ) ;
#2188=ORIENTED_EDGE ( 'NONE', *, *, #7577, .F. ) ;
#2193=CARTESIAN_POINT ( 'NONE',  ( 143.1451861577818079, 39.41250000108393436, -5.444914386472297529 ) ) ;
#2196=CARTESIAN_POINT ( 'NONE',  ( 74.29505027212704249, 40.25585937608393294, 9.295050272127046043 ) ) ;
#2198=CARTESIAN_POINT ( 'NONE',  ( 181.8548138422182205, 34.40195312608393152, 0.000000000000000000 ) ) ;
#2200=( BOUNDED_CURVE ( )  B_SPLINE_CURVE ( 2, ( #2881, #18127, #19840, #468, #22129, #24400, #9013, #5168, #10985 ),
 .UNSPECIFIED., .F., .T. ) 
 B_SPLINE_CURVE_WITH_KNOTS ( ( 3, 2, 2, 2, 3 ),
 ( 0.02083333333333358892, 0.03125000000000020123, 0.04166666666666681007, 0.05208333333333342585, 0.06250000000000004163 ),
 .UNSPECIFIED. ) 
 CURVE ( )  GEOMETRIC_REPRESENTATION_ITEM ( )  RATIONAL_B_SPLINE_CURVE ( ( 0.9999999999999981126, 0.9238795325112886259, 1.000000000000000000, 0.9238795325112867385, 1.000000000000000000, 0.9238795325112867385, 1.000000000000000000, 0.9238795325112864054, 1.000000000000000222 ) ) 
 REPRESENTATION_ITEM ( '' )  );
#2204=CARTESIAN_POINT ( 'NONE',  ( 59.55508561352770158, 39.11484375108393863, 13.14518615778179722 ) ) ;
#2206=CARTESIAN_POINT ( 'NONE',  ( 104.4587341249999781, 82.87500000136560629, 1.846868145590721655 ) ) ;
#2207=CARTESIAN_POINT ( 'NONE',  ( 195.0000000000000000, 37.57695312608392868, 13.14518615778179544 ) ) ;
#2211=DIRECTION ( 'NONE',  ( -0.000000000000000000, 1.000000000000000000, -0.000000000000000000 ) ) ;
#2214=VERTEX_POINT ( 'NONE', #20117 ) ;
#2215=EDGE_CURVE ( 'NONE', #21433, #24113, #15951, .T. ) ;
#2219=CARTESIAN_POINT ( 'NONE',  ( 116.8548138422182205, 35.19570312608393436, 0.000000000000000000 ) ) ;
#2220=CARTESIAN_POINT ( 'NONE',  ( 78.14518615778179367, 34.60039062608392868, -1.609821015232357215E-15 ) ) ;
#2222=CARTESIAN_POINT ( 'NONE',  ( 185.7049497278729575, 36.68398437608393436, -9.295050272127046043 ) ) ;
#2225=CARTESIAN_POINT ( 'NONE',  ( 139.1801758136479918, 50.00000000000002132, -15.00000000000000000 ) ) ;
#2226=CARTESIAN_POINT ( 'NONE',  ( 188.6617095634187251, 36.00000000000002132, 11.53991937534743784 ) ) ;
#2227=FACE_OUTER_BOUND ( 'NONE', #10725, .T. ) ;
#2229=CARTESIAN_POINT ( 'NONE',  ( 13.14518615778179900, 36.93203125108394147, 5.444914386472293977 ) ) ;
#2230=EDGE_CURVE ( 'NONE', #4960, #27535, #2323, .T. ) ;
#2232=FACE_OUTER_BOUND ( 'NONE', #7500, .T. ) ;
#2234=CARTESIAN_POINT ( 'NONE',  ( 58.54912065733758197, 50.00000000106957998, 11.97362904075674983 ) ) ;
#2240=CARTESIAN_POINT ( 'NONE',  ( 130.3286002765670446, 53.49358765999040344, 14.99999999999996447 ) ) ;
#2242=DIRECTION ( 'NONE',  ( 0.000000000000000000, 0.000000000000000000, -1.000000000000000000 ) ) ;
#2243=CARTESIAN_POINT ( 'NONE',  ( 104.4587341249999781, 81.12500000136559208, 1.846868145590721655 ) ) ;
#2244=CARTESIAN_POINT ( 'NONE',  ( 70.44491438647230552, 34.94765625108394147, -13.14518615778179900 ) ) ;
#2251=CARTESIAN_POINT ( 'NONE',  ( 139.5988444088204687, 38.91640624999999432, 9.598844408820456309 ) ) ;
#2252=ADVANCED_FACE ( 'NONE', ( #16108 ), #20826, .T. ) ;
#2257=CARTESIAN_POINT ( 'NONE',  ( 116.8548138422182205, 35.79101562608393294, 0.000000000000000000 ) ) ;
#2258=CARTESIAN_POINT ( 'NONE',  ( 65.00000000000000000, 33.36015625216786873, 13.57481594606304576 ) ) ;
#2261=STYLED_ITEM ( 'NONE', ( #5076 ), #2892 ) ;
#2262=CARTESIAN_POINT ( 'NONE',  ( 7.171391395016640580, 31.30502190640808990, -11.52591746582321974 ) ) ;
#2263=AXIS2_PLACEMENT_3D ( 'NONE', #26535, #15966, #13820 ) ;
#2266=CARTESIAN_POINT ( 'NONE',  ( 208.1451861577817795, 34.65000000108393152, -5.444914386472297529 ) ) ;
#2267=DIRECTION ( 'NONE',  ( -0.000000000000000000, 1.000000000000000000, -0.000000000000000000 ) ) ;
#2268=CARTESIAN_POINT ( 'NONE',  ( 104.9999999999999716, 81.50000000000000000, -1.449011120738813565E-14 ) ) ;
#2271=CARTESIAN_POINT ( 'NONE',  ( 200.6228728715778118, 39.26367187716788010, -13.57481594606312036 ) ) ;
#2276=CARTESIAN_POINT ( 'NONE',  ( 208.5748159460630120, 33.50898437499999716, -5.622872871577873077 ) ) ;
#2279=CARTESIAN_POINT ( 'NONE',  ( 70.44491438647230552, 35.54296875108393294, -13.14518615778179900 ) ) ;
#2280=DIRECTION ( 'NONE',  ( 0.000000000000000000, 0.000000000000000000, 1.000000000000000000 ) ) ;
#2284=CARTESIAN_POINT ( 'NONE',  ( 5.622872871577871301, 35.19570312499999432, -13.57481594606304753 ) ) ;
#2285=CARTESIAN_POINT ( 'NONE',  ( 143.1451861577818079, 37.18007812608393436, -1.609821015232357215E-15 ) ) ;
#2288=CARTESIAN_POINT ( 'NONE',  ( 104.9999999999999574, 84.56250000000002842, -2.071067811865491937 ) ) ;
#2289=CARTESIAN_POINT ( 'NONE',  ( 97.92893218813451028, 83.93750000273119838, -5.000000000000018652 ) ) ;
#2292=ORIENTED_EDGE ( 'NONE', *, *, #20278, .F. ) ;
#2294=CARTESIAN_POINT ( 'NONE',  ( 59.55508561352770158, 34.25312500108393010, -13.14518615778179900 ) ) ;
#2295=ORIENTED_EDGE ( 'NONE', *, *, #13803, .F. ) ;
#2296=CARTESIAN_POINT ( 'NONE',  ( 135.6228728715777834, 39.26367187716788010, -13.57481594606312036 ) ) ;
#2298=ORIENTED_EDGE ( 'NONE', *, *, #2382, .T. ) ;
#2301=CARTESIAN_POINT ( 'NONE',  ( 185.4011555911795597, 38.02343750216788010, 9.598844408820459861 ) ) ;
#2303=LINE ( 'NONE', #26090, #17632 ) ;
#2304=DIRECTION ( 'NONE',  ( -0.000000000000000000, 1.000000000000000000, -0.000000000000000000 ) ) ;
#2305=ORIENTED_EDGE ( 'NONE', *, *, #5823, .F. ) ;
#2306=CARTESIAN_POINT ( 'NONE',  ( -9.295050272127046043, 39.85898437608393152, -9.295050272127046043 ) ) ;
#2307=AXIS2_PLACEMENT_3D ( 'NONE', #10384, #15073, #23791 ) ;
#2309=CARTESIAN_POINT ( 'NONE',  ( 130.0000000000000000, 35.59257812608393579, -13.14518615778179544 ) ) ;
#2310=CARTESIAN_POINT ( 'NONE',  ( 74.59884440882045453, 35.93984374999999432, -9.598844408820458085 ) ) ;
#2319=CARTESIAN_POINT ( 'NONE',  ( -13.14518615778179189, 36.83281250108393579, 5.444914386472304635 ) ) ;
#2321=ORIENTED_EDGE ( 'NONE', *, *, #2520, .T. ) ;
#2323=( BOUNDED_CURVE ( )  B_SPLINE_CURVE ( 2, ( #169, #6703, #15391, #24103, #4581, #13241, #18816, #24677, #16541 ),
 .UNSPECIFIED., .F., .F. ) 
 B_SPLINE_CURVE_WITH_KNOTS ( ( 3, 2, 2, 2, 3 ),
 ( 0.3958333333333331483, 0.4062499999999999445, 0.4166666666666667407, 0.4270833333333335369, 0.4375000000000003331 ),
 .UNSPECIFIED. ) 
 CURVE ( )  GEOMETRIC_REPRESENTATION_ITEM ( )  RATIONAL_B_SPLINE_CURVE ( ( 1.000000000000001110, 0.9238795325112855172, 1.000000000000000000, 0.9238795325112867385, 1.000000000000000000, 0.9238795325112867385, 1.000000000000000000, 0.9238795325112842960, 1.000000000000002442 ) ) 
 REPRESENTATION_ITEM ( '' )  );
#2324=DIRECTION ( 'NONE',  ( -0.000000000000000000, 1.000000000000000000, -0.000000000000000000 ) ) ;
#2325=CARTESIAN_POINT ( 'NONE',  ( 219.9999999999999716, 80.00000000000000000, -10.00000000000000178 ) ) ;
#2326=CARTESIAN_POINT ( 'NONE',  ( 208.1451861577817795, 38.51953125108393294, 5.444914386472293977 ) ) ;
#2328=CARTESIAN_POINT ( 'NONE',  ( 74.29505027212704249, 36.48554687608393721, -9.295050272127046043 ) ) ;
#2329=CARTESIAN_POINT ( 'NONE',  ( 191.2025481310419366, 54.08938259242988522, -15.00000000000000000 ) ) ;
#2330=VERTEX_POINT ( 'NONE', #888 ) ;
#2333=CARTESIAN_POINT ( 'NONE',  ( 94.99999999999995737, 81.12500000273119838, -1.387778780781445676E-14 ) ) ;
#2334=CARTESIAN_POINT ( 'NONE',  ( 139.2950502721270425, 40.25585937608393294, -9.295050272127046043 ) ) ;
#2335=CARTESIAN_POINT ( 'NONE',  ( -8.049105076161786076E-16, 39.75976562608394005, -13.14518615778179544 ) ) ;
#2337=CARTESIAN_POINT ( 'NONE',  ( 65.00000000000000000, 38.96601562608393721, -13.14518615778179544 ) ) ;
#2340=CARTESIAN_POINT ( 'NONE',  ( 195.0000000000000000, 34.99726562608393721, -13.14518615778179544 ) ) ;
#2344=VERTEX_POINT ( 'NONE', #13960 ) ;
#2349=CARTESIAN_POINT ( 'NONE',  ( 104.4587341249999781, 81.00000000136560629, -1.846868145590750521 ) ) ;
#2350=CARTESIAN_POINT ( 'NONE',  ( 195.0000000000000000, 39.95820312608393010, 13.14518615778179544 ) ) ;
#2352=FACE_OUTER_BOUND ( 'NONE', #19097, .T. ) ;
#2353=CARTESIAN_POINT ( 'NONE',  ( 65.00000000000000000, -7.395377635281828788, 13.57481594606303688 ) ) ;
#2354=CARTESIAN_POINT ( 'NONE',  ( 181.8548138422182205, 40.70234375108392300, -5.444914386472297529 ) ) ;
#2356=EDGE_CURVE ( 'NONE', #25435, #8206, #11967, .T. ) ;
#2361=CARTESIAN_POINT ( 'NONE',  ( 130.0000000000000000, 37.77539062608393294, 13.14518615778179544 ) ) ;
#2362=CARTESIAN_POINT ( 'NONE',  ( 59.55508561352770158, 34.84843750108393579, -13.14518615778179900 ) ) ;
#2363=CARTESIAN_POINT ( 'NONE',  ( 181.8548138422181921, 35.93984375108393436, -5.444914386472297529 ) ) ;
#2364=ORIENTED_EDGE ( 'NONE', *, *, #3092, .F. ) ;
#2366=CARTESIAN_POINT ( 'NONE',  ( -8.049105076161786076E-16, 33.21132812608393436, -13.14518615778179544 ) ) ;
#2367=CARTESIAN_POINT ( 'NONE',  ( 131.9473259220810064, 51.47162402671692405, -15.00000000000066258 ) ) ;
#2369=CARTESIAN_POINT ( 'NONE',  ( 139.5988444088204403, 40.00781250216787299, -9.598844408820458085 ) ) ;
#2374=CARTESIAN_POINT ( 'NONE',  ( 74.18017581364799184, 55.00000000000000000, 14.99999999999997868 ) ) ;
#2375=CARTESIAN_POINT ( 'NONE',  ( 58.83893782516223325, 51.27996893917264032, 14.99999999999997868 ) ) ;
#2381=CARTESIAN_POINT ( 'NONE',  ( 130.9830651851037260, 49.99999999949027796, 13.54930971656715677 ) ) ;
#2382=EDGE_CURVE ( 'NONE', #4458, #28041, #4313, .T. ) ;
#2385=CARTESIAN_POINT ( 'NONE',  ( 101.8468681455906903, 81.37500000136563472, -4.458734125000016313 ) ) ;
#2386=CARTESIAN_POINT ( 'NONE',  ( 78.14518615778179367, 34.84843750108393579, -5.444914386472297529 ) ) ;
#2388=CARTESIAN_POINT ( 'NONE',  ( 9.295050272127046043, 37.87460937608393152, -9.295050272127046043 ) ) ;
#2389=DIRECTION ( 'NONE',  ( 0.000000000000000000, 1.000000000000000000, 0.000000000000000000 ) ) ;
#2392=CARTESIAN_POINT ( 'NONE',  ( 124.3771271284221314, 36.08867187500000284, -13.57481594606304753 ) ) ;
#2393=ADVANCED_FACE ( 'NONE', ( #1446 ), #10279, .T. ) ;
#2398=CARTESIAN_POINT ( 'NONE',  ( 143.1451861577818079, 37.72578125108393721, 5.444914386472293977 ) ) ;
#2400=CARTESIAN_POINT ( 'NONE',  ( 78.57481594606304043, 35.09648437716787583, 5.622872871577869525 ) ) ;
#2402=CARTESIAN_POINT ( 'NONE',  ( -9.295050272127046043, 40.45429687608393721, -9.295050272127046043 ) ) ;
#2405=CARTESIAN_POINT ( 'NONE',  ( 189.5550856135277229, 33.26093750108393721, -13.14518615778179900 ) ) ;
#2409=DIRECTION ( 'NONE',  ( -1.000000000000000000, 0.000000000000000000, -3.469446951953613696E-16 ) ) ;
#2412=DIRECTION ( 'NONE',  ( -0.8660254037844418162, -0.4999999999999947264, -0.000000000000000000 ) ) ;
#2414=LINE ( 'NONE', #11497, #21638 ) ;
#2417=CARTESIAN_POINT ( 'NONE',  ( 189.3771271284221314, 35.29492187500000000, -13.57481594606304753 ) ) ;
#2420=CARTESIAN_POINT ( 'NONE',  ( 139.5988444088204687, 36.53515624999999289, 9.598844408820456309 ) ) ;
#2421=CARTESIAN_POINT ( 'NONE',  ( 70.44491438647230552, 33.95546875108393436, -13.14518615778179900 ) ) ;
#2425=CARTESIAN_POINT ( 'NONE',  ( 9.598844408820456309, 37.52734375000000000, -9.598844408820458085 ) ) ;
#2426=CARTESIAN_POINT ( 'NONE',  ( 116.8548138422182063, 39.21406250108392300, 5.444914386472304635 ) ) ;
#2428=CARTESIAN_POINT ( 'NONE',  ( 104.9999999999999716, 82.50000000000000000, -1.449011120738813565E-14 ) ) ;
#2429=CARTESIAN_POINT ( 'NONE',  ( 99.99999999999995737, 81.87500000273119838, -5.000000000000018652 ) ) ;
#2431=CARTESIAN_POINT ( 'NONE',  ( 52.14049004392254005, 36.00000000000001421, -3.245221471867175023 ) ) ;
#2434=CARTESIAN_POINT ( 'NONE',  ( 51.42518405393695957, 40.99999999999999289, 0.000000000000000000 ) ) ;
#2435=VERTEX_POINT ( 'NONE', #20752 ) ;
#2438=VERTEX_POINT ( 'NONE', #9900 ) ;
#2441=CARTESIAN_POINT ( 'NONE',  ( 204.5988444088204403, 36.03906250216787299, -9.598844408820458085 ) ) ;
#2443=LINE ( 'NONE', #24236, #2126 ) ;
#2444=CARTESIAN_POINT ( 'NONE',  ( 214.9999999999999716, 75.00000000000000000, -10.00000000000000000 ) ) ;
#2445=CARTESIAN_POINT ( 'NONE',  ( -5.444914386472299306, 35.34453125108393579, 13.14518615778179722 ) ) ;
#2446=CARTESIAN_POINT ( 'NONE',  ( 139.2950502721270425, 34.69960937608393436, -9.295050272127046043 ) ) ;
#2447=CARTESIAN_POINT ( 'NONE',  ( 78.57481594606305464, 33.45937499999999432, -1.662435489736055892E-15 ) ) ;
#2448=FACE_OUTER_BOUND ( 'NONE', #24937, .T. ) ;
#2450=FACE_OUTER_BOUND ( 'NONE', #14400, .T. ) ;
#2455=CARTESIAN_POINT ( 'NONE',  ( 2.414731522848535132E-15, 35.39414062608393863, 13.14518615778179544 ) ) ;
#2457=EDGE_LOOP ( 'NONE', ( #17288, #711, #27032 ) ) ;
#2461=EDGE_CURVE ( 'NONE', #9259, #27424, #23781, .T. ) ;
#2462=CARTESIAN_POINT ( 'NONE',  ( 208.1451861577817795, 37.82500000108392868, -5.444914386472297529 ) ) ;
#2463=ORIENTED_EDGE ( 'NONE', *, *, #27785, .F. ) ;
#2465=CARTESIAN_POINT ( 'NONE',  ( 203.7726092461557812, 50.37415326817817629, -14.99999999999999822 ) ) ;
#2471=CARTESIAN_POINT ( 'NONE',  ( 139.2950502721270425, 40.05742187608392868, 9.295050272127046043 ) ) ;
#2474=CARTESIAN_POINT ( 'NONE',  ( 74.29505027212704249, 38.07304687608393579, -9.295050272127046043 ) ) ;
#2476=CARTESIAN_POINT ( 'NONE',  ( 200.4449143864723055, 36.23750000108393721, 13.14518615778179189 ) ) ;
#2478=ORIENTED_EDGE ( 'NONE', *, *, #24239, .T. ) ;
#2483=CARTESIAN_POINT ( 'NONE',  ( 65.00000000000000000, 39.95820312608393010, 13.14518615778179544 ) ) ;
#2484=CARTESIAN_POINT ( 'NONE',  ( 96.84719886470459471, 79.56250000136559208, 3.152801135295355994 ) ) ;
#2485=CARTESIAN_POINT ( 'NONE',  ( 185.7049497278729575, 40.45429687608393721, -9.295050272127046043 ) ) ;
#2489=CARTESIAN_POINT ( 'NONE',  ( 78.57481594606305464, 39.80937499999999574, -1.662435489736055892E-15 ) ) ;
#2491=ORIENTED_EDGE ( 'NONE', *, *, #25266, .F. ) ;
#2492=ORIENTED_EDGE ( 'NONE', *, *, #12484, .F. ) ;
#2496=CARTESIAN_POINT ( 'NONE',  ( 120.7049497278729575, 32.11992187608393579, 9.295050272127047819 ) ) ;
#2497=CARTESIAN_POINT ( 'NONE',  ( 59.55508561352770158, 35.14609375108393152, 13.14518615778179722 ) ) ;
#2498=CARTESIAN_POINT ( 'NONE',  ( 200.4449143864723055, 36.23750000108393721, 13.14518615778179189 ) ) ;
#2499=ADVANCED_FACE ( 'NONE', ( #11466 ), #20185, .T. ) ;
#2502=CARTESIAN_POINT ( 'NONE',  ( 9.295050272127047819, 32.11992187608393579, 9.295050272127046043 ) ) ;
#2503=CARTESIAN_POINT ( 'NONE',  ( 129.6030005853479850, 51.45716825712189291, -15.00000000000033573 ) ) ;
#2506=CARTESIAN_POINT ( 'NONE',  ( 199.1572863549628210, 35.99999999999999289, -12.92256159328821141 ) ) ;
#2512=EDGE_LOOP ( 'NONE', ( #26472, #17277, #3650, #10533 ) ) ;
#2515=CARTESIAN_POINT ( 'NONE',  ( 124.6345034319466691, 54.48174559708144926, 14.99999999999996803 ) ) ;
#2518=CARTESIAN_POINT ( 'NONE',  ( 104.4587341249999781, 82.25000000136559208, -1.846868145590750299 ) ) ;
#2519=CARTESIAN_POINT ( 'NONE',  ( 51.85481384221820633, 35.24531250108393721, 5.444914386472304635 ) ) ;
#2520=EDGE_CURVE ( 'NONE', #2344, #26363, #3502, .T. ) ;
#2522=CARTESIAN_POINT ( 'NONE',  ( 2.414731522848535132E-15, 39.16445312608392726, 13.14518615778179544 ) ) ;
#2524=LINE ( 'NONE', #241, #1328 ) ;
#2525=CARTESIAN_POINT ( 'NONE',  ( 99.99999999999995737, 82.25000000000000000, 4.999999999999990230 ) ) ;
#2526=CARTESIAN_POINT ( 'NONE',  ( 120.4011555911795455, 37.92421874999999432, 9.598844408820459861 ) ) ;
#2528=ORIENTED_EDGE ( 'NONE', *, *, #17246, .T. ) ;
#2533=CARTESIAN_POINT ( 'NONE',  ( 120.7049497278729575, 35.69179687608393436, -9.295050272127046043 ) ) ;
#2535=CARTESIAN_POINT ( 'NONE',  ( 51.42518405393695957, 33.95546875216787441, 0.000000000000000000 ) ) ;
#2539=AXIS2_PLACEMENT_3D ( 'NONE', #8020, #8434, #3890 ) ;
#2541=CARTESIAN_POINT ( 'NONE',  ( -5.622872871577873077, 33.01289062716787726, -13.57481594606304753 ) ) ;
#2542=EDGE_CURVE ( 'NONE', #9045, #28041, #7908, .T. ) ;
#2545=CARTESIAN_POINT ( 'NONE',  ( 189.5550856135277229, 34.84843750108393579, -13.14518615778179900 ) ) ;
#2556=CARTESIAN_POINT ( 'NONE',  ( 185.4011555911795313, 33.75703124999999005, -9.598844408820458085 ) ) ;
#2559=CARTESIAN_POINT ( 'NONE',  ( 65.00000000000000000, 35.19570312608392726, 13.14518615778179544 ) ) ;
#2563=CARTESIAN_POINT ( 'NONE',  ( -5.622872871577873077, 36.08867187500000284, -13.57481594606304753 ) ) ;
#2564=CARTESIAN_POINT ( 'NONE',  ( 139.2950502721270425, 38.86679687608393863, -9.295050272127046043 ) ) ;
#2565=EDGE_CURVE ( 'NONE', #15436, #20385, #18866, .T. ) ;
#2566=EDGE_LOOP ( 'NONE', ( #21580, #13791, #18482, #26653 ) ) ;
#2567=CARTESIAN_POINT ( 'NONE',  ( 104.9999999999999716, 84.50000000000000000, -1.449011120738813565E-14 ) ) ;
#2569=CARTESIAN_POINT ( 'NONE',  ( 96.46446609406721961, 84.00000000273119838, -3.535533905932755072 ) ) ;
#2570=AXIS2_PLACEMENT_3D ( 'NONE', #21626, #19619, #4236 ) ;
#2572=CARTESIAN_POINT ( 'NONE',  ( 60.02711226049118665, 36.00000000000001421, -12.48139679469878871 ) ) ;
#2573=EDGE_CURVE ( 'NONE', #3340, #28009, #14451, .T. ) ;
#2575=CARTESIAN_POINT ( 'NONE',  ( 78.14518615778179367, 33.21132812608393436, -1.609821015232357215E-15 ) ) ;
#2578=CYLINDRICAL_SURFACE ( 'NONE', #19038, 5.000000000000004441 ) ;
#2583=CARTESIAN_POINT ( 'NONE',  ( 185.4011555911795597, 33.26093750216787726, 9.598844408820459861 ) ) ;
#2586=CARTESIAN_POINT ( 'NONE',  ( 55.81982418635200816, 55.00000000000000000, -14.99999999999999822 ) ) ;
#2587=CARTESIAN_POINT ( 'NONE',  ( 204.5988444088204403, 38.42031250216787441, -9.598844408820458085 ) ) ;
#2588=CARTESIAN_POINT ( 'NONE',  ( 5.444914386472302859, 36.23750000108393721, 13.14518615778179189 ) ) ;
#2589=CARTESIAN_POINT ( 'NONE',  ( 143.1451861577818079, 36.23750000108393010, -5.444914386472297529 ) ) ;
#2590=CARTESIAN_POINT ( 'NONE',  ( 55.40115559117954547, 35.54296874999999289, 9.598844408820459861 ) ) ;
#2591=AXIS2_PLACEMENT_3D ( 'NONE', #24762, #11485, #17780 ) ;
#2594=CARTESIAN_POINT ( 'NONE',  ( 195.0000000000000000, -7.395377635281828788, -2.255140518769849538E-14 ) ) ;
#2598=DIRECTION ( 'NONE',  ( 0.000000000000000000, -1.000000000000000000, 0.000000000000000000 ) ) ;
#2600=CARTESIAN_POINT ( 'NONE',  ( 9.295050272127047819, 36.28710937608393294, 9.295050272127046043 ) ) ;
#2602=ORIENTED_EDGE ( 'NONE', *, *, #1788, .F. ) ;
#2605=DIRECTION ( 'NONE',  ( -0.8660254037844418162, 0.4999999999999947264, 0.000000000000000000 ) ) ;
#2606=CARTESIAN_POINT ( 'NONE',  ( 181.8548138422181921, 37.32890625108393579, -5.444914386472297529 ) ) ;
#2608=CARTESIAN_POINT ( 'NONE',  ( 195.8421075954646255, 53.50112910130381749, -15.00000000000000178 ) ) ;
#2614=CARTESIAN_POINT ( 'NONE',  ( 124.3771271284221314, 32.51679687716787726, 13.57481594606304753 ) ) ;
#2615=CARTESIAN_POINT ( 'NONE',  ( -9.295050272127046043, 39.85898437608393152, -9.295050272127046043 ) ) ;
#2618=CARTESIAN_POINT ( 'NONE',  ( 59.55508561352770158, 37.72578125108395142, 13.14518615778179722 ) ) ;
#2619=CARTESIAN_POINT ( 'NONE',  ( 68.86392526511711765, 54.10645156200380512, -15.00000000000000000 ) ) ;
#2620=CARTESIAN_POINT ( 'NONE',  ( 200.6228728715778686, 40.75195312500000711, -13.57481594606304753 ) ) ;
#2622=CARTESIAN_POINT ( 'NONE',  ( 74.59884440882045453, 38.32109374999999574, -9.598844408820458085 ) ) ;
#2624=ORIENTED_EDGE ( 'NONE', *, *, #15897, .T. ) ;
#2628=CARTESIAN_POINT ( 'NONE',  ( 55.70494972787295751, 38.86679687608393863, -9.295050272127046043 ) ) ;
#2630=CARTESIAN_POINT ( 'NONE',  ( 204.2950502721270425, 37.67617187608393436, 9.295050272127046043 ) ) ;
#2634=CARTESIAN_POINT ( 'NONE',  ( 200.4449143864723055, 38.12265625108393863, -13.14518615778179722 ) ) ;
#2636=ORIENTED_EDGE ( 'NONE', *, *, #16630, .F. ) ;
#2640=CARTESIAN_POINT ( 'NONE',  ( 120.7049497278729575, 32.71523437608393436, -9.295050272127046043 ) ) ;
#2641=CARTESIAN_POINT ( 'NONE',  ( 78.14518615778179367, 33.06250000108393294, -5.444914386472297529 ) ) ;
#2642=CARTESIAN_POINT ( 'NONE',  ( 195.0000000000000000, 36.98164062608393721, 13.14518615778179544 ) ) ;
#2643=ORIENTED_EDGE ( 'NONE', *, *, #479, .T. ) ;
#2645=CARTESIAN_POINT ( 'NONE',  ( 9.295050272127047819, 33.70742187608393436, 9.295050272127046043 ) ) ;
#2647=CARTESIAN_POINT ( 'NONE',  ( 120.4011555911795455, 39.41250000216787441, -9.598844408820458085 ) ) ;
#2651=CARTESIAN_POINT ( 'NONE',  ( 71.87350824357694989, 51.14166184781134206, 15.00000000000195222 ) ) ;
#2656=ORIENTED_EDGE ( 'NONE', *, *, #84, .F. ) ;
#2659=CARTESIAN_POINT ( 'NONE',  ( 51.42518405393695957, 37.87460937716787868, -5.622872871577872189 ) ) ;
#2662=CARTESIAN_POINT ( 'NONE',  ( -13.57481594606304576, 38.71796875216787726, 0.000000000000000000 ) ) ;
#2663=CARTESIAN_POINT ( 'NONE',  ( 101.8468681455906903, 81.00000000136560629, 4.458734124999987891 ) ) ;
#2664=CARTESIAN_POINT ( 'NONE',  ( 51.85481384221819923, 35.93984375108393436, -5.444914386472297529 ) ) ;
#2666=CARTESIAN_POINT ( 'NONE',  ( -13.14518615778179189, 38.22187500108393721, 5.444914386472304635 ) ) ;
#2667=CARTESIAN_POINT ( 'NONE',  ( -13.57481594606304576, 37.87460937499999147, 5.622872871577880183 ) ) ;
#2668=CARTESIAN_POINT ( 'NONE',  ( 6.119843627700378264, 51.28708186914656153, 14.99999999999999645 ) ) ;
#2670=CARTESIAN_POINT ( 'NONE',  ( 130.0000000000000000, 38.42031249999999432, -13.57481594606304576 ) ) ;
#2673=DIRECTION ( 'NONE',  ( 0.000000000000000000, 0.000000000000000000, -1.000000000000000000 ) ) ;
#2677=CARTESIAN_POINT ( 'NONE',  ( 116.8548138422182205, 34.99726562608393721, 0.000000000000000000 ) ) ;
#2678=CARTESIAN_POINT ( 'NONE',  ( 78.57481594606304043, 33.50898437716787015, 5.622872871577869525 ) ) ;
#2679=CARTESIAN_POINT ( 'NONE',  ( -13.57481594606304753, 31.52460937716787370, -5.622872871577873077 ) ) ;
#2680=CIRCLE ( 'NONE', #16323, 11.57481594606304398 ) ;
#2686=CARTESIAN_POINT ( 'NONE',  ( 208.1451861577818079, 33.01289062608393010, -1.609821015232357215E-15 ) ) ;
#2687=DIRECTION ( 'NONE',  ( -0.000000000000000000, 1.000000000000000000, -0.000000000000000000 ) ) ;
#2689=CARTESIAN_POINT ( 'NONE',  ( 130.0000000000000000, 39.31328125216787583, -13.57481594606304576 ) ) ;
#2697=CARTESIAN_POINT ( 'NONE',  ( 200.6228728715778686, 34.89804687499999147, 13.57481594606304576 ) ) ;
#2700=CARTESIAN_POINT ( 'NONE',  ( 143.5748159460630688, 36.68398437500000142, -5.622872871577873966 ) ) ;
#2701=CARTESIAN_POINT ( 'NONE',  ( 70.44491438647230552, 36.33671875108394289, -13.14518615778179900 ) ) ;
#2706=DIRECTION ( 'NONE',  ( -0.000000000000000000, 1.000000000000000000, -0.000000000000000000 ) ) ;
#2707=CARTESIAN_POINT ( 'NONE',  ( -13.57481594606304576, 36.23749999999999005, 0.000000000000000000 ) ) ;
#2708=CARTESIAN_POINT ( 'NONE',  ( 143.1451861577818079, 37.92421875108392726, 5.444914386472293977 ) ) ;
#2712=CARTESIAN_POINT ( 'NONE',  ( 103.5355339059327093, 82.75000000273119838, -3.535533905932755072 ) ) ;
#2715=CARTESIAN_POINT ( 'NONE',  ( 60.54052658636183537, 35.99999999999998579, -12.68347323196786292 ) ) ;
#2716=EDGE_CURVE ( 'NONE', #17777, #16548, #13009, .T. ) ;
#2718=CARTESIAN_POINT ( 'NONE',  ( 51.85481384221819923, 32.76484375108393010, -5.444914386472297529 ) ) ;
#2724=CARTESIAN_POINT ( 'NONE',  ( 181.4251840539369596, 33.16171875216787868, 0.000000000000000000 ) ) ;
#2727=CARTESIAN_POINT ( 'NONE',  ( 204.5988444088204403, 40.00781250216787299, -9.598844408820458085 ) ) ;
#2728=CARTESIAN_POINT ( 'NONE',  ( 9.295050272127047819, 34.69960937608393436, 9.295050272127046043 ) ) ;
#2729=CARTESIAN_POINT ( 'NONE',  ( 143.1451861577818079, 32.96328125108393436, 5.444914386472293977 ) ) ;
#2730=CARTESIAN_POINT ( 'NONE',  ( 74.59884440882045453, 34.94765624999999432, 9.598844408820456309 ) ) ;
#2731=DIRECTION ( 'NONE',  ( -0.000000000000000000, 1.000000000000000000, -0.000000000000000000 ) ) ;
#2736=DIRECTION ( 'NONE',  ( 0.000000000000000000, 0.000000000000000000, 1.000000000000000000 ) ) ;
#2739=CARTESIAN_POINT ( 'NONE',  ( -8.049105076161786076E-16, 36.58476562608393579, -13.14518615778179544 ) ) ;
#2740=EDGE_CURVE ( 'NONE', #21141, #21949, #922, .T. ) ;
#2744=( BOUNDED_CURVE ( )  B_SPLINE_CURVE ( 2, ( #4644, #19740, #13302 ),
 .UNSPECIFIED., .F., .F. ) 
 B_SPLINE_CURVE_WITH_KNOTS ( ( 3, 3 ),
 ( 0.5208333333333332593, 0.5249747582430959181 ),
 .UNSPECIFIED. ) 
 CURVE ( )  GEOMETRIC_REPRESENTATION_ITEM ( )  RATIONAL_B_SPLINE_CURVE ( ( 1.000000000000000888, 0.9697362687807495885, 0.9635368518655813563 ) ) 
 REPRESENTATION_ITEM ( '' )  );
#2747=CARTESIAN_POINT ( 'NONE',  ( 208.1451861577817795, 34.55078125108393294, 5.444914386472293977 ) ) ;
#2748=ORIENTED_EDGE ( 'NONE', *, *, #26047, .F. ) ;
#2749=CARTESIAN_POINT ( 'NONE',  ( 191.9606029491974084, 53.88964894337311762, -15.00000000000000000 ) ) ;
#2756=CARTESIAN_POINT ( 'NONE',  ( 120.4011555911795455, 31.67343750216787512, 9.598844408820459861 ) ) ;
#2758=CARTESIAN_POINT ( 'NONE',  ( -13.14518615778179189, 35.04687500108393294, 5.444914386472304635 ) ) ;
#2759=CIRCLE ( 'NONE', #9135, 11.57481594606304398 ) ;
#2761=CARTESIAN_POINT ( 'NONE',  ( 59.55508561352770158, 38.51953125108393294, 13.14518615778179722 ) ) ;
#2762=CARTESIAN_POINT ( 'NONE',  ( 58.58713332374817639, 50.00000000108478559, -11.99502265407751267 ) ) ;
#2764=CARTESIAN_POINT ( 'NONE',  ( 185.7049497278729575, 32.11992187608393579, 9.295050272127047819 ) ) ;
#2765=CARTESIAN_POINT ( 'NONE',  ( 72.75412397599441761, 36.00000000000002842, 10.77549638133779553 ) ) ;
#2768=CARTESIAN_POINT ( 'NONE',  ( 65.00000000000000000, 36.38632812608393152, -13.14518615778179544 ) ) ;
#2769=FACE_OUTER_BOUND ( 'NONE', #17556, .T. ) ;
#2771=ORIENTED_EDGE ( 'NONE', *, *, #3331, .T. ) ;
#2774=CARTESIAN_POINT ( 'NONE',  ( 208.1451861577818079, 37.92421875108393436, 5.444914386472293977 ) ) ;
#2776=ORIENTED_EDGE ( 'NONE', *, *, #18913, .T. ) ;
#2779=ORIENTED_EDGE ( 'NONE', *, *, #19455, .T. ) ;
#2780=CARTESIAN_POINT ( 'NONE',  ( 143.1451861577818079, 34.74921875108395142, 5.444914386472293977 ) ) ;
#2781=CARTESIAN_POINT ( 'NONE',  ( 51.85481384221820633, 40.75195312608393294, 0.000000000000000000 ) ) ;
#2782=CARTESIAN_POINT ( 'NONE',  ( 200.4449143864723055, 35.44375000108393436, 13.14518615778179189 ) ) ;
#2787=AXIS2_PLACEMENT_3D ( 'NONE', #5811, #14482, #23199 ) ;
#2791=CARTESIAN_POINT ( 'NONE',  ( 68.04460945692940754, 53.89089363584395898, 14.99999999999997868 ) ) ;
#2793=VERTEX_POINT ( 'NONE', #18442 ) ;
#2799=CARTESIAN_POINT ( 'NONE',  ( 65.00000000000000000, 37.32890625216786873, 13.57481594606304576 ) ) ;
#2801=CARTESIAN_POINT ( 'NONE',  ( 181.4251840539369596, 37.87460937499999147, 5.622872871577880183 ) ) ;
#2802=CARTESIAN_POINT ( 'NONE',  ( -5.444914386472297529, 37.22968750108394431, -13.14518615778179722 ) ) ;
#2806=CARTESIAN_POINT ( 'NONE',  ( 120.4011555911795455, 36.13828124999999147, -9.598844408820458085 ) ) ;
#2812=CARTESIAN_POINT ( 'NONE',  ( 143.1451861577818079, 33.06250000108393294, -5.444914386472297529 ) ) ;
#2813=CARTESIAN_POINT ( 'NONE',  ( 55.70494972787295751, 39.85898437608393152, 9.295050272127047819 ) ) ;
#2815=CARTESIAN_POINT ( 'NONE',  ( 104.9999999999999716, 80.43750000000002842, 2.071067811865462627 ) ) ;
#2816=CARTESIAN_POINT ( 'NONE',  ( -8.312177448680279460E-16, 32.96328125216787441, -13.57481594606304576 ) ) ;
#2820=CARTESIAN_POINT ( 'NONE',  ( 195.0000000000000000, 34.79882812608393294, -13.14518615778179544 ) ) ;
#2824=CARTESIAN_POINT ( 'NONE',  ( 204.5988444088204403, 39.11484374999999858, -9.598844408820458085 ) ) ;
#2827=CARTESIAN_POINT ( 'NONE',  ( 99.99999999999995737, 85.00000000000000000, 2.999999999999990674 ) ) ;
#2829=DIRECTION ( 'NONE',  ( -1.040834085586084848E-15, 1.000000000000000000, 0.000000000000000000 ) ) ;
#2832=CARTESIAN_POINT ( 'NONE',  ( 185.4011555911795597, 32.36796874999999574, 9.598844408820459861 ) ) ;
#2835=CARTESIAN_POINT ( 'NONE',  ( 98.15313185440925281, 84.25000000136559208, -4.458734125000016313 ) ) ;
#2836=CARTESIAN_POINT ( 'NONE',  ( 51.85481384221820633, 35.04687500108393294, 5.444914386472304635 ) ) ;
#2840=CARTESIAN_POINT ( 'NONE',  ( 13.57481594606304931, 33.40976562499999858, 5.622872871577869525 ) ) ;
#2841=CARTESIAN_POINT ( 'NONE',  ( 130.0000000000000000, 38.56914062608393579, 13.14518615778179544 ) ) ;
#2842=VERTEX_POINT ( 'NONE', #26571 ) ;
#2843=CARTESIAN_POINT ( 'NONE',  ( 94.99999999999995737, 82.00000000000000000, -1.387778780781445676E-14 ) ) ;
#2844=CARTESIAN_POINT ( 'NONE',  ( 78.57481594606305464, 38.32109375216786873, -1.662435489736055892E-15 ) ) ;
#2845=CARTESIAN_POINT ( 'NONE',  ( 97.92893218813451028, 79.93750000273119838, -5.000000000000018652 ) ) ;
#2849=CARTESIAN_POINT ( 'NONE',  ( 51.42518405393695957, 40.25585937499999289, 5.622872871577880183 ) ) ;
#2852=AXIS2_PLACEMENT_3D ( 'NONE', #23754, #6637, #24035 ) ;
#2854=EDGE_CURVE ( 'NONE', #19811, #10089, #8507, .T. ) ;
#2855=ORIENTED_EDGE ( 'NONE', *, *, #27287, .F. ) ;
#2857=CARTESIAN_POINT ( 'NONE',  ( 200.6228728715778686, 34.50117187716788436, -13.57481594606304753 ) ) ;
#2861=CARTESIAN_POINT ( 'NONE',  ( -13.14518615778179900, 35.14609375108393152, -5.444914386472297529 ) ) ;
#2862=CARTESIAN_POINT ( 'NONE',  ( 124.5550856135277087, 32.46718750108393436, -13.14518615778179900 ) ) ;
#2866=CARTESIAN_POINT ( 'NONE',  ( 208.2454503467689904, 36.00000000000000711, 2.307131236160025800 ) ) ;
#2869=CYLINDRICAL_SURFACE ( 'NONE', #20474, 13.57481594606304398 ) ;
#2870=CARTESIAN_POINT ( 'NONE',  ( 99.99999999999995737, 78.00000000000000000, -1.387778780781445676E-14 ) ) ;
#2872=CARTESIAN_POINT ( 'NONE',  ( -13.14518615778179189, 33.65781250108393152, 5.444914386472304635 ) ) ;
#2874=ORIENTED_EDGE ( 'NONE', *, *, #16651, .F. ) ;
#2876=CARTESIAN_POINT ( 'NONE',  ( 195.0000000000000000, 52.00000000000000711, -11.57481594606306707 ) ) ;
#2877=DIRECTION ( 'NONE',  ( -0.000000000000000000, -1.000000000000000000, -0.000000000000000000 ) ) ;
#2878=CARTESIAN_POINT ( 'NONE',  ( 185.7049497278729575, 34.89804687608393152, -9.295050272127046043 ) ) ;
#2881=CARTESIAN_POINT ( 'NONE',  ( -8.312177448680279460E-16, 40.10703125216787157, -13.57481594606304576 ) ) ;
#2883=ORIENTED_EDGE ( 'NONE', *, *, #3607, .T. ) ;
#2888=B_SPLINE_CURVE_WITH_KNOTS ( 'NONE', 3,
 ( #12183, #9645, #11770, #22776, #11911, #1117, #978, #25178, #12045, #5666, #23050, #3524, #25877, #19319, #2226, #3940, #17314, #8624, #19178, #6214, #14607, #23741, #25592, #10325, #8342 ),
 .UNSPECIFIED., .F., .F.,
 ( 4, 2, 2, 2, 2, 2, 2, 1, 2, 2, 2, 2, 4 ),
 ( 0.000000000000000000, 0.001301161269048876174, 0.002602322538097752349, 0.005204645076195502963, 0.007806967614293254878, 0.01040929015239100593, 0.01171045142143988319, 0.01301161269048875871, 0.01431277395953763597, 0.01561393522858651149, 0.01821625776668426427, 0.01951741903573314327, 0.02081858030478202226 ),
 .UNSPECIFIED. ) ;
#2889=CARTESIAN_POINT ( 'NONE',  ( 116.8548138422182063, 37.42812500108393436, 5.444914386472304635 ) ) ;
#2890=CARTESIAN_POINT ( 'NONE',  ( 5.444914386472297529, 36.53515625108394715, -13.14518615778179722 ) ) ;
#2891=CARTESIAN_POINT ( 'NONE',  ( 13.14518615778179900, 34.55078125108393294, 5.444914386472293977 ) ) ;
#2892=ADVANCED_BREP_SHAPE_REPRESENTATION ( '', ( #7448, #26844 ), #12238 ) ;
#2894=CARTESIAN_POINT ( 'NONE',  ( 69.57159163252556766, 51.44262710532576932, -14.99999999999933742 ) ) ;
#2896=CARTESIAN_POINT ( 'NONE',  ( 181.4251840539369596, 40.15664062500000142, -5.622872871577873077 ) ) ;
#2897=EDGE_CURVE ( 'NONE', #2435, #24292, #1999, .T. ) ;
#2902=CARTESIAN_POINT ( 'NONE',  ( 55.70494972787295751, 37.27929687608393294, -9.295050272127046043 ) ) ;
#2908=CARTESIAN_POINT ( 'NONE',  ( 195.0000000000000000, 37.77539062608393294, 13.14518615778179544 ) ) ;
#2914=CARTESIAN_POINT ( 'NONE',  ( 116.8548138422182063, 32.76484375108393010, -5.444914386472297529 ) ) ;
#2916=CARTESIAN_POINT ( 'NONE',  ( 204.2950502721270425, 33.90585937608393863, 9.295050272127046043 ) ) ;
#2919=CARTESIAN_POINT ( 'NONE',  ( 7.636241067997081799, 54.91786508990981019, -14.99999999999999822 ) ) ;
#2922=CARTESIAN_POINT ( 'NONE',  ( 130.0000000000000000, 36.93203125216787441, -13.57481594606304576 ) ) ;
#2925=CARTESIAN_POINT ( 'NONE',  ( 65.98306518510102592, 49.99999999949029217, 13.54930971656748717 ) ) ;
#2928=VERTEX_POINT ( 'NONE', #28203 ) ;
#2931=CARTESIAN_POINT ( 'NONE',  ( 135.3237909639547070, 54.47170356488064868, 14.99999999999996447 ) ) ;
#2933=CARTESIAN_POINT ( 'NONE',  ( -12.83975123685818964, 35.99999999999999289, 2.850296047819762535 ) ) ;
#2934=CARTESIAN_POINT ( 'NONE',  ( 51.85481384221820633, 32.81445312608393294, 0.000000000000000000 ) ) ;
#2936=CARTESIAN_POINT ( 'NONE',  ( 5.444914386472297529, 37.13046875108393152, -13.14518615778179722 ) ) ;
#2939=CARTESIAN_POINT ( 'NONE',  ( 0.4460412567804681316, 49.99999999978076204, 13.57776691409236314 ) ) ;
#2941=CARTESIAN_POINT ( 'NONE',  ( 130.0000000000000000, 33.65781249999999147, -13.57481594606304576 ) ) ;
#2944=( BOUNDED_CURVE ( )  B_SPLINE_CURVE ( 2, ( #19603, #28164, #8631, #26018, #26158, #23883, #15311, #24026, #21900 ),
 .UNSPECIFIED., .F., .F. ) 
 B_SPLINE_CURVE_WITH_KNOTS ( ( 3, 2, 2, 2, 3 ),
 ( 0.8500000000000007550, 0.8750000000000008882, 0.9000000000000009104, 0.9250000000000009326, 0.9500000000000009548 ),
 .UNSPECIFIED. ) 
 CURVE ( )  GEOMETRIC_REPRESENTATION_ITEM ( )  RATIONAL_B_SPLINE_CURVE ( ( 0.9999999999999976685, 0.9238795325112890700, 1.000000000000000000, 0.9238795325112867385, 1.000000000000000000, 0.9238795325112867385, 1.000000000000000000, 0.9238795325112837409, 1.000000000000003109 ) ) 
 REPRESENTATION_ITEM ( '' )  );
#2948=CARTESIAN_POINT ( 'NONE',  ( 130.0000000000000000, 34.79882812608393294, -13.14518615778179544 ) ) ;
#2949=CARTESIAN_POINT ( 'NONE',  ( 72.17139139501665568, 31.30502190640808990, -11.52591746582321974 ) ) ;
#2950=CARTESIAN_POINT ( 'NONE',  ( 65.00000000000000000, 36.93203125216787441, -13.57481594606304576 ) ) ;
#2951=CARTESIAN_POINT ( 'NONE',  ( 9.295050272127047819, 37.67617187608393436, 9.295050272127046043 ) ) ;
#2952=DIRECTION ( 'NONE',  ( 0.000000000000000000, 0.000000000000000000, 1.000000000000000000 ) ) ;
#2956=DIRECTION ( 'NONE',  ( 0.000000000000000000, 0.000000000000000000, -1.000000000000000000 ) ) ;
#2959=CARTESIAN_POINT ( 'NONE',  ( 195.0000000000000000, 40.00781250000000000, -13.57481594606304576 ) ) ;
#2969=CARTESIAN_POINT ( 'NONE',  ( 103.1528011352953342, 82.06250000136559208, -3.152801135295383084 ) ) ;
#2970=CARTESIAN_POINT ( 'NONE',  ( 74.29505027212704249, 33.70742187608393436, 9.295050272127046043 ) ) ;
#2973=CARTESIAN_POINT ( 'NONE',  ( -8.312177448680279460E-16, 40.00781250000000000, -13.57481594606304576 ) ) ;
#2975=CARTESIAN_POINT ( 'NONE',  ( 5.622872871577946796, 37.27929687499999289, 13.57481594606297115 ) ) ;
#2976=CARTESIAN_POINT ( 'NONE',  ( -13.57481594606304753, 32.21914062500000142, -5.622872871577873077 ) ) ;
#2977=CARTESIAN_POINT ( 'NONE',  ( 139.2950502721270425, 33.31054687608394005, -9.295050272127046043 ) ) ;
#2978=ORIENTED_EDGE ( 'NONE', *, *, #14429, .F. ) ;
#2979=CARTESIAN_POINT ( 'NONE',  ( 103.5355339059327093, 82.37500000000000000, 3.535533905932726206 ) ) ;
#2982=CARTESIAN_POINT ( 'NONE',  ( 96.46446609406721961, 79.25000000273118417, 3.535533905932727539 ) ) ;
#2987=CARTESIAN_POINT ( 'NONE',  ( 51.42518405393695957, 40.20624999999999005, 0.000000000000000000 ) ) ;
#2988=CARTESIAN_POINT ( 'NONE',  ( 13.57481594606304931, 39.85898437716787157, 5.622872871577869525 ) ) ;
#2990=CIRCLE ( 'NONE', #6612, 11.57481594606304398 ) ;
#2991=EDGE_LOOP ( 'NONE', ( #24693, #11613, #10535, #26856, #19842, #22309, #27827, #24422, #25104, #11015 ) ) ;
#2992=DIRECTION ( 'NONE',  ( 0.000000000000000000, -1.000000000000000000, 0.000000000000000000 ) ) ;
#2996=CARTESIAN_POINT ( 'NONE',  ( 208.5748159460630120, 35.19570312716788152, -5.622872871577873077 ) ) ;
#3000=LINE ( 'NONE', #13673, #21644 ) ;
#3001=CARTESIAN_POINT ( 'NONE',  ( 13.14518615778179900, 36.33671875108394289, 5.444914386472293977 ) ) ;
#3002=CARTESIAN_POINT ( 'NONE',  ( 139.2950502721270425, 33.11210937608393579, -9.295050272127046043 ) ) ;
#3003=CARTESIAN_POINT ( 'NONE',  ( 72.17139121699895554, 31.99955315621561525, -11.52591757658528948 ) ) ;
#3006=CARTESIAN_POINT ( 'NONE',  ( 117.1602487631418086, 35.99999999999998579, 2.850296047819834033 ) ) ;
#3009=ADVANCED_FACE ( 'NONE', ( #10247 ), #18956, .F. ) ;
#3013=VECTOR ( 'NONE', #11470, 1000.000000000000000 ) ;
#3014=DIRECTION ( 'NONE',  ( 1.000000000000000000, 0.000000000000000000, 0.000000000000000000 ) ) ;
#3016=CARTESIAN_POINT ( 'NONE',  ( -8.049105076161786076E-16, 33.40976562608393863, -13.14518615778179544 ) ) ;
#3021=CARTESIAN_POINT ( 'NONE',  ( 181.8548138422181921, 35.84062500108394289, 5.444914386472304635 ) ) ;
#3022=VERTEX_POINT ( 'NONE', #19237 ) ;
#3024=CARTESIAN_POINT ( 'NONE',  ( 188.1264917564332109, 51.14166184781122837, -15.00000000000000000 ) ) ;
#3031=CARTESIAN_POINT ( 'NONE',  ( 130.0000000000000000, -7.395377635281828788, -1.503427012513233026E-14 ) ) ;
#3032=CARTESIAN_POINT ( 'NONE',  ( 124.5550856135277087, 39.11484375108394573, 13.14518615778179722 ) ) ;
#3033=CARTESIAN_POINT ( 'NONE',  ( -8.049105076161786076E-16, 36.58476562608393579, -13.14518615778179544 ) ) ;
#3034=CARTESIAN_POINT ( 'NONE',  ( -8.049105076161786076E-16, 35.59257812608393579, -13.14518615778179544 ) ) ;
#3037=CARTESIAN_POINT ( 'NONE',  ( 64.12347373463796885, 51.45968077935077645, -15.00000000000135536 ) ) ;
#3039=VERTEX_POINT ( 'NONE', #10804 ) ;
#3040=CARTESIAN_POINT ( 'NONE',  ( 78.24545034676866351, 35.99999999999998579, 2.307131236161231058 ) ) ;
#3044=ADVANCED_FACE ( 'NONE', ( #6266 ), #5235, .T. ) ;
#3045=CARTESIAN_POINT ( 'NONE',  ( 78.14518615778180788, 37.72578125108393010, 5.444914386472293977 ) ) ;
#3047=CARTESIAN_POINT ( 'NONE',  ( 208.1451861577818079, 36.23750000108393010, -5.444914386472297529 ) ) ;
#3048=EDGE_CURVE ( 'NONE', #22877, #5951, #10459, .T. ) ;
#3050=VERTEX_POINT ( 'NONE', #19166 ) ;
#3053=CARTESIAN_POINT ( 'NONE',  ( 181.8548138422182205, 39.21406250108392300, 5.444914386472304635 ) ) ;
#3056=EDGE_LOOP ( 'NONE', ( #5747, #12969, #24221, #139 ) ) ;
#3060=CARTESIAN_POINT ( 'NONE',  ( 139.2950502721270425, 32.31835937608393294, 9.295050272127046043 ) ) ;
#3063=EDGE_CURVE ( 'NONE', #10173, #13216, #16120, .T. ) ;
#3064=CARTESIAN_POINT ( 'NONE',  ( 208.1451861577817795, 34.84843750108393579, -5.444914386472297529 ) ) ;
#3069=CARTESIAN_POINT ( 'NONE',  ( 116.4251840539369454, 36.28710937716787299, -5.622872871577873077 ) ) ;
#3072=CARTESIAN_POINT ( 'NONE',  ( 3.100818213308542287E-15, 78.00000000000000000, 12.99999999999999645 ) ) ;
#3074=CARTESIAN_POINT ( 'NONE',  ( 189.5550856135277229, 39.80937500108392868, -13.14518615778179900 ) ) ;
#3076=ORIENTED_EDGE ( 'NONE', *, *, #1856, .F. ) ;
#3082=CARTESIAN_POINT ( 'NONE',  ( 139.5988444088204403, 38.42031250216787441, -9.598844408820458085 ) ) ;
#3083=CARTESIAN_POINT ( 'NONE',  ( 0.7050241099689084079, 36.00000000000001421, 13.13343125082108820 ) ) ;
#3084=CARTESIAN_POINT ( 'NONE',  ( 70.44491438647230552, 33.06250000108393294, 13.14518615778179189 ) ) ;
#3085=SURFACE_STYLE_USAGE ( .BOTH. , #10036 ) ;
#3087=VECTOR ( 'NONE', #22411, 1000.000000000000000 ) ;
#3088=DIRECTION ( 'NONE',  ( 0.000000000000000000, 0.000000000000000000, 1.000000000000000000 ) ) ;
#3089=CARTESIAN_POINT ( 'NONE',  ( -8.402315781222888802, 54.99999999485619639, 14.99999999999999822 ) ) ;
#3090=CARTESIAN_POINT ( 'NONE',  ( 59.37712712842223794, 40.85117187499999147, -13.57481594606315412 ) ) ;
#3091=CARTESIAN_POINT ( 'NONE',  ( 116.4251840539369596, 33.06249999999999289, 0.000000000000000000 ) ) ;
#3092=EDGE_CURVE ( 'NONE', #27029, #27310, #25419, .T. ) ;
#3094=FACE_BOUND ( 'NONE', #27669, .T. ) ;
#3098=CARTESIAN_POINT ( 'NONE',  ( 143.1451861577818079, 33.80664062608393294, -1.609821015232357215E-15 ) ) ;
#3100=CARTESIAN_POINT ( 'NONE',  ( 65.00000000000000000, 31.77265625216787370, 13.57481594606304576 ) ) ;
#3102=CARTESIAN_POINT ( 'NONE',  ( -9.295050272127044266, 37.47773437608393010, 9.295050272127047819 ) ) ;
#3106=CARTESIAN_POINT ( 'NONE',  ( 198.7556382656599396, 31.58960998161716560, -13.14518615778179900 ) ) ;
#3110=CARTESIAN_POINT ( 'NONE',  ( 127.9130013513679103, 36.00000000000000711, -13.31420566034935327 ) ) ;
#3118=CARTESIAN_POINT ( 'NONE',  ( 189.3771271284221314, 32.41757812499999858, 13.57481594606304753 ) ) ;
#3122=CARTESIAN_POINT ( 'NONE',  ( 95.54126587499996504, 83.43750000136560629, -1.387778780781445676E-14 ) ) ;
#3123=CARTESIAN_POINT ( 'NONE',  ( 55.70494972787295751, 31.92148437608393508, 9.295050272127047819 ) ) ;
#3124=( BOUNDED_CURVE ( )  B_SPLINE_CURVE ( 2, ( #18841, #23130, #10129, #27549, #21834, #19263, #4441, #8848, #27963 ),
 .UNSPECIFIED., .F., .F. ) 
 B_SPLINE_CURVE_WITH_KNOTS ( ( 3, 2, 2, 2, 3 ),
 ( 0.06250000000000004163, 0.07291666666666665741, 0.08333333333333325932, 0.09374999999999987510, 0.1041666666666664909 ),
 .UNSPECIFIED. ) 
 CURVE ( )  GEOMETRIC_REPRESENTATION_ITEM ( )  RATIONAL_B_SPLINE_CURVE ( ( 0.9999999999999996669, 0.9238795325112870716, 1.000000000000000000, 0.9238795325112867385, 1.000000000000000000, 0.9238795325112867385, 1.000000000000000000, 0.9238795325112880708, 0.9999999999999986677 ) ) 
 REPRESENTATION_ITEM ( '' )  );
#3128=CARTESIAN_POINT ( 'NONE',  ( 120.4011555911795455, 38.02343750216788010, 9.598844408820459861 ) ) ;
#3129=CARTESIAN_POINT ( 'NONE',  ( -9.598844408820454532, 33.95546874999999432, 9.598844408820459861 ) ) ;
#3131=CARTESIAN_POINT ( 'NONE',  ( 143.1451861577818079, 33.26093750108393721, -5.444914386472297529 ) ) ;
#3133=CARTESIAN_POINT ( 'NONE',  ( 103.1528011352953342, 84.06250000136560629, -3.152801135295383084 ) ) ;
#3135=CARTESIAN_POINT ( 'NONE',  ( 55.40115559117954547, 38.81718750216787583, 9.598844408820459861 ) ) ;
#3139=CARTESIAN_POINT ( 'NONE',  ( 185.7049497278729575, 39.06523437608392868, -9.295050272127046043 ) ) ;
#3141=FACE_OUTER_BOUND ( 'NONE', #14026, .T. ) ;
#3143=CARTESIAN_POINT ( 'NONE',  ( 183.3096217544866420, 35.99999999999998579, -6.307928093363108779 ) ) ;
#3148=CARTESIAN_POINT ( 'NONE',  ( 204.2950502721270425, 39.46210937608393010, -9.295050272127046043 ) ) ;
#3151=CARTESIAN_POINT ( 'NONE',  ( 130.0000000000000000, 32.41757812608393863, -13.14518615778179544 ) ) ;
#3156=CARTESIAN_POINT ( 'NONE',  ( -9.598844408820458085, 37.82500000216787583, -9.598844408820458085 ) ) ;
#3160=CARTESIAN_POINT ( 'NONE',  ( 104.9999999999999716, 83.56250000273119838, 2.071067811865462627 ) ) ;
#3162=CARTESIAN_POINT ( 'NONE',  ( -5.444914386472297529, 33.45937500108394147, -13.14518615778179900 ) ) ;
#3166=CARTESIAN_POINT ( 'NONE',  ( 208.1451861577818079, 36.98164062608393010, -1.609821015232357215E-15 ) ) ;
#3171=VERTEX_POINT ( 'NONE', #13110 ) ;
#3176=DIRECTION ( 'NONE',  ( -0.000000000000000000, 1.000000000000000000, -0.000000000000000000 ) ) ;
#3177=AXIS2_PLACEMENT_3D ( 'NONE', #16031, #18612, #7910 ) ;
#3178=CARTESIAN_POINT ( 'NONE',  ( 116.8548138422182063, 38.22187500108393010, 5.444914386472304635 ) ) ;
#3179=CARTESIAN_POINT ( 'NONE',  ( -5.444914386472297529, 38.22187500108393721, -13.14518615778179722 ) ) ;
#3180=CARTESIAN_POINT ( 'NONE',  ( 9.295050272127046043, 36.28710937608393294, -9.295050272127046043 ) ) ;
#3187=CARTESIAN_POINT ( 'NONE',  ( 51.85481384221820633, 36.58476562608393579, 0.000000000000000000 ) ) ;
#3188=CARTESIAN_POINT ( 'NONE',  ( -20.00000000000000355, 55.00000000000000000, -14.99999999999999822 ) ) ;
#3189=CARTESIAN_POINT ( 'NONE',  ( 189.5550856135277229, 36.73359375108393010, 13.14518615778179722 ) ) ;
#3193=CARTESIAN_POINT ( 'NONE',  ( 208.1451861577818079, 37.97382812608393721, -1.609821015232357215E-15 ) ) ;
#3198=ORIENTED_EDGE ( 'NONE', *, *, #22826, .F. ) ;
#3199=CARTESIAN_POINT ( 'NONE',  ( 208.5748159460630688, 37.47773437716787015, 5.622872871577868636 ) ) ;
#3200=CARTESIAN_POINT ( 'NONE',  ( 51.85481384221820633, 39.90859375108393436, -5.444914386472297529 ) ) ;
#3202=CARTESIAN_POINT ( 'NONE',  ( 200.4449143864723055, 34.15390625108393863, -13.14518615778179900 ) ) ;
#3203=ORIENTED_EDGE ( 'NONE', *, *, #23415, .F. ) ;
#3206=CARTESIAN_POINT ( 'NONE',  ( 195.3247243111960643, 53.49346745874645137, 14.99999999999994849 ) ) ;
#3208=CARTESIAN_POINT ( 'NONE',  ( 135.6228728715778686, 37.67617187716787441, -13.57481594606304753 ) ) ;
#3214=CIRCLE ( 'NONE', #2307, 5.000000000000000888 ) ;
#3222=CARTESIAN_POINT ( 'NONE',  ( 51.85481384221820633, 33.60820312608393579, 0.000000000000000000 ) ) ;
#3227=CARTESIAN_POINT ( 'NONE',  ( 1.505492181556994380, 53.60078691996478284, 14.99999999999999645 ) ) ;
#3228=CARTESIAN_POINT ( 'NONE',  ( -15.00000000000000355, 55.00000000000000000, -9.999999999999998224 ) ) ;
#3229=CARTESIAN_POINT ( 'NONE',  ( 130.0000000000000000, 32.86406249999999574, -13.57481594606304576 ) ) ;
#3231=CARTESIAN_POINT ( 'NONE',  ( 104.9999999999999716, 84.43750000000000000, 2.071067811865462627 ) ) ;
#3236=CARTESIAN_POINT ( 'NONE',  ( 130.0000000000000000, 32.02070312608393010, 13.14518615778179544 ) ) ;
#3237=CARTESIAN_POINT ( 'NONE',  ( 51.85481384221820633, 38.96601562608393721, 0.000000000000000000 ) ) ;
#3240=CARTESIAN_POINT ( 'NONE',  ( 9.295050272127047819, 38.46992187608393010, 9.295050272127046043 ) ) ;
#3245=LINE ( 'NONE', #19033, #4898 ) ;
#3248=CARTESIAN_POINT ( 'NONE',  ( 104.9999999999999716, 82.68750000273119838, -2.071067811865491937 ) ) ;
#3249=DIRECTION ( 'NONE',  ( 0.8660254037844407060, 0.4999999999999963363, 0.000000000000000000 ) ) ;
#3260=EDGE_CURVE ( 'NONE', #17753, #21288, #13398, .T. ) ;
#3263=CARTESIAN_POINT ( 'NONE',  ( 104.4587341249999639, 82.93750000136560629, -1.442382525525748735E-14 ) ) ;
#3264=CARTESIAN_POINT ( 'NONE',  ( 70.44491438647230552, 33.16171875108393152, -13.14518615778179900 ) ) ;
#3265=LINE ( 'NONE', #9245, #8019 ) ;
#3267=CARTESIAN_POINT ( 'NONE',  ( 9.598844408820459861, 37.32890624999999574, 9.598844408820456309 ) ) ;
#3268=CARTESIAN_POINT ( 'NONE',  ( -9.598844408820458085, 34.55078124999999289, -9.598844408820458085 ) ) ;
#3270=CARTESIAN_POINT ( 'NONE',  ( 124.5550856135277087, 34.25312500108393010, -13.14518615778179900 ) ) ;
#3273=CARTESIAN_POINT ( 'NONE',  ( 208.5748159460630688, 36.68398437716787441, 5.622872871577868636 ) ) ;
#3274=CARTESIAN_POINT ( 'NONE',  ( 94.99999999999995737, 80.06250000273118417, -2.071067811865491048 ) ) ;
#3278=CARTESIAN_POINT ( 'NONE',  ( 181.8548138422182205, 31.82226562608393650, 0.000000000000000000 ) ) ;
#3279=CARTESIAN_POINT ( 'NONE',  ( -13.57481594606304576, 39.51171875216787299, 0.000000000000000000 ) ) ;
#3284=CARTESIAN_POINT ( 'NONE',  ( 181.8548138422181921, 40.50390625108394005, -5.444914386472297529 ) ) ;
#3285=CARTESIAN_POINT ( 'NONE',  ( 2.493653234604083739E-15, 36.53515625216787299, 13.57481594606304576 ) ) ;
#3286=EDGE_CURVE ( 'NONE', #144, #21487, #180, .T. ) ;
#3288=CARTESIAN_POINT ( 'NONE',  ( 195.0000000000000000, 38.12265625216787157, 13.57481594606304576 ) ) ;
#3289=CARTESIAN_POINT ( 'NONE',  ( 2.414731522848535132E-15, 32.21914062608393436, 13.14518615778179544 ) ) ;
#3292=CARTESIAN_POINT ( 'NONE',  ( 59.37712712842213136, 32.91367187499999858, -13.57481594606304753 ) ) ;
#3295=CARTESIAN_POINT ( 'NONE',  ( 70.62287287157795390, 36.58476562716786873, 13.57481594606297115 ) ) ;
#3303=CARTESIAN_POINT ( 'NONE',  ( -9.295050272127046043, 32.71523437608393436, -9.295050272127046043 ) ) ;
#3305=CARTESIAN_POINT ( 'NONE',  ( 124.3771271284221740, 37.18007812499999432, 13.57481594606311504 ) ) ;
#3308=CARTESIAN_POINT ( 'NONE',  ( 208.1451861577817795, 33.06250000108393294, -5.444914386472297529 ) ) ;
#3309=ORIENTED_EDGE ( 'NONE', *, *, #27913, .T. ) ;
#3310=CARTESIAN_POINT ( 'NONE',  ( 186.7985538123501215, 50.69246985422704910, -14.99999999999999822 ) ) ;
#3315=CARTESIAN_POINT ( 'NONE',  ( 181.4251840539369596, 40.25585937716787299, -5.622872871577873077 ) ) ;
#3317=CARTESIAN_POINT ( 'NONE',  ( 143.1451861577818079, 37.03125000108393294, -5.444914386472297529 ) ) ;
#3318=CARTESIAN_POINT ( 'NONE',  ( -13.14518615778179544, 39.16445312608393436, 0.000000000000000000 ) ) ;
#3319=CARTESIAN_POINT ( 'NONE',  ( -8.049105076161786076E-16, 40.55351562608393579, -13.14518615778179544 ) ) ;
#3321=DIRECTION ( 'NONE',  ( -0.000000000000000000, 1.000000000000000000, -0.000000000000000000 ) ) ;
#3326=CARTESIAN_POINT ( 'NONE',  ( 195.0000000000000000, 36.00000000000000000, -2.255140518769849538E-14 ) ) ;
#3327=CARTESIAN_POINT ( 'NONE',  ( 0.000000000000000000, -7.395377635281828788, 0.000000000000000000 ) ) ;
#3328=CARTESIAN_POINT ( 'NONE',  ( 204.2950502721270425, 36.08867187608392868, 9.295050272127046043 ) ) ;
#3331=EDGE_CURVE ( 'NONE', #16904, #8652, #25972, .T. ) ;
#3334=CARTESIAN_POINT ( 'NONE',  ( 182.3184072029388005, 36.04503594658365984, 5.908507747192915716 ) ) ;
#3339=CARTESIAN_POINT ( 'NONE',  ( 65.00000000000000000, 31.62382812608393579, -13.14518615778179544 ) ) ;
#3340=VERTEX_POINT ( 'NONE', #24117 ) ;
#3343=CARTESIAN_POINT ( 'NONE',  ( 204.2950502721270425, 33.11210937608393579, 9.295050272127046043 ) ) ;
#3346=CARTESIAN_POINT ( 'NONE',  ( 8.268597328390889345, 50.00000000054355098, -10.78867689284122733 ) ) ;
#3348=CARTESIAN_POINT ( 'NONE',  ( 124.3771271284221314, 36.98164062716787015, -13.57481594606304753 ) ) ;
#3351=CARTESIAN_POINT ( 'NONE',  ( 208.1451861577817795, 37.22968750108393721, -5.444914386472297529 ) ) ;
#3352=ORIENTED_EDGE ( 'NONE', *, *, #971, .F. ) ;
#3355=CARTESIAN_POINT ( 'NONE',  ( 136.0859442160083859, 54.65299103241780898, 14.99999999999996092 ) ) ;
#3357=CARTESIAN_POINT ( 'NONE',  ( 65.00000000000000000, 31.82226562608393650, -13.14518615778179544 ) ) ;
#3358=VECTOR ( 'NONE', #22604, 1000.000000000000000 ) ;
#3360=CARTESIAN_POINT ( 'NONE',  ( -5.622872871577890841, 39.66054687716787441, 13.57481594606302444 ) ) ;
#3362=CARTESIAN_POINT ( 'NONE',  ( 143.5748159460630404, 34.30273437500000000, -5.622872871577873077 ) ) ;
#3365=CARTESIAN_POINT ( 'NONE',  ( 219.9999999999999716, 55.00000000000000000, 14.99999999999994316 ) ) ;
#3369=CARTESIAN_POINT ( 'NONE',  ( 143.1451861577818079, 39.61093750108393863, -5.444914386472297529 ) ) ;
#3370=CARTESIAN_POINT ( 'NONE',  ( 51.85481384221819923, 40.50390625108394005, -5.444914386472297529 ) ) ;
#3371=VERTEX_POINT ( 'NONE', #25829 ) ;
#3372=CARTESIAN_POINT ( 'NONE',  ( 0.000000000000000000, 36.00000000000000000, 0.000000000000000000 ) ) ;
#3373=CARTESIAN_POINT ( 'NONE',  ( -5.444914386472297529, 37.22968750108393721, -13.14518615778179900 ) ) ;
#3378=CARTESIAN_POINT ( 'NONE',  ( 201.9444237971526661, 31.55306878032414986, -11.16113333171310451 ) ) ;
#3379=DIRECTION ( 'NONE',  ( 0.000000000000000000, 0.000000000000000000, 1.000000000000000000 ) ) ;
#3382=CARTESIAN_POINT ( 'NONE',  ( 125.5405265863609969, 36.00000000000002842, -12.68347323196757337 ) ) ;
#3383=EDGE_CURVE ( 'NONE', #21141, #9074, #11023, .T. ) ;
#3384=CARTESIAN_POINT ( 'NONE',  ( 130.0000000000000000, 40.10703125216787157, -13.57481594606304576 ) ) ;
#3387=EDGE_LOOP ( 'NONE', ( #12731, #6830, #16012, #16694 ) ) ;
#3394=CARTESIAN_POINT ( 'NONE',  ( 104.4587341249999781, 82.87500000136560629, 1.846868145590721655 ) ) ;
#3395=CARTESIAN_POINT ( 'NONE',  ( 59.55508561352770158, 33.55859375108393294, 13.14518615778179722 ) ) ;
#3396=CYLINDRICAL_SURFACE ( 'NONE', #21703, 5.000000000000004441 ) ;
#3398=( BOUNDED_CURVE ( )  B_SPLINE_CURVE ( 2, ( #1880, #4286, #2010, #153, #19386, #27952, #10959, #12676, #15232 ),
 .UNSPECIFIED., .F., .F. ) 
 B_SPLINE_CURVE_WITH_KNOTS ( ( 3, 2, 2, 2, 3 ),
 ( 0.3500000000000003109, 0.3750000000000003331, 0.4000000000000003553, 0.4250000000000003775, 0.4500000000000003997 ),
 .UNSPECIFIED. ) 
 CURVE ( )  GEOMETRIC_REPRESENTATION_ITEM ( )  RATIONAL_B_SPLINE_CURVE ( ( 0.9999999999999990008, 0.9238795325112877377, 1.000000000000000000, 0.9238795325112867385, 1.000000000000000000, 0.9238795325112867385, 1.000000000000000000, 0.9238795325112855172, 1.000000000000001110 ) ) 
 REPRESENTATION_ITEM ( '' )  );
#3401=CARTESIAN_POINT ( 'NONE',  ( -9.598844408820454532, 32.36796874999999574, 9.598844408820459861 ) ) ;
#3403=CARTESIAN_POINT ( 'NONE',  ( 130.0000000000000000, 33.80664062608393294, 13.14518615778179544 ) ) ;
#3405=ADVANCED_FACE ( 'NONE', ( #898 ), #20265, .T. ) ;
#3406=CARTESIAN_POINT ( 'NONE',  ( 204.5988444088204687, 36.63437500216787157, 9.598844408820456309 ) ) ;
#3407=CARTESIAN_POINT ( 'NONE',  ( 98.15313185440925281, 81.62500000136560629, 4.458734124999987891 ) ) ;
#3408=CARTESIAN_POINT ( 'NONE',  ( 116.8548138422182205, 39.75976562608393294, 0.000000000000000000 ) ) ;
#3409=CARTESIAN_POINT ( 'NONE',  ( 74.59884440882045453, 39.21406250216787015, -9.598844408820458085 ) ) ;
#3413=CARTESIAN_POINT ( 'NONE',  ( 200.4449143864723055, 39.41250000108393436, 13.14518615778179189 ) ) ;
#3414=CARTESIAN_POINT ( 'NONE',  ( 5.622872871577878406, 38.96601562716787015, 13.57481594606304576 ) ) ;
#3418=ORIENTED_EDGE ( 'NONE', *, *, #13399, .F. ) ;
#3420=CARTESIAN_POINT ( 'NONE',  ( 195.0000000000000000, 40.35507812608393152, -13.14518615778179544 ) ) ;
#3423=CARTESIAN_POINT ( 'NONE',  ( 139.2950502721270425, 40.05742187608392868, 9.295050272127046043 ) ) ;
#3424=CARTESIAN_POINT ( 'NONE',  ( -9.295050272127046043, 33.50898437608393010, -9.295050272127046043 ) ) ;
#3428=CARTESIAN_POINT ( 'NONE',  ( 195.0000000000000000, 33.01289062608393721, 13.14518615778179544 ) ) ;
#3429=EDGE_CURVE ( 'NONE', #5791, #10301, #673, .T. ) ;
#3438=LINE ( 'NONE', #20408, #19355 ) ;
#3439=CARTESIAN_POINT ( 'NONE',  ( -13.14518615778179544, 34.40195312608393152, 0.000000000000000000 ) ) ;
#3442=CARTESIAN_POINT ( 'NONE',  ( 95.54126587499996504, 82.68750000136560629, -1.387778780781445676E-14 ) ) ;
#3446=EDGE_CURVE ( 'NONE', #1909, #24277, #8462, .T. ) ;
#3447=CARTESIAN_POINT ( 'NONE',  ( 208.1451861577818079, 33.80664062608393294, -1.609821015232357215E-15 ) ) ;
#3449=CARTESIAN_POINT ( 'NONE',  ( 186.6040612587084695, 54.99999999495823033, -15.00000000000000533 ) ) ;
#3451=ORIENTED_EDGE ( 'NONE', *, *, #160, .F. ) ;
#3453=( BOUNDED_CURVE ( )  B_SPLINE_CURVE ( 2, ( #22997, #20044, #18438, #3467, #2662, #27147, #24990, #13456, #12133 ),
 .UNSPECIFIED., .F., .F. ) 
 B_SPLINE_CURVE_WITH_KNOTS ( ( 3, 2, 2, 2, 3 ),
 ( 0.1458333333333336757, 0.1562500000000002776, 0.1666666666666669072, 0.1770833333333335369, 0.1875000000000001388 ),
 .UNSPECIFIED. ) 
 CURVE ( )  GEOMETRIC_REPRESENTATION_ITEM ( )  RATIONAL_B_SPLINE_CURVE ( ( 0.9999999999999975575, 0.9238795325112891810, 1.000000000000000000, 0.9238795325112867385, 1.000000000000000000, 0.9238795325112867385, 1.000000000000000000, 0.9238795325112857393, 1.000000000000001110 ) ) 
 REPRESENTATION_ITEM ( '' )  );
#3455=CARTESIAN_POINT ( 'NONE',  ( 5.622872871578008080, 36.08867187716787583, -13.57481594606290898 ) ) ;
#3457=CARTESIAN_POINT ( 'NONE',  ( -5.444914386472299306, 39.31328125108392868, 13.14518615778179722 ) ) ;
#3458=CARTESIAN_POINT ( 'NONE',  ( -13.14518615778179189, 40.00781250108393294, 5.444914386472304635 ) ) ;
#3460=VECTOR ( 'NONE', #2706, 1000.000000000000000 ) ;
#3462=CARTESIAN_POINT ( 'NONE',  ( -15.00000000000000355, 50.00000000000000000, -9.999999999999998224 ) ) ;
#3465=CARTESIAN_POINT ( 'NONE',  ( 95.54126587499996504, 81.62500000136560629, -1.846868145590750077 ) ) ;
#3467=CARTESIAN_POINT ( 'NONE',  ( -13.57481594606304398, 38.76757812716787299, 5.622872871577880183 ) ) ;
#3468=CARTESIAN_POINT ( 'NONE',  ( 68.03939705080254896, 53.88964894337313183, 14.99999999999997868 ) ) ;
#3472=CARTESIAN_POINT ( 'NONE',  ( -20.00000000000000000, 50.00000000000000000, 10.00000000000000178 ) ) ;
#3476=LINE ( 'NONE', #8024, #3497 ) ;
#3480=CARTESIAN_POINT ( 'NONE',  ( 74.29505027212704249, 39.66054687608393436, -9.295050272127046043 ) ) ;
#3482=DIRECTION ( 'NONE',  ( 0.000000000000000000, -1.000000000000000000, -0.000000000000000000 ) ) ;
#3483=CARTESIAN_POINT ( 'NONE',  ( 181.8548138422182205, 32.02070312608393010, 0.000000000000000000 ) ) ;
#3487=CARTESIAN_POINT ( 'NONE',  ( 203.3922152916383936, 54.99999999999998579, 14.99999999999994316 ) ) ;
#3488=( BOUNDED_CURVE ( )  B_SPLINE_CURVE ( 2, ( #19860, #9034, #17726, #10594, #8605, #4336, #7450, #921, #24420 ),
 .UNSPECIFIED., .F., .F. ) 
 B_SPLINE_CURVE_WITH_KNOTS ( ( 3, 2, 2, 2, 3 ),
 ( 0.3958333333333331483, 0.4062499999999999445, 0.4166666666666667407, 0.4270833333333335369, 0.4375000000000003331 ),
 .UNSPECIFIED. ) 
 CURVE ( )  GEOMETRIC_REPRESENTATION_ITEM ( )  RATIONAL_B_SPLINE_CURVE ( ( 1.000000000000001110, 0.9238795325112855172, 1.000000000000000000, 0.9238795325112867385, 1.000000000000000000, 0.9238795325112867385, 1.000000000000000000, 0.9238795325112842960, 1.000000000000002442 ) ) 
 REPRESENTATION_ITEM ( '' )  );
#3489=CARTESIAN_POINT ( 'NONE',  ( 143.5748159460630688, 38.32109375216786873, -1.662435489736055892E-15 ) ) ;
#3490=VECTOR ( 'NONE', #6838, 1000.000000000000000 ) ;
#3494=CARTESIAN_POINT ( 'NONE',  ( 208.1451861577817795, 37.92421875108392726, 5.444914386472293977 ) ) ;
#3497=VECTOR ( 'NONE', #1488, 1000.000000000000000 ) ;
#3498=CARTESIAN_POINT ( 'NONE',  ( -1.816500417285228597, 36.00000000000000711, -13.35830014193482285 ) ) ;
#3499=CARTESIAN_POINT ( 'NONE',  ( 13.57481594606304576, 39.80937499999999574, -1.662435489736055892E-15 ) ) ;
#3501=CARTESIAN_POINT ( 'NONE',  ( 95.54126587499996504, 83.37500000136563472, -1.846868145590750077 ) ) ;
#3502=LINE ( 'NONE', #12439, #8056 ) ;
#3505=CARTESIAN_POINT ( 'NONE',  ( 5.622872871577976994, 40.75195312499999289, -13.57481594606294095 ) ) ;
#3508=CARTESIAN_POINT ( 'NONE',  ( 135.6228728715778686, 32.81445312499999289, -13.57481594606304753 ) ) ;
#3510=CARTESIAN_POINT ( 'NONE',  ( 70.62287287157784021, 36.48554687499999716, 13.57481594606309194 ) ) ;
#3517=CARTESIAN_POINT ( 'NONE',  ( 120.7049497278729575, 38.27148437608393294, -9.295050272127046043 ) ) ;
#3518=CARTESIAN_POINT ( 'NONE',  ( 74.29505027212704249, 36.08867187608392868, 9.295050272127046043 ) ) ;
#3520=ORIENTED_EDGE ( 'NONE', *, *, #27613, .T. ) ;
#3522=CARTESIAN_POINT ( 'NONE',  ( 9.295050272127047819, 39.26367187608393294, 9.295050272127046043 ) ) ;
#3524=CARTESIAN_POINT ( 'NONE',  ( 186.8746960822089136, 36.00000000000000711, 10.34220695173589810 ) ) ;
#3528=CARTESIAN_POINT ( 'NONE',  ( 208.5748159460630688, 40.65273437499999432, -5.622872871577873966 ) ) ;
#3529=CARTESIAN_POINT ( 'NONE',  ( 195.0000000000000000, 32.41757812608393863, -13.14518615778179544 ) ) ;
#3530=DIRECTION ( 'NONE',  ( 0.000000000000000000, 0.000000000000000000, -1.000000000000000000 ) ) ;
#3533=CARTESIAN_POINT ( 'NONE',  ( 117.4334932752013145, 36.00000000000000000, -4.295155080288600047 ) ) ;
#3534=( BOUNDED_CURVE ( )  B_SPLINE_CURVE ( 2, ( #9992, #3455, #23262, #14127, #22706 ),
 .UNSPECIFIED., .F., .F. ) 
 B_SPLINE_CURVE_WITH_KNOTS ( ( 3, 2, 3 ),
 ( 0.4375000000000003331, 0.4479166666666667962, 0.4520580917964582834 ),
 .UNSPECIFIED. ) 
 CURVE ( )  GEOMETRIC_REPRESENTATION_ITEM ( )  RATIONAL_B_SPLINE_CURVE ( ( 0.9999999999999975575, 0.9238795325112891810, 1.000000000000000000, 0.9697362671728727568, 0.9635368512068458458 ) ) 
 REPRESENTATION_ITEM ( '' )  );
#3535=DIRECTION ( 'NONE',  ( 0.000000000000000000, 0.000000000000000000, 1.000000000000000000 ) ) ;
#3544=CARTESIAN_POINT ( 'NONE',  ( 99.99999999999995737, 79.68750000136559208, 4.458734124999988779 ) ) ;
#3545=CARTESIAN_POINT ( 'NONE',  ( 78.14518615778179367, 33.75703125108393010, 5.444914386472293977 ) ) ;
#3549=DIRECTION ( 'NONE',  ( -1.000000000000000000, 0.000000000000000000, -0.000000000000000000 ) ) ;
#3551=CARTESIAN_POINT ( 'NONE',  ( 143.1451861577818079, 35.54296875108394715, 5.444914386472293977 ) ) ;
#3553=CARTESIAN_POINT ( 'NONE',  ( 1.605271876576585877, 53.60388944777323417, -15.00000000000000355 ) ) ;
#3556=CARTESIAN_POINT ( 'NONE',  ( 130.0000000000000000, 39.16445312608392726, 13.14518615778179544 ) ) ;
#3557=CARTESIAN_POINT ( 'NONE',  ( 65.00000000000000000, 40.10703125216787157, -13.57481594606304576 ) ) ;
#3559=CARTESIAN_POINT ( 'NONE',  ( 5.622872871577871301, 39.26367187716787299, -13.57481594606304753 ) ) ;
#3560=VERTEX_POINT ( 'NONE', #27260 ) ;
#3564=CARTESIAN_POINT ( 'NONE',  ( 204.5988444088204687, 31.87187500216787228, 9.598844408820456309 ) ) ;
#3568=CARTESIAN_POINT ( 'NONE',  ( 143.1451861577818079, 38.56914062608393579, -1.609821015232357215E-15 ) ) ;
#3569=CARTESIAN_POINT ( 'NONE',  ( 5.444914386472297529, 32.56640625108394005, -13.14518615778179900 ) ) ;
#3575=CARTESIAN_POINT ( 'NONE',  ( 208.5748159460630120, 37.37851562499999858, 5.622872871577869525 ) ) ;
#3584=CARTESIAN_POINT ( 'NONE',  ( 5.622872871577878406, 38.86679687499999858, 13.57481594606304576 ) ) ;
#3586=EDGE_CURVE ( 'NONE', #7991, #9045, #19962, .T. ) ;
#3588=CARTESIAN_POINT ( 'NONE',  ( 104.4587341249999781, 83.12500000136560629, 1.846868145590721655 ) ) ;
#3590=FACE_OUTER_BOUND ( 'NONE', #3656, .T. ) ;
#3592=ORIENTED_EDGE ( 'NONE', *, *, #1010, .F. ) ;
#3593=CARTESIAN_POINT ( 'NONE',  ( 194.6030005853479850, 51.45716825712459297, -15.00000000000067324 ) ) ;
#3599=CARTESIAN_POINT ( 'NONE',  ( 204.5988444088204687, 39.80937500216786873, 9.598844408820456309 ) ) ;
#3602=VECTOR ( 'NONE', #28060, 1000.000000000000000 ) ;
#3603=CARTESIAN_POINT ( 'NONE',  ( 130.0000000000000000, 39.36289062608393152, 13.14518615778179544 ) ) ;
#3604=CARTESIAN_POINT ( 'NONE',  ( -13.14518615778179900, 31.77265625108393365, -5.444914386472297529 ) ) ;
#3605=CARTESIAN_POINT ( 'NONE',  ( 59.37712712842213136, 37.67617187499999432, -13.57481594606304753 ) ) ;
#3606=CARTESIAN_POINT ( 'NONE',  ( 65.00000000000000000, -7.395377635281828788, 13.57481594606303688 ) ) ;
#3607=EDGE_CURVE ( 'NONE', #1074, #11913, #13690, .T. ) ;
#3608=CARTESIAN_POINT ( 'NONE',  ( -13.57481594606304576, 37.13046875216787868, 0.000000000000000000 ) ) ;
#3611=CARTESIAN_POINT ( 'NONE',  ( 99.99999999999995737, 81.93750000136559208, 4.458734124999988779 ) ) ;
#3613=CARTESIAN_POINT ( 'NONE',  ( 70.62287287157774074, 38.96601562716787015, 13.57481594606318076 ) ) ;
#3614=CARTESIAN_POINT ( 'NONE',  ( 71.07908002051881624, 54.65154858643460756, 14.99999999999997513 ) ) ;
#3625=CARTESIAN_POINT ( 'NONE',  ( 55.70494972787295751, 39.26367187608393294, 9.295050272127047819 ) ) ;
#3627=CARTESIAN_POINT ( 'NONE',  ( -5.622872871578011633, 39.56132812500000284, 13.57481594606290720 ) ) ;
#3628=ORIENTED_EDGE ( 'NONE', *, *, #11512, .F. ) ;
#3630=LINE ( 'NONE', #12293, #23172 ) ;
#3631=DIRECTION ( 'NONE',  ( -0.000000000000000000, 1.000000000000000000, -0.000000000000000000 ) ) ;
#3632=CARTESIAN_POINT ( 'NONE',  ( 135.6228728715778971, 34.20351562716788862, 13.57481594606304576 ) ) ;
#3633=CARTESIAN_POINT ( 'NONE',  ( 55.40115559117954547, 40.20625000216787726, -9.598844408820458085 ) ) ;
#3636=CARTESIAN_POINT ( 'NONE',  ( 181.8548138422182205, 38.37070312608393152, 0.000000000000000000 ) ) ;
#3637=EDGE_LOOP ( 'NONE', ( #10292, #16089 ) ) ;
#3638=VERTEX_POINT ( 'NONE', #2876 ) ;
#3642=CARTESIAN_POINT ( 'NONE',  ( 103.1528011352953342, 83.06250000136560629, -3.152801135295383084 ) ) ;
#3643=CARTESIAN_POINT ( 'NONE',  ( 65.00000000000000000, 40.10703125216787157, -13.57481594606304576 ) ) ;
#3646=CARTESIAN_POINT ( 'NONE',  ( -13.57481594606304753, 39.46210937716787726, -5.622872871577872189 ) ) ;
#3648=CARTESIAN_POINT ( 'NONE',  ( 99.99999999999995737, 83.25000000000000000, 4.999999999999990230 ) ) ;
#3650=ORIENTED_EDGE ( 'NONE', *, *, #11058, .T. ) ;
#3653=CARTESIAN_POINT ( 'NONE',  ( 102.0710678118654329, 84.31250000000000000, 4.999999999999999112 ) ) ;
#3656=EDGE_LOOP ( 'NONE', ( #3628, #19484, #11881, #4808 ) ) ;
#3659=CARTESIAN_POINT ( 'NONE',  ( 116.8548138422182063, 39.21406250108392300, 5.444914386472304635 ) ) ;
#3660=CARTESIAN_POINT ( 'NONE',  ( 55.70494972787295751, 38.07304687608393579, -9.295050272127046043 ) ) ;
#3663=CARTESIAN_POINT ( 'NONE',  ( 5.444914386472297529, 37.13046875108393152, -13.14518615778179900 ) ) ;
#3664=CARTESIAN_POINT ( 'NONE',  ( 51.42518405393695957, 36.28710937499999289, 5.622872871577880183 ) ) ;
#3666=CARTESIAN_POINT ( 'NONE',  ( 195.0000000000000000, 36.53515625216787299, 13.57481594606304576 ) ) ;
#3667=CARTESIAN_POINT ( 'NONE',  ( 99.99999999999995737, 81.75000000000000000, -5.000000000000018652 ) ) ;
#3670=DIRECTION ( 'NONE',  ( -0.000000000000000000, 0.000000000000000000, -1.000000000000000000 ) ) ;
#3671=CARTESIAN_POINT ( 'NONE',  ( 2.414731522848535132E-15, 37.57695312608392868, 13.14518615778179544 ) ) ;
#3672=CARTESIAN_POINT ( 'NONE',  ( 131.6855116490828834, 35.99999999999997868, 13.05727741351676130 ) ) ;
#3675=CARTESIAN_POINT ( 'NONE',  ( 116.8473230904128002, 35.99999999999999289, 0.5874252385153416745 ) ) ;
#3677=ORIENTED_EDGE ( 'NONE', *, *, #27980, .T. ) ;
#3683=CARTESIAN_POINT ( 'NONE',  ( 99.99999999999995737, 84.43750000136560629, -4.458734125000016313 ) ) ;
#3684=CARTESIAN_POINT ( 'NONE',  ( 65.00000000000000000, 37.37851562608393863, -13.14518615778179544 ) ) ;
#3690=CARTESIAN_POINT ( 'NONE',  ( 143.5748159460630404, 39.75976562499999289, 5.622872871577869525 ) ) ;
#3695=CARTESIAN_POINT ( 'NONE',  ( 95.54126587499996504, 81.43750000136559208, -1.387778780781445676E-14 ) ) ;
#3696=CARTESIAN_POINT ( 'NONE',  ( 120.7049497278729575, 39.06523437608392868, 9.295050272127047819 ) ) ;
#3697=CARTESIAN_POINT ( 'NONE',  ( 51.42518405393695957, 37.18007812716787441, 5.622872871577880183 ) ) ;
#3700=CARTESIAN_POINT ( 'NONE',  ( 9.598844408820456309, 35.24531250216787726, -9.598844408820458085 ) ) ;
#3706=CARTESIAN_POINT ( 'NONE',  ( 208.1451861577817795, 37.03125000108393294, -5.444914386472297529 ) ) ;
#3708=CARTESIAN_POINT ( 'NONE',  ( 130.0000000000000000, 37.97382812608393721, -13.14518615778179544 ) ) ;
#3709=CARTESIAN_POINT ( 'NONE',  ( -13.14518615778179544, 32.81445312608393294, 0.000000000000000000 ) ) ;
#3710=DIRECTION ( 'NONE',  ( 1.000000000000000000, 0.000000000000000000, -0.000000000000000000 ) ) ;
#3714=CARTESIAN_POINT ( 'NONE',  ( 204.5988444088204403, 36.73359374999999716, -9.598844408820458085 ) ) ;
#3716=CARTESIAN_POINT ( 'NONE',  ( 125.6259778691823641, 36.00000000000001421, 12.40367315690590466 ) ) ;
#3718=CARTESIAN_POINT ( 'NONE',  ( 65.00000000000000000, 39.95820312608393010, 13.14518615778179544 ) ) ;
#3724=CARTESIAN_POINT ( 'NONE',  ( -8.312177448680279460E-16, 39.21406249999999716, -13.57481594606304576 ) ) ;
#3726=CARTESIAN_POINT ( 'NONE',  ( 104.4587341249999781, 81.12500000136559208, 1.846868145590721655 ) ) ;
#3739=CARTESIAN_POINT ( 'NONE',  ( 143.1451861577818079, 40.35507812608393863, -1.609821015232357215E-15 ) ) ;
#3740=CARTESIAN_POINT ( 'NONE',  ( 9.295050272127047819, 32.11992187608393579, 9.295050272127046043 ) ) ;
#3742=CARTESIAN_POINT ( 'NONE',  ( 55.40115559117954547, 38.51953124999999289, -9.598844408820458085 ) ) ;
#3744=CARTESIAN_POINT ( 'NONE',  ( 201.1066586549484896, 35.99999999999998579, 11.74215035806523488 ) ) ;
#3749=CARTESIAN_POINT ( 'NONE',  ( 104.4587341249999639, 81.18750000136559208, -1.442382525525748735E-14 ) ) ;
#3751=CARTESIAN_POINT ( 'NONE',  ( 5.444914386472302859, 39.41250000108393436, 13.14518615778179189 ) ) ;
#3752=CARTESIAN_POINT ( 'NONE',  ( 195.0000000000000000, -7.395377635281828788, -13.57481594606306707 ) ) ;
#3757=CARTESIAN_POINT ( 'NONE',  ( 99.99999999999995737, 85.00000000000000000, -1.387778780781445676E-14 ) ) ;
#3758=CARTESIAN_POINT ( 'NONE',  ( 65.00000000000000000, -7.395377635281828788, -7.517135062566165128E-15 ) ) ;
#3760=ADVANCED_FACE ( 'NONE', ( #1039 ), #18413, .T. ) ;
#3762=ORIENTED_EDGE ( 'NONE', *, *, #25973, .F. ) ;
#3763=CARTESIAN_POINT ( 'NONE',  ( 55.70494972787295751, 37.47773437608393010, -9.295050272127046043 ) ) ;
#3766=CARTESIAN_POINT ( 'NONE',  ( 189.5550856135277229, 32.16953125108393152, 13.14518615778179722 ) ) ;
#3768=CARTESIAN_POINT ( 'NONE',  ( 130.0000000000000000, 38.02343749999999289, 13.57481594606304576 ) ) ;
#3770=CIRCLE ( 'NONE', #15587, 11.57481594606304398 ) ;
#3771=ADVANCED_FACE ( 'NONE', ( #3590 ), #8131, .T. ) ;
#3772=CARTESIAN_POINT ( 'NONE',  ( 130.0000000000000000, 33.36015625216786873, 13.57481594606304576 ) ) ;
#3773=CARTESIAN_POINT ( 'NONE',  ( 185.4011555911795313, 40.90078124999999432, -9.598844408820458085 ) ) ;
#3775=CARTESIAN_POINT ( 'NONE',  ( 204.2950502721270425, 38.07304687608393579, -9.295050272127046043 ) ) ;
#3777=ORIENTED_EDGE ( 'NONE', *, *, #26938, .T. ) ;
#3783=LINE ( 'NONE', #25858, #15457 ) ;
#3784=CARTESIAN_POINT ( 'NONE',  ( 10.56308295035981182, 36.00000000000000000, 8.196709705857815109 ) ) ;
#3787=VECTOR ( 'NONE', #20153, 1000.000000000000000 ) ;
#3792=CARTESIAN_POINT ( 'NONE',  ( 120.7049497278729575, 31.72304687608393081, -9.295050272127046043 ) ) ;
#3793=CARTESIAN_POINT ( 'NONE',  ( 65.00000000000000000, 37.18007812608393436, -13.14518615778179544 ) ) ;
#3796=CARTESIAN_POINT ( 'NONE',  ( 9.295050272127047819, 36.08867187608392868, 9.295050272127046043 ) ) ;
#3797=CARTESIAN_POINT ( 'NONE',  ( 181.8258427830772916, 35.99999999999999289, 0.03826467346029673727 ) ) ;
#3799=CARTESIAN_POINT ( 'NONE',  ( -20.00000000000000000, 50.00000000000000000, 10.00000000000000178 ) ) ;
#3801=CARTESIAN_POINT ( 'NONE',  ( 13.14518615778179900, 38.51953125108393294, 5.444914386472293977 ) ) ;
#3802=CARTESIAN_POINT ( 'NONE',  ( 136.3519322287719717, 36.00000000000000000, 11.61660627739482621 ) ) ;
#3816=CARTESIAN_POINT ( 'NONE',  ( 95.54126587499995082, 80.37500000136562051, -1.846868145590750077 ) ) ;
#3817=CARTESIAN_POINT ( 'NONE',  ( 78.14518615778179367, 39.51171875108392584, 5.444914386472293977 ) ) ;
#3819=( BOUNDED_CURVE ( )  B_SPLINE_CURVE ( 2, ( #22835, #7564, #1451, #16258, #1177, #18820, #16682, #25381, #9843 ),
 .UNSPECIFIED., .F., .F. ) 
 B_SPLINE_CURVE_WITH_KNOTS ( ( 3, 2, 2, 2, 3 ),
 ( 0.1041666666666664909, 0.1145833333333332732, 0.1250000000000000833, 0.1354166666666668517, 0.1458333333333336757 ),
 .UNSPECIFIED. ) 
 CURVE ( )  GEOMETRIC_REPRESENTATION_ITEM ( )  RATIONAL_B_SPLINE_CURVE ( ( 1.000000000000001332, 0.9238795325112854062, 1.000000000000000000, 0.9238795325112867385, 1.000000000000000000, 0.9238795325112867385, 1.000000000000000000, 0.9238795325112842960, 1.000000000000002442 ) ) 
 REPRESENTATION_ITEM ( '' )  );
#3823=CARTESIAN_POINT ( 'NONE',  ( 116.4251840539369454, 39.36289062499999858, -5.622872871577873077 ) ) ;
#3825=CARTESIAN_POINT ( 'NONE',  ( -1.501019124304961982, 53.60014735326988244, -14.99999999999999822 ) ) ;
#3828=CARTESIAN_POINT ( 'NONE',  ( 139.2950502721270425, 39.46210937608393010, -9.295050272127046043 ) ) ;
#3829=CARTESIAN_POINT ( 'NONE',  ( 74.59884440882045453, 36.83281250216787583, -9.598844408820458085 ) ) ;
#3831=CARTESIAN_POINT ( 'NONE',  ( -9.598844408820458085, 36.23750000216787726, -9.598844408820458085 ) ) ;
#3836=CARTESIAN_POINT ( 'NONE',  ( 200.4449143864723055, 36.33671875108394289, -13.14518615778179900 ) ) ;
#3838=CARTESIAN_POINT ( 'NONE',  ( 124.5550856135277087, 36.73359375108393010, 13.14518615778179722 ) ) ;
#3841=CARTESIAN_POINT ( 'NONE',  ( 130.0000000000000000, 37.62656249999999858, -13.57481594606304576 ) ) ;
#3845=CARTESIAN_POINT ( 'NONE',  ( 204.5988444088204687, 38.91640624999999432, 9.598844408820456309 ) ) ;
#3849=CARTESIAN_POINT ( 'NONE',  ( 55.70494972787295751, 38.27148437608393294, 9.295050272127047819 ) ) ;
#3854=CARTESIAN_POINT ( 'NONE',  ( -9.598844408820454532, 39.51171874999999289, 9.598844408820459861 ) ) ;
#3857=CARTESIAN_POINT ( 'NONE',  ( 101.8468681455906903, 82.00000000136560629, 4.458734124999987891 ) ) ;
#3860=EDGE_LOOP ( 'NONE', ( #20155, #26876, #23303 ) ) ;
#3861=( BOUNDED_CURVE ( )  B_SPLINE_CURVE ( 2, ( #24797, #22525, #5804, #3664, #14606, #7544, #21182, #1664, #6075 ),
 .UNSPECIFIED., .F., .T. ) 
 B_SPLINE_CURVE_WITH_KNOTS ( ( 3, 2, 2, 2, 3 ),
 ( 0.4791666666666667962, 0.4895833333333333703, 0.5000000000000000000, 0.5104166666666665186, 0.5208333333333332593 ),
 .UNSPECIFIED. ) 
 CURVE ( )  GEOMETRIC_REPRESENTATION_ITEM ( )  RATIONAL_B_SPLINE_CURVE ( ( 0.9999999999999992228, 0.9238795325112875156, 1.000000000000000000, 0.9238795325112867385, 1.000000000000000000, 0.9238795325112867385, 1.000000000000000000, 0.9238795325112875156, 0.9999999999999992228 ) ) 
 REPRESENTATION_ITEM ( '' )  );
#3869=CARTESIAN_POINT ( 'NONE',  ( 181.4251840539369596, 38.76757812716787299, 5.622872871577880183 ) ) ;
#3872=CARTESIAN_POINT ( 'NONE',  ( 190.4284083674847636, 51.44262710532314742, 15.00000000000126654 ) ) ;
#3873=CARTESIAN_POINT ( 'NONE',  ( 116.8548138422182205, 40.75195312608393294, 0.000000000000000000 ) ) ;
#3874=CARTESIAN_POINT ( 'NONE',  ( -5.444914386472299306, 33.55859375108393294, 13.14518615778179722 ) ) ;
#3876=AXIS2_PLACEMENT_3D ( 'NONE', #21322, #21044, #18763 ) ;
#3877=VERTEX_POINT ( 'NONE', #25792 ) ;
#3878=CARTESIAN_POINT ( 'NONE',  ( 65.00000000000000000, 37.62656249999999858, -13.57481594606304576 ) ) ;
#3884=CARTESIAN_POINT ( 'NONE',  ( 104.4587341249999639, 83.18750000136560629, -1.442382525525748735E-14 ) ) ;
#3886=CARTESIAN_POINT ( 'NONE',  ( -8.049105076161786076E-16, 38.96601562608393721, -13.14518615778179544 ) ) ;
#3887=FACE_OUTER_BOUND ( 'NONE', #9286, .T. ) ;
#3888=ORIENTED_EDGE ( 'NONE', *, *, #440, .T. ) ;
#3890=DIRECTION ( 'NONE',  ( 0.000000000000000000, 0.000000000000000000, 1.000000000000000000 ) ) ;
#3897=CARTESIAN_POINT ( 'NONE',  ( 74.29505027212704249, 38.07304687608393579, -9.295050272127046043 ) ) ;
#3900=EDGE_CURVE ( 'NONE', #21810, #18157, #27942, .T. ) ;
#3903=CARTESIAN_POINT ( 'NONE',  ( -3.979814445820054392, 50.00000000123264954, -13.01613927312573793 ) ) ;
#3904=AXIS2_PLACEMENT_3D ( 'NONE', #10327, #25180, #21720 ) ;
#3906=CARTESIAN_POINT ( 'NONE',  ( 143.5748159460630404, 34.40195312716787157, -5.622872871577873077 ) ) ;
#3907=CARTESIAN_POINT ( 'NONE',  ( 51.85481384221820633, 40.00781250108393294, 5.444914386472304635 ) ) ;
#3909=CARTESIAN_POINT ( 'NONE',  ( -18.00000000000000711, 78.00000000000000000, -12.99999999999999822 ) ) ;
#3910=CARTESIAN_POINT ( 'NONE',  ( 208.1451861577818079, 37.97382812608393721, -1.609821015232357215E-15 ) ) ;
#3911=ORIENTED_EDGE ( 'NONE', *, *, #26252, .T. ) ;
#3912=ORIENTED_EDGE ( 'NONE', *, *, #27435, .F. ) ;
#3918=CARTESIAN_POINT ( 'NONE',  ( 13.57481594606304931, 38.17226562499999432, 5.622872871577868636 ) ) ;
#3919=ADVANCED_FACE ( 'NONE', ( #19066 ), #23048, .T. ) ;
#3927=CARTESIAN_POINT ( 'NONE',  ( 143.5748159460630404, 32.61601562499999574, 5.622872871577869525 ) ) ;
#3929=ORIENTED_EDGE ( 'NONE', *, *, #17022, .T. ) ;
#3933=CARTESIAN_POINT ( 'NONE',  ( 120.7049497278729575, 40.05742187608393579, 9.295050272127047819 ) ) ;
#3934=CARTESIAN_POINT ( 'NONE',  ( 55.70494972787295751, 36.48554687608393721, -9.295050272127046043 ) ) ;
#3935=CARTESIAN_POINT ( 'NONE',  ( 185.7049497278729575, 32.51679687608393721, -9.295050272127046043 ) ) ;
#3937=CARTESIAN_POINT ( 'NONE',  ( 9.295050272127047819, 36.88242187608393152, 9.295050272127046043 ) ) ;
#3938=CARTESIAN_POINT ( 'NONE',  ( 195.3745404134769785, 35.99999999999998579, -13.51869779562198381 ) ) ;
#3940=CARTESIAN_POINT ( 'NONE',  ( 189.4309414480975704, 36.00000000000000000, 11.91493531101289882 ) ) ;
#3943=CARTESIAN_POINT ( 'NONE',  ( 5.444914386472302859, 39.21406250108392300, 13.14518615778179189 ) ) ;
#3945=CARTESIAN_POINT ( 'NONE',  ( -7.623941961925451594, 55.00000000000000000, 14.99999999999999645 ) ) ;
#3947=CARTESIAN_POINT ( 'NONE',  ( 130.0000000000000000, -7.395377635281828788, -1.503427012513233026E-14 ) ) ;
#3951=CARTESIAN_POINT ( 'NONE',  ( 130.0000000000000000, 38.51953125216787299, -13.57481594606304576 ) ) ;
#3959=CARTESIAN_POINT ( 'NONE',  ( 101.8468681455906903, 80.12500000136560629, -4.458734125000016313 ) ) ;
#3960=CARTESIAN_POINT ( 'NONE',  ( 65.00000000000000000, 38.17226562608394147, -13.14518615778179544 ) ) ;
#3962=CARTESIAN_POINT ( 'NONE',  ( -8.049105076161786076E-16, 40.35507812608393152, -13.14518615778179544 ) ) ;
#3965=CARTESIAN_POINT ( 'NONE',  ( 59.37712712842218110, 38.56914062716787583, -13.57481594606310260 ) ) ;
#3967=CARTESIAN_POINT ( 'NONE',  ( 130.0000000000000000, 31.82226562608393650, -13.14518615778179544 ) ) ;
#3968=ORIENTED_EDGE ( 'NONE', *, *, #11866, .F. ) ;
#3970=CYLINDRICAL_SURFACE ( 'NONE', #27177, 13.57481594606304398 ) ;
#3971=CARTESIAN_POINT ( 'NONE',  ( 99.99999999999995737, 81.18750000136559208, -4.458734125000016313 ) ) ;
#3972=CARTESIAN_POINT ( 'NONE',  ( 143.1451861577818079, 40.10703125108393152, 5.444914386472293977 ) ) ;
#3973=CARTESIAN_POINT ( 'NONE',  ( 59.37712712842213136, 38.56914062716788294, -13.57481594606304753 ) ) ;
#3975=CARTESIAN_POINT ( 'NONE',  ( 5.622872871577878406, 34.99726562716787726, 13.57481594606304576 ) ) ;
#3976=VERTEX_POINT ( 'NONE', #6137 ) ;
#3978=ORIENTED_EDGE ( 'NONE', *, *, #26236, .F. ) ;
#3979=CARTESIAN_POINT ( 'NONE',  ( 195.0000000000000000, 35.98945312608393010, 13.14518615778179544 ) ) ;
#3982=CARTESIAN_POINT ( 'NONE',  ( 124.5550856135277087, 37.22968750108394431, -13.14518615778179722 ) ) ;
#3984=DIRECTION ( 'NONE',  ( 0.000000000000000000, -2.775557561562890720E-14, -1.000000000000000000 ) ) ;
#3986=LINE ( 'NONE', #23782, #5722 ) ;
#3987=( BOUNDED_CURVE ( )  B_SPLINE_CURVE ( 2, ( #14435, #3627, #5766, #16993, #25693, #6176, #16442, #9885, #23565 ),
 .UNSPECIFIED., .F., .T. ) 
 B_SPLINE_CURVE_WITH_KNOTS ( ( 3, 2, 2, 2, 3 ),
 ( 0.1458333333333336757, 0.1562500000000002776, 0.1666666666666669072, 0.1770833333333335369, 0.1875000000000001388 ),
 .UNSPECIFIED. ) 
 CURVE ( )  GEOMETRIC_REPRESENTATION_ITEM ( )  RATIONAL_B_SPLINE_CURVE ( ( 0.9999999999999975575, 0.9238795325112891810, 1.000000000000000000, 0.9238795325112867385, 1.000000000000000000, 0.9238795325112867385, 1.000000000000000000, 0.9238795325112857393, 1.000000000000001110 ) ) 
 REPRESENTATION_ITEM ( '' )  );
#3989=CARTESIAN_POINT ( 'NONE',  ( 181.4251840539369596, 36.28710937499999289, 5.622872871577880183 ) ) ;
#3993=CARTESIAN_POINT ( 'NONE',  ( 78.14518615778179367, 38.61875000108393152, -5.444914386472297529 ) ) ;
#3998=CARTESIAN_POINT ( 'NONE',  ( -8.312177448680279460E-16, 38.42031249999999432, -13.57481594606304576 ) ) ;
#4001=CARTESIAN_POINT ( 'NONE',  ( 101.8468681455906903, 84.00000000136560629, 4.458734124999987891 ) ) ;
#4003=VERTEX_POINT ( 'NONE', #1218 ) ;
#4005=CARTESIAN_POINT ( 'NONE',  ( 55.70494972787295751, 35.29492187608393294, 9.295050272127047819 ) ) ;
#4006=ORIENTED_EDGE ( 'NONE', *, *, #12484, .T. ) ;
#4010=FACE_OUTER_BOUND ( 'NONE', #7858, .T. ) ;
#4012=CARTESIAN_POINT ( 'NONE',  ( 200.6228728715778686, 38.17226562716786731, 13.57481594606304576 ) ) ;
#4014=CARTESIAN_POINT ( 'NONE',  ( 130.0000000000000000, 36.00000000000000000, -1.503427012513233026E-14 ) ) ;
#4015=CARTESIAN_POINT ( 'NONE',  ( 204.1801758136480203, 55.00000000000000711, 14.99999999999994671 ) ) ;
#4016=CARTESIAN_POINT ( 'NONE',  ( 120.7049497278729575, 39.06523437608392868, -9.295050272127046043 ) ) ;
#4017=CARTESIAN_POINT ( 'NONE',  ( 13.14518615778179900, 39.61093750108393863, -5.444914386472297529 ) ) ;
#4018=ORIENTED_EDGE ( 'NONE', *, *, #26747, .F. ) ;
#4019=CARTESIAN_POINT ( 'NONE',  ( 74.59884440882045453, 37.32890624999999574, 9.598844408820456309 ) ) ;
#4023=CARTESIAN_POINT ( 'NONE',  ( 198.3041185978229350, 36.00000000000001421, 12.77244747738234487 ) ) ;
#4028=CARTESIAN_POINT ( 'NONE',  ( 96.84719886470459471, 79.81250000136559208, 3.152801135295355994 ) ) ;
#4030=CARTESIAN_POINT ( 'NONE',  ( 9.295050272127047819, 40.25585937608393294, 9.295050272127046043 ) ) ;
#4036=CARTESIAN_POINT ( 'NONE',  ( 99.99999999999995737, 82.37500000273119838, 4.999999999999990230 ) ) ;
#4038=EDGE_CURVE ( 'NONE', #4887, #506, #27532, .T. ) ;
#4039=CARTESIAN_POINT ( 'NONE',  ( 189.5550856135277229, 39.61093750108393152, -13.14518615778179900 ) ) ;
#4041=CARTESIAN_POINT ( 'NONE',  ( 78.14518615778180788, 37.22968750108394431, -5.444914386472297529 ) ) ;
#4042=DIRECTION ( 'NONE',  ( 0.000000000000000000, -1.000000000000000000, 0.000000000000000000 ) ) ;
#4043=CIRCLE ( 'NONE', #10389, 5.000000000000004441 ) ;
#4046=ORIENTED_EDGE ( 'NONE', *, *, #14668, .F. ) ;
#4048=CARTESIAN_POINT ( 'NONE',  ( -1.505492181556997933, 53.60078691996342570, -14.99999999999999645 ) ) ;
#4051=CARTESIAN_POINT ( 'NONE',  ( 143.5748159460630688, 34.35234375216787583, -1.662435489736055892E-15 ) ) ;
#4052=FACE_OUTER_BOUND ( 'NONE', #786, .T. ) ;
#4054=CARTESIAN_POINT ( 'NONE',  ( 195.0000000000000000, 35.39414062608393863, 13.14518615778179544 ) ) ;
#4055=ORIENTED_EDGE ( 'NONE', *, *, #24116, .T. ) ;
#4059=CARTESIAN_POINT ( 'NONE',  ( 70.44491438647229131, 40.00781250108393294, 13.14518615778179189 ) ) ;
#4060=CARTESIAN_POINT ( 'NONE',  ( 101.8468681455907046, 80.75000000136560629, 4.458734124999987891 ) ) ;
#4061=DIRECTION ( 'NONE',  ( -1.000000000000000000, 0.000000000000000000, 7.228014483236696740E-18 ) ) ;
#4065=CYLINDRICAL_SURFACE ( 'NONE', #12103, 5.000000000000004441 ) ;
#4067=CARTESIAN_POINT ( 'NONE',  ( 181.8548138422182205, 40.00781250108393294, 5.444914386472304635 ) ) ;
#4068=CARTESIAN_POINT ( 'NONE',  ( 137.1713912169990124, 31.99955315621561525, -11.52591757658528948 ) ) ;
#4073=CARTESIAN_POINT ( 'NONE',  ( 130.0000000000000000, 36.18789062608393436, 13.14518615778179544 ) ) ;
#4074=CARTESIAN_POINT ( 'NONE',  ( 74.29505027212704249, 36.28710937608393294, -9.295050272127046043 ) ) ;
#4075=CARTESIAN_POINT ( 'NONE',  ( 181.8548138422181921, 31.87187500108393223, 5.444914386472304635 ) ) ;
#4076=ADVANCED_FACE ( 'NONE', ( #19380 ), #25794, .T. ) ;
#4077=CARTESIAN_POINT ( 'NONE',  ( 65.00000000000000000, 52.00000000000000711, 11.57481594606303688 ) ) ;
#4078=CARTESIAN_POINT ( 'NONE',  ( -5.444914386472297529, 34.84843750108393579, -13.14518615778179900 ) ) ;
#4082=CARTESIAN_POINT ( 'NONE',  ( 5.444914386472297529, 39.51171875108392584, -13.14518615778179900 ) ) ;
#4083=DIRECTION ( 'NONE',  ( 1.000000000000000000, 1.387778780781445478E-15, 0.000000000000000000 ) ) ;
#4085=CARTESIAN_POINT ( 'NONE',  ( 60.93741645942577634, 50.00000000116062182, 12.98908657125237376 ) ) ;
#4092=B_SPLINE_CURVE_WITH_KNOTS ( 'NONE', 3,
 ( #22896, #18879, #1240, #8190, #1515, #12582, #7778, #27730, #27451, #5788, #25445, #14593, #17012, #23312, #9903, #3784, #25716, #23035, #14728, #10039, #16745, #5926, #1649, #14455, #21168, #7912, #20755, #16465, #12442, #10309, #19016 ),
 .UNSPECIFIED., .F., .F.,
 ( 4, 2, 2, 2, 2, 2, 2, 2, 2, 2, 1, 2, 2, 2, 2, 4 ),
 ( 0.000000000000000000, 0.001647793485000534136, 0.003295586970001068271, 0.004943380455001602190, 0.005767277197501870234, 0.006591173940002139145, 0.008238967425002673498, 0.009886760910003206115, 0.01318234788000428176, 0.01483014136500482132, 0.01647793485000536087, 0.01812572833500590216, 0.01977352182000643999, 0.02306910879000751910, 0.02471690227500805692, 0.02636469576000859821 ),
 .UNSPECIFIED. ) ;
#4096=CARTESIAN_POINT ( 'NONE',  ( 95.54126587499996504, 83.68750000136560629, -1.387778780781445676E-14 ) ) ;
#4097=CARTESIAN_POINT ( 'NONE',  ( 78.14518615778179367, 39.56132812608393579, -1.609821015232357215E-15 ) ) ;
#4099=CARTESIAN_POINT ( 'NONE',  ( 13.14518615778179722, 40.20625000108393010, -5.444914386472297529 ) ) ;
#4103=CARTESIAN_POINT ( 'NONE',  ( 130.0000000000000000, 40.00781250000000000, -13.57481594606304576 ) ) ;
#4105=CARTESIAN_POINT ( 'NONE',  ( 1.662435489736055498E-15, -7.395377635281828788, -13.57481594606304398 ) ) ;
#4108=CARTESIAN_POINT ( 'NONE',  ( 124.5550856135277087, 36.73359375108393010, 13.14518615778179722 ) ) ;
#4109=EDGE_CURVE ( 'NONE', #15719, #3050, #14153, .T. ) ;
#4110=CARTESIAN_POINT ( 'NONE',  ( 51.42518405393695957, 37.13046875216787868, 0.000000000000000000 ) ) ;
#4112=CARTESIAN_POINT ( 'NONE',  ( -9.598844408820454532, 37.22968750216787726, 9.598844408820459861 ) ) ;
#4113=EDGE_CURVE ( 'NONE', #9852, #16430, #11364, .T. ) ;
#4116=CARTESIAN_POINT ( 'NONE',  ( 200.4449143864723055, 36.83281250108392868, 13.14518615778179189 ) ) ;
#4119=CARTESIAN_POINT ( 'NONE',  ( 135.4449143864723339, 39.51171875108393294, -13.14518615778179722 ) ) ;
#4121=DIRECTION ( 'NONE',  ( -0.000000000000000000, -0.000000000000000000, 1.000000000000000000 ) ) ;
#4122=DIRECTION ( 'NONE',  ( 0.000000000000000000, -1.000000000000000000, 0.000000000000000000 ) ) ;
#4126=CARTESIAN_POINT ( 'NONE',  ( 181.4251840539369596, 37.82499999999999574, 0.000000000000000000 ) ) ;
#4129=CARTESIAN_POINT ( 'NONE',  ( 59.55508561352770158, 37.52734375108393294, 13.14518615778179722 ) ) ;
#4132=FACE_OUTER_BOUND ( 'NONE', #19605, .T. ) ;
#4135=CARTESIAN_POINT ( 'NONE',  ( -8.312177448680279460E-16, 40.80156249999999574, -13.57481594606304576 ) ) ;
#4136=CARTESIAN_POINT ( 'NONE',  ( 135.4449143864723055, 40.20625000108394431, 13.14518615778179189 ) ) ;
#4137=ORIENTED_EDGE ( 'NONE', *, *, #26047, .T. ) ;
#4138=CARTESIAN_POINT ( 'NONE',  ( 96.46446609406721961, 84.87500000000000000, -3.535533905932755072 ) ) ;
#4141=VERTEX_POINT ( 'NONE', #1427 ) ;
#4142=DIRECTION ( 'NONE',  ( 0.000000000000000000, -1.000000000000000000, -0.000000000000000000 ) ) ;
#4143=CARTESIAN_POINT ( 'NONE',  ( 55.70494972787295751, 36.08867187608393579, 9.295050272127047819 ) ) ;
#4144=( BOUNDED_CURVE ( )  B_SPLINE_CURVE ( 2, ( #10791, #21092, #14651, #17216, #6526, #25776, #1581, #6255, #10653 ),
 .UNSPECIFIED., .F., .T. ) 
 B_SPLINE_CURVE_WITH_KNOTS ( ( 3, 2, 2, 2, 3 ),
 ( 0.3958333333333331483, 0.4062499999999999445, 0.4166666666666667407, 0.4270833333333335369, 0.4375000000000003331 ),
 .UNSPECIFIED. ) 
 CURVE ( )  GEOMETRIC_REPRESENTATION_ITEM ( )  RATIONAL_B_SPLINE_CURVE ( ( 1.000000000000001110, 0.9238795325112855172, 1.000000000000000000, 0.9238795325112867385, 1.000000000000000000, 0.9238795325112867385, 1.000000000000000000, 0.9238795325112842960, 1.000000000000002442 ) ) 
 REPRESENTATION_ITEM ( '' )  );
#4145=VERTEX_POINT ( 'NONE', #10085 ) ;
#4148=AXIS2_PLACEMENT_3D ( 'NONE', #21012, #3482, #12146 ) ;
#4153=CARTESIAN_POINT ( 'NONE',  ( 181.4251840539369596, 36.28710937716787299, -5.622872871577873077 ) ) ;
#4155=DIRECTION ( 'NONE',  ( 0.000000000000000000, -0.000000000000000000, 1.000000000000000000 ) ) ;
#4157=CARTESIAN_POINT ( 'NONE',  ( 130.0000000000000000, 38.56914062608393579, 13.14518615778179544 ) ) ;
#4158=CARTESIAN_POINT ( 'NONE',  ( 9.295050272127047819, 39.46210937608393721, 9.295050272127046043 ) ) ;
#4159=VECTOR ( 'NONE', #12298, 1000.000000000000000 ) ;
#4160=CARTESIAN_POINT ( 'NONE',  ( 130.0000000000000000, 34.40195312608393152, 13.14518615778179544 ) ) ;
#4161=CARTESIAN_POINT ( 'NONE',  ( 74.59884440882045453, 36.73359374999999716, -9.598844408820458085 ) ) ;
#4170=CARTESIAN_POINT ( 'NONE',  ( 13.14518615778179544, 40.35507812608393863, -1.609821015232357215E-15 ) ) ;
#4176=CARTESIAN_POINT ( 'NONE',  ( 185.7049497278729575, 38.86679687608393863, -9.295050272127046043 ) ) ;
#4178=CARTESIAN_POINT ( 'NONE',  ( 142.0772764098356333, 36.00000000000000711, -6.197985357349214297 ) ) ;
#4185=CARTESIAN_POINT ( 'NONE',  ( 135.6228728715778686, 34.50117187716788436, -13.57481594606304753 ) ) ;
#4188=CARTESIAN_POINT ( 'NONE',  ( 181.8548138422182205, 35.98945312608393721, 0.000000000000000000 ) ) ;
#4190=ADVANCED_FACE ( 'NONE', ( #16926 ), #14774, .T. ) ;
#4191=( BOUNDED_CURVE ( )  B_SPLINE_CURVE ( 2, ( #8750, #2354, #26140, #23863, #21590, #15291, #19445, #352, #24008, #11009, #19722, #17731, #6199, #14869, #23583, #4067, #12729, #21453, #1931, #10599, #19307, #8471, #17158, #24285, #20446, #13428, #13719, #14004, #927, #24717, #16149, #3053, #9312, #24857, #22156, #20158, #9739, #6892, #17871, #7166, #4766, #9598, #11720, #15863, #24573, #13575, #26433, #9178, #26576, #639, #18300, #22727, #26720, #2634, #11864, #7455, #3193, #2774, #9454, #7025, #2908, #5195, #11577, #18010, #15723, #5054, #24426, #20587, #22299, #26868, #7314, #22441, #20297, #27008, #784, #5338, #18154, #4915, #16003, #13859, #1070, #15578, #22585, #11294, #20017, #497, #11438, #5477, #25555, #14427, #18992, #27290, #16856, #16434, #20865, #3334, #27701 ),
 .UNSPECIFIED., .F., .T. ) 
 B_SPLINE_CURVE_WITH_KNOTS ( ( 3, 2, 2, 2, 2, 2, 2, 2, 2, 2, 2, 2, 2, 2, 2, 2, 2, 2, 2, 2, 2, 2, 2, 2, 2, 2, 2, 2, 2, 2, 2, 2, 2, 2, 2, 2, 2, 2, 2, 2, 2, 2, 2, 2, 2, 2, 2, 2, 3 ),
 ( 0.000000000000000000, 0.01041666666666666609, 0.02083333333333333218, 0.03125000000000000000, 0.04166666666666666435, 0.05208333333333333565, 0.06250000000000000000, 0.07291666666666667129, 0.08333333333333332871, 0.09374999999999998612, 0.1041666666666666713, 0.1145833333333333287, 0.1250000000000000000, 0.1354166666666666574, 0.1458333333333333426, 0.1562500000000000000, 0.1666666666666666574, 0.1770833333333333426, 0.1874999999999999722, 0.1979166666666666574, 0.2083333333333333426, 0.2187500000000000000, 0.2291666666666666574, 0.2395833333333333426, 0.2500000000000000000, 0.2604166666666666852, 0.2708333333333333148, 0.2812500000000000000, 0.2916666666666666852, 0.3020833333333333148, 0.3125000000000000000, 0.3229166666666666852, 0.3333333333333333148, 0.3437500000000000000, 0.3541666666666666852, 0.3645833333333333148, 0.3749999999999999445, 0.3854166666666666852, 0.3958333333333333148, 0.4062500000000000000, 0.4166666666666666852, 0.4270833333333333148, 0.4375000000000000000, 0.4479166666666666852, 0.4583333333333333148, 0.4687500000000000000, 0.4791666666666666852, 0.4895833333333333148, 0.4988304892921909817 ),
 .UNSPECIFIED. ) 
 CURVE ( )  GEOMETRIC_REPRESENTATION_ITEM ( )  RATIONAL_B_SPLINE_CURVE ( ( 1.000000000000000000, 0.9238795325112867385, 1.000000000000000000, 0.9238795325112867385, 1.000000000000000000, 0.9238795325112867385, 1.000000000000000000, 0.9238795325112867385, 1.000000000000000000, 0.9238795325112867385, 1.000000000000000000, 0.9238795325112867385, 1.000000000000000000, 0.9238795325112867385, 1.000000000000000000, 0.9238795325112867385, 1.000000000000000000, 0.9238795325112867385, 1.000000000000000000, 0.9238795325112867385, 1.000000000000000000, 0.9238795325112867385, 1.000000000000000000, 0.9238795325112867385, 1.000000000000000000, 0.9238795325112867385, 1.000000000000000000, 0.9238795325112867385, 1.000000000000000000, 0.9238795325112867385, 1.000000000000000000, 0.9238795325112867385, 1.000000000000000000, 0.9238795325112867385, 1.000000000000000000, 0.9238795325112867385, 1.000000000000000000, 0.9238795325112867385, 1.000000000000000000, 0.9238795325112867385, 1.000000000000000000, 0.9238795325112867385, 1.000000000000000000, 0.9238795325112867385, 1.000000000000000000, 0.9238795325112867385, 1.000000000000000000, 0.9238795325112867385, 1.000000000000000000, 0.9238795325112867385, 1.000000000000000000, 0.9238795325112867385, 1.000000000000000000, 0.9238795325112867385, 1.000000000000000000, 0.9238795325112867385, 1.000000000000000000, 0.9238795325112867385, 1.000000000000000000, 0.9238795325112867385, 1.000000000000000000, 0.9238795325112867385, 1.000000000000000000, 0.9238795325112867385, 1.000000000000000000, 0.9238795325112867385, 1.000000000000000000, 0.9238795325112867385, 1.000000000000000000, 0.9238795325112867385, 1.000000000000000000, 0.9238795325112867385, 1.000000000000000000, 0.9238795325112867385, 1.000000000000000000, 0.9238795325112867385, 1.000000000000000000, 0.9238795325112867385, 1.000000000000000000, 0.9238795325112867385, 1.000000000000000000, 0.9238795325112867385, 1.000000000000000000, 0.9238795325112867385, 1.000000000000000000, 0.9238795325112867385, 1.000000000000000000, 0.9238795325112867385, 1.000000000000000000, 0.9238795325112867385, 1.000000000000000000, 0.9238795325112867385, 1.000000000000000000, 0.9238795325112867385, 1.000000000000000000, 0.9324258078851886955, 0.9848264816800353927 ) ) 
 REPRESENTATION_ITEM ( '' )  );
#4195=CARTESIAN_POINT ( 'NONE',  ( 97.92893218813451028, 83.81250000000001421, -5.000000000000031974 ) ) ;
#4197=CARTESIAN_POINT ( 'NONE',  ( 101.8468681455907046, 81.75000000136560629, 4.458734124999987891 ) ) ;
#4198=CARTESIAN_POINT ( 'NONE',  ( 185.7049497278729575, 37.47773437608393010, 9.295050272127047819 ) ) ;
#4201=PLANE ( 'NONE',  #22590 ) ;
#4203=CARTESIAN_POINT ( 'NONE',  ( 130.0000000000000000, 32.46718749999999432, 13.57481594606304576 ) ) ;
#4208=CARTESIAN_POINT ( 'NONE',  ( 116.8548138422182063, 35.14609375108393152, -5.444914386472297529 ) ) ;
#4209=CARTESIAN_POINT ( 'NONE',  ( 51.85481384221820633, 34.99726562608393721, 0.000000000000000000 ) ) ;
#4211=CARTESIAN_POINT ( 'NONE',  ( 189.5550856135277229, 36.13828125108393863, 13.14518615778179722 ) ) ;
#4212=ORIENTED_EDGE ( 'NONE', *, *, #16018, .F. ) ;
#4214=CARTESIAN_POINT ( 'NONE',  ( 13.14518615778179900, 34.65000000108393152, -5.444914386472297529 ) ) ;
#4215=CARTESIAN_POINT ( 'NONE',  ( 133.7165341137897201, 51.46663580899082291, -14.99999999999932143 ) ) ;
#4218=CARTESIAN_POINT ( 'NONE',  ( -13.14518615778179189, 38.22187500108393010, 5.444914386472304635 ) ) ;
#4224=CARTESIAN_POINT ( 'NONE',  ( 77.32011696698889125, 36.00000000000002132, -5.704949255836485378 ) ) ;
#4228=CARTESIAN_POINT ( 'NONE',  ( 121.7314026716134379, 50.00000000054362914, 10.78867689284450826 ) ) ;
#4231=CARTESIAN_POINT ( 'NONE',  ( 181.6399989480775901, 40.87597656304196647, 0.000000000000000000 ) ) ;
#4232=CARTESIAN_POINT ( 'NONE',  ( 103.1528011352953342, 82.31250000136559208, -3.152801135295383084 ) ) ;
#4233=CARTESIAN_POINT ( 'NONE',  ( 65.00000000000000000, 34.60039062608393579, 13.14518615778179544 ) ) ;
#4235=CARTESIAN_POINT ( 'NONE',  ( 185.8198241863519797, 50.00000000000000000, -9.999999999999991118 ) ) ;
#4236=DIRECTION ( 'NONE',  ( 0.000000000000000000, 0.000000000000000000, 1.000000000000000000 ) ) ;
#4238=CARTESIAN_POINT ( 'NONE',  ( 102.0710678118654329, 82.68750000000000000, -4.999999999999992006 ) ) ;
#4239=CARTESIAN_POINT ( 'NONE',  ( 143.5748159460630404, 39.85898437499999858, -5.622872871577873077 ) ) ;
#4244=CARTESIAN_POINT ( 'NONE',  ( 139.2950502721270425, 35.29492187608393294, 9.295050272127046043 ) ) ;
#4245=CARTESIAN_POINT ( 'NONE',  ( 78.57481594606305464, 37.52734375216787299, -1.662435489736055892E-15 ) ) ;
#4247=CARTESIAN_POINT ( 'NONE',  ( -5.622872871577873077, 36.18789062716787441, -13.57481594606304753 ) ) ;
#4251=EDGE_CURVE ( 'NONE', #8417, #27733, #21046, .T. ) ;
#4252=CARTESIAN_POINT ( 'NONE',  ( 185.7049497278729575, 38.07304687608393579, -9.295050272127046043 ) ) ;
#4253=CARTESIAN_POINT ( 'NONE',  ( 78.57481594606305464, 39.01562500000000000, -1.662435489736055892E-15 ) ) ;
#4258=DIRECTION ( 'NONE',  ( -0.000000000000000000, 1.000000000000000000, -0.000000000000000000 ) ) ;
#4262=CARTESIAN_POINT ( 'NONE',  ( 189.3771271284221314, 34.50117187499999005, -13.57481594606304753 ) ) ;
#4265=CARTESIAN_POINT ( 'NONE',  ( 51.85481384221819923, 37.32890625108393579, -5.444914386472297529 ) ) ;
#4268=PLANE ( 'NONE',  #13187 ) ;
#4271=CARTESIAN_POINT ( 'NONE',  ( 13.57481594606304753, 35.89023437499999858, -5.622872871577873077 ) ) ;
#4274=ORIENTED_EDGE ( 'NONE', *, *, #24347, .T. ) ;
#4275=CARTESIAN_POINT ( 'NONE',  ( 99.99999999999995737, 80.43750000136559208, -4.458734125000016313 ) ) ;
#4276=VECTOR ( 'NONE', #3249, 1000.000000000000227 ) ;
#4281=CARTESIAN_POINT ( 'NONE',  ( 51.85481384221819923, 33.55859375108393294, -5.444914386472297529 ) ) ;
#4283=CARTESIAN_POINT ( 'NONE',  ( 129.2802394038908176, 53.51499872091922327, -15.00000000000000000 ) ) ;
#4286=CARTESIAN_POINT ( 'NONE',  ( 97.92893218813449607, 82.31250000273122680, 4.999999999999968914 ) ) ;
#4288=CARTESIAN_POINT ( 'NONE',  ( 204.5988444088204687, 38.22187500216787015, 9.598844408820456309 ) ) ;
#4290=CARTESIAN_POINT ( 'NONE',  ( 65.00000000000000000, 38.81718749999999574, 13.57481594606304576 ) ) ;
#4291=CARTESIAN_POINT ( 'NONE',  ( 191.2834658862103936, 51.46663580899083001, 14.99999999999791989 ) ) ;
#4293=CARTESIAN_POINT ( 'NONE',  ( 208.5748159460630688, 39.85898437716787157, 5.622872871577868636 ) ) ;
#4294=VERTEX_POINT ( 'NONE', #24332 ) ;
#4295=CARTESIAN_POINT ( 'NONE',  ( -13.14518615778179544, 36.78320312608393294, 0.000000000000000000 ) ) ;
#4296=CARTESIAN_POINT ( 'NONE',  ( 116.8548138422182063, 35.04687500108393294, 5.444914386472304635 ) ) ;
#4297=CARTESIAN_POINT ( 'NONE',  ( 65.00000000000000000, 35.24531249999999716, -13.57481594606304576 ) ) ;
#4301=CARTESIAN_POINT ( 'NONE',  ( 199.8599772695822878, 36.00000000000001421, 12.29462155906273502 ) ) ;
#4302=AXIS2_PLACEMENT_3D ( 'NONE', #7000, #15694, #24688 ) ;
#4307=DIRECTION ( 'NONE',  ( 0.000000000000000000, 0.000000000000000000, -1.000000000000000000 ) ) ;
#4309=CARTESIAN_POINT ( 'NONE',  ( -13.14518615778179900, 40.70234375108393721, -5.444914386472297529 ) ) ;
#4312=EDGE_LOOP ( 'NONE', ( #15865, #11332, #4570, #17656 ) ) ;
#4313=( BOUNDED_CURVE ( )  B_SPLINE_CURVE ( 2, ( #27249, #15962, #5583, #27109, #22686, #11680, #3156, #16399, #12235 ),
 .UNSPECIFIED., .F., .T. ) 
 B_SPLINE_CURVE_WITH_KNOTS ( ( 3, 2, 2, 2, 3 ),
 ( 0.2291666666666665741, 0.2395833333333332316, 0.2499999999999998335, 0.2604166666666665186, 0.2708333333333330928 ),
 .UNSPECIFIED. ) 
 CURVE ( )  GEOMETRIC_REPRESENTATION_ITEM ( )  RATIONAL_B_SPLINE_CURVE ( ( 1.000000000000000666, 0.9238795325112861834, 1.000000000000000000, 0.9238795325112867385, 1.000000000000000000, 0.9238795325112867385, 1.000000000000000000, 0.9238795325112884038, 0.9999999999999983347 ) ) 
 REPRESENTATION_ITEM ( '' )  );
#4314=CARTESIAN_POINT ( 'NONE',  ( 120.4011555911795455, 37.22968750216787726, 9.598844408820459861 ) ) ;
#4316=CARTESIAN_POINT ( 'NONE',  ( 204.2950502721270425, 39.46210937608393010, -9.295050272127046043 ) ) ;
#4317=ORIENTED_EDGE ( 'NONE', *, *, #5970, .F. ) ;
#4318=CARTESIAN_POINT ( 'NONE',  ( 135.6228728715777834, 39.95820312499999716, -13.57481594606312036 ) ) ;
#4319=ORIENTED_EDGE ( 'NONE', *, *, #24397, .F. ) ;
#4324=CARTESIAN_POINT ( 'NONE',  ( 130.0000000000000000, 31.77265625216787370, 13.57481594606304576 ) ) ;
#4326=CARTESIAN_POINT ( 'NONE',  ( 103.5355339059327093, 81.75000000273119838, -3.535533905932755072 ) ) ;
#4328=CARTESIAN_POINT ( 'NONE',  ( 181.8548138422181921, 35.93984375108393436, -5.444914386472297529 ) ) ;
#4331=ORIENTED_EDGE ( 'NONE', *, *, #3900, .F. ) ;
#4336=CARTESIAN_POINT ( 'NONE',  ( 51.42518405393695957, 36.28710937716787299, -5.622872871577872189 ) ) ;
#4337=CARTESIAN_POINT ( 'NONE',  ( 185.7049497278729575, 38.27148437608393294, 9.295050272127047819 ) ) ;
#4342=CARTESIAN_POINT ( 'NONE',  ( 65.00000000000000000, 36.03906250000000000, -13.57481594606304576 ) ) ;
#4347=AXIS2_PLACEMENT_3D ( 'NONE', #10855, #13559, #17565 ) ;
#4348=AXIS2_PLACEMENT_3D ( 'NONE', #22690, #5587, #9977 ) ;
#4350=CARTESIAN_POINT ( 'NONE',  ( 143.1451861577818079, 34.84843750108393579, -5.444914386472297529 ) ) ;
#4351=CARTESIAN_POINT ( 'NONE',  ( 55.70494972787295751, 32.71523437608393436, 9.295050272127047819 ) ) ;
#4352=CARTESIAN_POINT ( 'NONE',  ( 181.8548138422181921, 36.83281250108393579, 5.444914386472304635 ) ) ;
#4354=CARTESIAN_POINT ( 'NONE',  ( 134.0625835405769237, 50.00000000116060761, -12.98908657125173960 ) ) ;
#4359=CARTESIAN_POINT ( 'NONE',  ( -13.14518615778179900, 35.74140625108393721, -5.444914386472297529 ) ) ;
#4360=DIRECTION ( 'NONE',  ( -0.000000000000000000, 1.000000000000000000, -0.000000000000000000 ) ) ;
#4362=CARTESIAN_POINT ( 'NONE',  ( 219.9999999999999716, 55.00000000000000000, -10.00000000000000000 ) ) ;
#4364=ORIENTED_EDGE ( 'NONE', *, *, #6983, .T. ) ;
#4366=AXIS2_PLACEMENT_3D ( 'NONE', #5476, #20864, #1346 ) ;
#4370=CARTESIAN_POINT ( 'NONE',  ( 121.2273907538632898, 50.37415326813481897, 15.00000000000582645 ) ) ;
#4373=CARTESIAN_POINT ( 'NONE',  ( 101.8468681455906903, 80.00000000136559208, 4.458734124999987891 ) ) ;
#4374=CARTESIAN_POINT ( 'NONE',  ( 51.85481384221819923, 34.35234375108393579, -5.444914386472297529 ) ) ;
#4376=CYLINDRICAL_SURFACE ( 'NONE', #23682, 13.57481594606304398 ) ;
#4379=DIRECTION ( 'NONE',  ( 0.000000000000000000, 0.000000000000000000, 1.000000000000000000 ) ) ;
#4381=CARTESIAN_POINT ( 'NONE',  ( 116.4251840539369454, 36.18789062499999432, -5.622872871577873077 ) ) ;
#4382=ORIENTED_EDGE ( 'NONE', *, *, #8158, .T. ) ;
#4386=CARTESIAN_POINT ( 'NONE',  ( 120.7049497278729575, 37.27929687608393294, -9.295050272127046043 ) ) ;
#4387=CARTESIAN_POINT ( 'NONE',  ( 70.62287287157786864, 34.50117187716788436, -13.57481594606304753 ) ) ;
#4389=DIRECTION ( 'NONE',  ( 0.000000000000000000, 0.000000000000000000, -1.000000000000000000 ) ) ;
#4390=CARTESIAN_POINT ( 'NONE',  ( 5.622872871577878406, 31.82226562716787654, 13.57481594606304576 ) ) ;
#4394=CARTESIAN_POINT ( 'NONE',  ( 195.0000000000000000, 34.40195312608393152, 13.14518615778179544 ) ) ;
#4396=LINE ( 'NONE', #23917, #22880 ) ;
#4397=CARTESIAN_POINT ( 'NONE',  ( 139.2950502721270425, 36.08867187608392868, 9.295050272127046043 ) ) ;
#4399=LINE ( 'NONE', #27924, #13581 ) ;
#4400=CARTESIAN_POINT ( 'NONE',  ( 208.5748159460630688, 36.58476562499999574, 5.622872871577868636 ) ) ;
#4402=CARTESIAN_POINT ( 'NONE',  ( 0.000000000000000000, -7.395377635281828788, 0.000000000000000000 ) ) ;
#4406=CARTESIAN_POINT ( 'NONE',  ( 204.5988444088204403, 35.14609374999999858, -9.598844408820458085 ) ) ;
#4409=CARTESIAN_POINT ( 'NONE',  ( 65.00000000000000000, 35.98945312608393010, 13.14518615778179544 ) ) ;
#4415=CARTESIAN_POINT ( 'NONE',  ( 9.598844408820456309, 36.73359374999999716, -9.598844408820458085 ) ) ;
#4416=CARTESIAN_POINT ( 'NONE',  ( 139.2950502721270425, 40.45429687608393721, -9.295050272127046043 ) ) ;
#4420=CARTESIAN_POINT ( 'NONE',  ( 96.84719886470459471, 80.81250000136559208, 3.152801135295355994 ) ) ;
#4422=CARTESIAN_POINT ( 'NONE',  ( 62.91300135136894056, 36.00000000000000000, -13.31420566034952380 ) ) ;
#4423=ORIENTED_EDGE ( 'NONE', *, *, #15615, .F. ) ;
#4425=CARTESIAN_POINT ( 'NONE',  ( 78.14518615778179367, 36.33671875108394289, 5.444914386472293977 ) ) ;
#4427=EDGE_CURVE ( 'NONE', #21367, #4613, #25948, .T. ) ;
#4430=EDGE_CURVE ( 'NONE', #28041, #4816, #656, .T. ) ;
#4434=CARTESIAN_POINT ( 'NONE',  ( 185.4011555911795597, 38.81718750216787583, 9.598844408820459861 ) ) ;
#4437=CARTESIAN_POINT ( 'NONE',  ( 116.8548138422182205, 37.62656250108393152, 5.444914386472304635 ) ) ;
#4438=CARTESIAN_POINT ( 'NONE',  ( 9.295050272127046043, 38.07304687608393579, -9.295050272127046043 ) ) ;
#4439=CARTESIAN_POINT ( 'NONE',  ( 143.1451861577818079, 34.60039062608392868, -1.609821015232357215E-15 ) ) ;
#4440=CARTESIAN_POINT ( 'NONE',  ( 78.57481594606304043, 35.89023437499999858, -5.622872871577873077 ) ) ;
#4441=CARTESIAN_POINT ( 'NONE',  ( 55.40115559117954547, 39.41250000216787441, -9.598844408820458085 ) ) ;
#4442=EDGE_CURVE ( 'NONE', #27424, #3039, #17958, .T. ) ;
#4448=CARTESIAN_POINT ( 'NONE',  ( 99.99999999999995737, 80.43750000136559208, -4.458734125000016313 ) ) ;
#4450=CARTESIAN_POINT ( 'NONE',  ( 5.444914386472297529, 36.53515625108393294, -13.14518615778179900 ) ) ;
#4454=CARTESIAN_POINT ( 'NONE',  ( 195.0000000000000000, -7.395377635281828788, -2.255140518769849538E-14 ) ) ;
#4456=EDGE_CURVE ( 'NONE', #11568, #4141, #26911, .T. ) ;
#4457=CARTESIAN_POINT ( 'NONE',  ( 204.2950502721270425, 40.25585937608393294, -9.295050272127046043 ) ) ;
#4458=VERTEX_POINT ( 'NONE', #24621 ) ;
#4459=CARTESIAN_POINT ( 'NONE',  ( 139.5988444088204403, 36.03906250216787299, -9.598844408820458085 ) ) ;
#4460=FACE_OUTER_BOUND ( 'NONE', #25903, .T. ) ;
#4466=EDGE_CURVE ( 'NONE', #506, #4887, #11580, .T. ) ;
#4467=CARTESIAN_POINT ( 'NONE',  ( 124.5550856135277087, 39.90859375108393436, 13.14518615778179722 ) ) ;
#4468=DIRECTION ( 'NONE',  ( 0.000000000000000000, 0.000000000000000000, -1.000000000000000000 ) ) ;
#4470=CARTESIAN_POINT ( 'NONE',  ( 51.85481384221819923, 39.11484375108394573, -5.444914386472297529 ) ) ;
#4472=CARTESIAN_POINT ( 'NONE',  ( 200.4449143864723055, 34.94765625108394147, -13.14518615778179900 ) ) ;
#4474=ORIENTED_EDGE ( 'NONE', *, *, #10559, .T. ) ;
#4480=CARTESIAN_POINT ( 'NONE',  ( 99.99999999999995737, 82.18750000136559208, -4.458734125000016313 ) ) ;
#4481=CARTESIAN_POINT ( 'NONE',  ( 181.8548138422182205, 39.01562500108393294, 5.444914386472304635 ) ) ;
#4483=CARTESIAN_POINT ( 'NONE',  ( 189.6345034319466549, 54.48174559707876341, 14.99999999999995026 ) ) ;
#4487=AXIS2_PLACEMENT_3D ( 'NONE', #271, #8957, #15501 ) ;
#4492=CARTESIAN_POINT ( 'NONE',  ( 135.4449143864723055, 36.23750000108393721, 13.14518615778179189 ) ) ;
#4493=CARTESIAN_POINT ( 'NONE',  ( 70.44491438647230552, 34.45156250108393436, 13.14518615778179189 ) ) ;
#4494=CARTESIAN_POINT ( 'NONE',  ( 185.7049497278729575, 38.46992187608393721, 9.295050272127047819 ) ) ;
#4497=CARTESIAN_POINT ( 'NONE',  ( -13.14518615778179900, 32.56640625108394005, -5.444914386472297529 ) ) ;
#4498=CARTESIAN_POINT ( 'NONE',  ( 135.3654965680425732, 54.48174559707607756, -15.00000000000000178 ) ) ;
#4499=ADVANCED_FACE ( 'NONE', ( #11623 ), #16049, .T. ) ;
#4500=DIRECTION ( 'NONE',  ( -1.156482317317871478E-16, 0.000000000000000000, -1.000000000000000000 ) ) ;
#4501=CARTESIAN_POINT ( 'NONE',  ( 143.5748159460630404, 39.85898437716787157, 5.622872871577869525 ) ) ;
#4503=CARTESIAN_POINT ( 'NONE',  ( -6.116560239716795522, 54.66944451632673463, 14.99999999999999822 ) ) ;
#4505=CARTESIAN_POINT ( 'NONE',  ( 56.78868598481955843, 50.68678854790645971, 14.99999999999929479 ) ) ;
#4508=VERTEX_POINT ( 'NONE', #5663 ) ;
#4511=CARTESIAN_POINT ( 'NONE',  ( 120.8198241863519939, 50.00000000000000000, 9.999999999999968026 ) ) ;
#4515=CARTESIAN_POINT ( 'NONE',  ( 59.55508561352770158, 36.13828125108393863, 13.14518615778179722 ) ) ;
#4517=CARTESIAN_POINT ( 'NONE',  ( 5.444914386472302859, 37.62656250108393152, 13.14518615778179189 ) ) ;
#4518=CARTESIAN_POINT ( 'NONE',  ( 116.4251840539369596, 36.18789062499999432, -5.622872871577872189 ) ) ;
#4520=CARTESIAN_POINT ( 'NONE',  ( 143.5748159460630404, 36.68398437499999432, -5.622872871577873077 ) ) ;
#4525=CARTESIAN_POINT ( 'NONE',  ( 143.1451861577818079, 36.98164062608393010, -1.609821015232357215E-15 ) ) ;
#4526=CARTESIAN_POINT ( 'NONE',  ( 65.00000000000000000, 32.56640625216787299, 13.57481594606304576 ) ) ;
#4529=CARTESIAN_POINT ( 'NONE',  ( 13.57481594606304753, 33.60820312716787583, -5.622872871577873077 ) ) ;
#4532=CARTESIAN_POINT ( 'NONE',  ( 181.8548138422181921, 35.04687500108393294, 5.444914386472304635 ) ) ;
#4536=CARTESIAN_POINT ( 'NONE',  ( 200.6228728715779539, 39.16445312500000142, -13.57481594606299247 ) ) ;
#4537=ORIENTED_EDGE ( 'NONE', *, *, #6691, .F. ) ;
#4544=CARTESIAN_POINT ( 'NONE',  ( 189.3771271284221314, 33.70742187500000142, -13.57481594606304753 ) ) ;
#4546=LINE ( 'NONE', #8676, #12390 ) ;
#4547=CARTESIAN_POINT ( 'NONE',  ( 59.55508561352770158, 34.05468750108393294, -13.14518615778179900 ) ) ;
#4553=CARTESIAN_POINT ( 'NONE',  ( 5.622872871577871301, 37.57695312499998863, -13.57481594606304753 ) ) ;
#4554=CARTESIAN_POINT ( 'NONE',  ( 139.2950502721270425, 37.87460937608393863, 9.295050272127046043 ) ) ;
#4556=CARTESIAN_POINT ( 'NONE',  ( 96.46446609406721961, 83.87500000000000000, -3.535533905932755072 ) ) ;
#4557=CARTESIAN_POINT ( 'NONE',  ( 104.9999999999999716, 80.62500000273119838, -1.449011120738813565E-14 ) ) ;
#4559=CARTESIAN_POINT ( 'NONE',  ( 53.06475762330939006, 36.00000000000000000, -5.809862729998005904 ) ) ;
#4561=CARTESIAN_POINT ( 'NONE',  ( 51.85481384221819923, 34.35234375108393579, -5.444914386472297529 ) ) ;
#4562=ORIENTED_EDGE ( 'NONE', *, *, #20293, .F. ) ;
#4563=( BOUNDED_CURVE ( )  B_SPLINE_CURVE ( 2, ( #17617, #6785, #11895, #13894, #9351, #26900, #7490, #676, #18190 ),
 .UNSPECIFIED., .F., .F. ) 
 B_SPLINE_CURVE_WITH_KNOTS ( ( 3, 2, 2, 2, 3 ),
 ( 0.02083333333333358892, 0.03125000000000020123, 0.04166666666666681007, 0.05208333333333342585, 0.06250000000000004163 ),
 .UNSPECIFIED. ) 
 CURVE ( )  GEOMETRIC_REPRESENTATION_ITEM ( )  RATIONAL_B_SPLINE_CURVE ( ( 0.9999999999999981126, 0.9238795325112886259, 1.000000000000000000, 0.9238795325112867385, 1.000000000000000000, 0.9238795325112867385, 1.000000000000000000, 0.9238795325112864054, 1.000000000000000222 ) ) 
 REPRESENTATION_ITEM ( '' )  );
#4567=DIRECTION ( 'NONE',  ( 0.000000000000000000, 0.000000000000000000, -1.000000000000000000 ) ) ;
#4569=CARTESIAN_POINT ( 'NONE',  ( 208.5748159460630120, 35.89023437716787868, 5.622872871577869525 ) ) ;
#4570=ORIENTED_EDGE ( 'NONE', *, *, #11427, .F. ) ;
#4573=CARTESIAN_POINT ( 'NONE',  ( 124.5550856135277087, 36.13828125108393152, 13.14518615778179722 ) ) ;
#4575=CARTESIAN_POINT ( 'NONE',  ( -9.295050272127044266, 36.08867187608393579, 9.295050272127047819 ) ) ;
#4577=CARTESIAN_POINT ( 'NONE',  ( 135.4449143864723055, 36.33671875108394289, -13.14518615778179900 ) ) ;
#4578=CARTESIAN_POINT ( 'NONE',  ( 74.59884440882045453, 35.14609374999999858, -9.598844408820458085 ) ) ;
#4581=CARTESIAN_POINT ( 'NONE',  ( 181.4251840539369596, 37.03124999999999289, 0.000000000000000000 ) ) ;
#4584=DIRECTION ( 'NONE',  ( 0.000000000000000000, 0.000000000000000000, 1.000000000000000000 ) ) ;
#4587=CARTESIAN_POINT ( 'NONE',  ( 9.295050272127046043, 37.27929687608394005, -9.295050272127046043 ) ) ;
#4589=ORIENTED_EDGE ( 'NONE', *, *, #23600, .F. ) ;
#4592=CARTESIAN_POINT ( 'NONE',  ( 116.4251840539369596, 37.13046875216787868, 0.000000000000000000 ) ) ;
#4593=CARTESIAN_POINT ( 'NONE',  ( 208.1451861577817795, 39.41250000108393436, -5.444914386472297529 ) ) ;
#4596=CARTESIAN_POINT ( 'NONE',  ( 204.1801758136480203, 50.00000000000000000, -9.999999999999992895 ) ) ;
#4600=VECTOR ( 'NONE', #25704, 1000.000000000000000 ) ;
#4603=CARTESIAN_POINT ( 'NONE',  ( 139.5988444088204403, 32.86406250216787583, -9.598844408820458085 ) ) ;
#4604=CARTESIAN_POINT ( 'NONE',  ( -5.444914386472297529, 40.60312500108393863, -13.14518615778179722 ) ) ;
#4606=( BOUNDED_CURVE ( )  B_SPLINE_CURVE ( 2, ( #19158, #5781, #14307, #8185, #3499, #5921, #27314, #10452, #23165 ),
 .UNSPECIFIED., .F., .F. ) 
 B_SPLINE_CURVE_WITH_KNOTS ( ( 3, 2, 2, 2, 3 ),
 ( 0.1041666666666664909, 0.1145833333333332732, 0.1250000000000000833, 0.1354166666666668517, 0.1458333333333336757 ),
 .UNSPECIFIED. ) 
 CURVE ( )  GEOMETRIC_REPRESENTATION_ITEM ( )  RATIONAL_B_SPLINE_CURVE ( ( 1.000000000000001332, 0.9238795325112854062, 1.000000000000000000, 0.9238795325112867385, 1.000000000000000000, 0.9238795325112867385, 1.000000000000000000, 0.9238795325112842960, 1.000000000000002442 ) ) 
 REPRESENTATION_ITEM ( '' )  );
#4609=CARTESIAN_POINT ( 'NONE',  ( 55.70494972787295751, 36.88242187608393152, 9.295050272127047819 ) ) ;
#4610=CARTESIAN_POINT ( 'NONE',  ( 74.18017581364799184, 50.00000000000000000, -15.00000000000000000 ) ) ;
#4611=CARTESIAN_POINT ( 'NONE',  ( 181.8548138422182205, 33.60820312608393579, 0.000000000000000000 ) ) ;
#4613=VERTEX_POINT ( 'NONE', #5936 ) ;
#4617=EDGE_CURVE ( 'NONE', #5488, #4145, #15221, .T. ) ;
#4618=CARTESIAN_POINT ( 'NONE',  ( 70.44491438647229131, 40.30546875108393579, -13.14518615778179722 ) ) ;
#4619=CARTESIAN_POINT ( 'NONE',  ( 103.1528011352953342, 79.81250000136559208, 3.152801135295355106 ) ) ;
#4620=CARTESIAN_POINT ( 'NONE',  ( 208.1451861577818079, 37.77539062608393294, -1.609821015232357215E-15 ) ) ;
#4621=ADVANCED_FACE ( 'NONE', ( #20767, #8200 ), #6073, .F. ) ;
#4631=EDGE_LOOP ( 'NONE', ( #23437, #20704, #27778, #22177 ) ) ;
#4632=CARTESIAN_POINT ( 'NONE',  ( 135.4449143864723055, 37.32890625108393579, -13.14518615778179900 ) ) ;
#4633=CARTESIAN_POINT ( 'NONE',  ( 74.29505027212704249, 35.29492187608393294, 9.295050272127046043 ) ) ;
#4634=EDGE_CURVE ( 'NONE', #5134, #9259, #1528, .T. ) ;
#4635=CARTESIAN_POINT ( 'NONE',  ( 204.2950502721270425, 36.48554687608393721, -9.295050272127046043 ) ) ;
#4636=VERTEX_POINT ( 'NONE', #16891 ) ;
#4638=CARTESIAN_POINT ( 'NONE',  ( -13.14518615778179544, 33.40976562608393863, 0.000000000000000000 ) ) ;
#4639=CARTESIAN_POINT ( 'NONE',  ( 128.1078166429076646, 53.66387243068088964, -14.99999999999999822 ) ) ;
#4641=CARTESIAN_POINT ( 'NONE',  ( 4.157286354961724939, 36.00000000000000000, -12.92256159328856135 ) ) ;
#4643=( BOUNDED_CURVE ( )  B_SPLINE_CURVE ( 2, ( #25666, #1884, #19390, #23813, #10408 ),
 .UNSPECIFIED., .F., .F. ) 
 B_SPLINE_CURVE_WITH_KNOTS ( ( 3, 2, 3 ),
 ( 0.4375000000000003331, 0.4479166666666667962, 0.4520580917964582834 ),
 .UNSPECIFIED. ) 
 CURVE ( )  GEOMETRIC_REPRESENTATION_ITEM ( )  RATIONAL_B_SPLINE_CURVE ( ( 0.9999999999999975575, 0.9238795325112891810, 1.000000000000000000, 0.9697362671728727568, 0.9635368512068458458 ) ) 
 REPRESENTATION_ITEM ( '' )  );
#4644=CARTESIAN_POINT ( 'NONE',  ( 195.0000000000000000, 36.03906250000000000, -13.57481594606304576 ) ) ;
#4648=( NAMED_UNIT ( * ) SI_UNIT ( $, .STERADIAN. ) SOLID_ANGLE_UNIT ( ) );
#4655=CARTESIAN_POINT ( 'NONE',  ( 116.4251840539369596, 38.66835937716787441, -5.622872871577872189 ) ) ;
#4656=FACE_OUTER_BOUND ( 'NONE', #27530, .T. ) ;
#4657=CARTESIAN_POINT ( 'NONE',  ( 65.00000000000000000, 35.79101562608394005, -13.14518615778179544 ) ) ;
#4659=CARTESIAN_POINT ( 'NONE',  ( -9.295050272127044266, 36.68398437608392726, 9.295050272127047819 ) ) ;
#4661=DIRECTION ( 'NONE',  ( -0.000000000000000000, 1.000000000000000000, -0.000000000000000000 ) ) ;
#4663=CARTESIAN_POINT ( 'NONE',  ( 143.5748159460630404, 38.17226562499999432, 5.622872871577869525 ) ) ;
#4664=ORIENTED_EDGE ( 'NONE', *, *, #1327, .T. ) ;
#4667=CARTESIAN_POINT ( 'NONE',  ( 219.9999999999999716, 50.00000000000000000, -10.00000000000000000 ) ) ;
#4671=CARTESIAN_POINT ( 'NONE',  ( 116.8548138422182205, 38.17226562608393436, 0.000000000000000000 ) ) ;
#4672=CARTESIAN_POINT ( 'NONE',  ( 70.62287287157786864, 35.29492187716788720, -13.57481594606304753 ) ) ;
#4675=CARTESIAN_POINT ( 'NONE',  ( -9.598844408820454532, 34.05468750216788010, 9.598844408820459861 ) ) ;
#4678=CARTESIAN_POINT ( 'NONE',  ( 208.1451861577817795, 33.85625000108393579, -5.444914386472297529 ) ) ;
#4679=CYLINDRICAL_SURFACE ( 'NONE', #11062, 13.57481594606304398 ) ;
#4680=VECTOR ( 'NONE', #7226, 1000.000000000000000 ) ;
#4681=CARTESIAN_POINT ( 'NONE',  ( 143.1451861577818363, 36.23750000108393010, -5.444914386472297529 ) ) ;
#4682=CARTESIAN_POINT ( 'NONE',  ( 181.4251840539369596, 40.20624999999999005, 0.000000000000000000 ) ) ;
#4684=CARTESIAN_POINT ( 'NONE',  ( 214.9999999999999716, 75.00000000000000000, 9.999999999999946709 ) ) ;
#4685=CARTESIAN_POINT ( 'NONE',  ( 208.5748159460630688, 39.16445312716788152, -5.622872871577873966 ) ) ;
#4690=CARTESIAN_POINT ( 'NONE',  ( 208.5748159460630120, 34.20351562499999432, 5.622872871577869525 ) ) ;
#4692=CARTESIAN_POINT ( 'NONE',  ( 51.42518405393695957, 40.25585937499999289, 5.622872871577880183 ) ) ;
#4693=CARTESIAN_POINT ( 'NONE',  ( 78.14518615778179367, 35.44375000108393436, -5.444914386472297529 ) ) ;
#4697=DIRECTION ( 'NONE',  ( 0.000000000000000000, 0.000000000000000000, -1.000000000000000000 ) ) ;
#4698=CARTESIAN_POINT ( 'NONE',  ( -9.598844408820458085, 36.13828124999999147, -9.598844408820458085 ) ) ;
#4699=CARTESIAN_POINT ( 'NONE',  ( 116.8548138422182063, 38.32109375108394289, -5.444914386472297529 ) ) ;
#4701=CARTESIAN_POINT ( 'NONE',  ( 101.8468681455906903, 81.00000000136560629, 4.458734124999987891 ) ) ;
#4703=CARTESIAN_POINT ( 'NONE',  ( 94.99999999999995737, 82.18750000273121259, 2.071067811865466624 ) ) ;
#4705=CARTESIAN_POINT ( 'NONE',  ( 69.15728635496172672, 36.00000000000000000, -12.92256159328856135 ) ) ;
#4708=CARTESIAN_POINT ( 'NONE',  ( 78.57481594606305464, 39.80937499999999574, -1.662435489736055892E-15 ) ) ;
#4709=VERTEX_POINT ( 'NONE', #16621 ) ;
#4712=ORIENTED_EDGE ( 'NONE', *, *, #3607, .F. ) ;
#4716=CARTESIAN_POINT ( 'NONE',  ( 208.5748159460630120, 33.50898437716787015, 5.622872871577869525 ) ) ;
#4717=ORIENTED_EDGE ( 'NONE', *, *, #9121, .F. ) ;
#4719=DIRECTION ( 'NONE',  ( -1.000000000000000000, -0.000000000000000000, -0.000000000000000000 ) ) ;
#4720=CARTESIAN_POINT ( 'NONE',  ( 139.2950502721270425, 36.48554687608393721, -9.295050272127046043 ) ) ;
#4721=CARTESIAN_POINT ( 'NONE',  ( -5.444914386472297529, 34.25312500108393010, -13.14518615778179900 ) ) ;
#4722=CARTESIAN_POINT ( 'NONE',  ( 139.2950502721270425, 33.90585937608393152, -9.295050272127046043 ) ) ;
#4723=CARTESIAN_POINT ( 'NONE',  ( 65.00000000000000000, 36.03906250000000000, -13.57481594606304576 ) ) ;
#4726=VECTOR ( 'NONE', #8630, 1000.000000000000000 ) ;
#4727=FACE_OUTER_BOUND ( 'NONE', #13614, .T. ) ;
#4730=CARTESIAN_POINT ( 'NONE',  ( 99.99999999999995737, 80.00000000000000000, -1.387778780781445676E-14 ) ) ;
#4731=CARTESIAN_POINT ( 'NONE',  ( 99.99999999999995737, 83.87500000273119838, -5.000000000000018652 ) ) ;
#4733=CARTESIAN_POINT ( 'NONE',  ( 13.14518615778179900, 35.64218750108393152, -5.444914386472297529 ) ) ;
#4740=CARTESIAN_POINT ( 'NONE',  ( 204.2950502721270425, 35.49335937608393010, -9.295050272127046043 ) ) ;
#4741=VERTEX_POINT ( 'NONE', #12324 ) ;
#4743=CARTESIAN_POINT ( 'NONE',  ( 135.6228728715777549, 39.66054687500000142, 13.57481594606318076 ) ) ;
#4744=EDGE_CURVE ( 'NONE', #18339, #13739, #10180, .T. ) ;
#4749=CARTESIAN_POINT ( 'NONE',  ( 130.0000000000000000, 32.16953125216787157, -13.57481594606304576 ) ) ;
#4753=CARTESIAN_POINT ( 'NONE',  ( 55.70494972787295751, 37.47773437608393010, -9.295050272127046043 ) ) ;
#4754=CARTESIAN_POINT ( 'NONE',  ( 58.12649175642295063, 51.14166184781131363, -15.00000000000130917 ) ) ;
#4755=CARTESIAN_POINT ( 'NONE',  ( 200.6228728715778686, 39.66054687500000142, 13.57481594606304576 ) ) ;
#4756=DIRECTION ( 'NONE',  ( -0.000000000000000000, 1.000000000000000000, 0.000000000000000000 ) ) ;
#4757=ORIENTED_EDGE ( 'NONE', *, *, #3586, .F. ) ;
#4758=ORIENTED_EDGE ( 'NONE', *, *, #25461, .T. ) ;
#4761=CARTESIAN_POINT ( 'NONE',  ( 55.70494972787295751, 36.68398437608392726, 9.295050272127047819 ) ) ;
#4763=CARTESIAN_POINT ( 'NONE',  ( 189.5550856135277229, 39.11484375108393863, 13.14518615778179722 ) ) ;
#4766=CARTESIAN_POINT ( 'NONE',  ( 208.1451861577818079, 38.76757812608393294, -1.609821015232357215E-15 ) ) ;
#4769=EDGE_CURVE ( 'NONE', #15330, #13131, #27478, .T. ) ;
#4773=ORIENTED_EDGE ( 'NONE', *, *, #368, .T. ) ;
#4774=CARTESIAN_POINT ( 'NONE',  ( 124.5550856135277087, 34.55078125108393294, 13.14518615778179722 ) ) ;
#4775=CARTESIAN_POINT ( 'NONE',  ( 65.00000000000000000, 34.00507812608393721, -13.14518615778179544 ) ) ;
#4776=CARTESIAN_POINT ( 'NONE',  ( 208.1451861577817795, 37.92421875108392726, 5.444914386472293977 ) ) ;
#4780=CARTESIAN_POINT ( 'NONE',  ( 13.14518615778179544, 33.80664062608393294, -1.609821015232357215E-15 ) ) ;
#4783=CARTESIAN_POINT ( 'NONE',  ( 195.0000000000000000, 36.13828125216787157, -13.57481594606304576 ) ) ;
#4785=EDGE_CURVE ( 'NONE', #13739, #24582, #9050, .T. ) ;
#4788=CARTESIAN_POINT ( 'NONE',  ( 195.0000000000000000, 39.75976562608394005, -13.14518615778179544 ) ) ;
#4792=ORIENTED_EDGE ( 'NONE', *, *, #10643, .T. ) ;
#4795=CARTESIAN_POINT ( 'NONE',  ( 128.0526740779191073, 51.47162402671428794, 14.99999999999996803 ) ) ;
#4799=CARTESIAN_POINT ( 'NONE',  ( 101.8468681455906903, 83.00000000136559208, 4.458734124999987891 ) ) ;
#4800=CARTESIAN_POINT ( 'NONE',  ( 51.85481384221820633, 36.03906250108394005, 5.444914386472304635 ) ) ;
#4801=CARTESIAN_POINT ( 'NONE',  ( 185.4011555911795597, 37.92421874999999432, 9.598844408820459861 ) ) ;
#4802=CARTESIAN_POINT ( 'NONE',  ( 5.444914386472302859, 39.21406250108392300, 13.14518615778179189 ) ) ;
#4804=CARTESIAN_POINT ( 'NONE',  ( 103.5355339059327093, 80.50000000273119838, 3.535533905932726206 ) ) ;
#4807=CARTESIAN_POINT ( 'NONE',  ( 143.5748159460630688, 38.22187499999999716, -1.662435489736055892E-15 ) ) ;
#4808=ORIENTED_EDGE ( 'NONE', *, *, #4442, .T. ) ;
#4813=CARTESIAN_POINT ( 'NONE',  ( 139.2950502721270425, 32.31835937608393294, -9.295050272127046043 ) ) ;
#4814=CARTESIAN_POINT ( 'NONE',  ( 74.59884440882045453, 32.86406250216787583, -9.598844408820458085 ) ) ;
#4816=VERTEX_POINT ( 'NONE', #6762 ) ;
#4817=AXIS2_PLACEMENT_3D ( 'NONE', #25573, #21160, #14722 ) ;
#4819=CARTESIAN_POINT ( 'NONE',  ( 5.622872871577871301, 32.11992187716787583, -13.57481594606304753 ) ) ;
#4820=( BOUNDED_CURVE ( )  B_SPLINE_CURVE ( 2, ( #1806, #10056, #1533, #18767, #1944, #1395, #27882, #23599, #3667 ),
 .UNSPECIFIED., .F., .F. ) 
 B_SPLINE_CURVE_WITH_KNOTS ( ( 3, 2, 2, 2, 3 ),
 ( 0.5500000000000004885, 0.5750000000000003997, 0.6000000000000005329, 0.6250000000000005551, 0.6500000000000005773 ),
 .UNSPECIFIED. ) 
 CURVE ( )  GEOMETRIC_REPRESENTATION_ITEM ( )  RATIONAL_B_SPLINE_CURVE ( ( 0.9999999999999986677, 0.9238795325112880708, 1.000000000000000000, 0.9238795325112867385, 1.000000000000000000, 0.9238795325112867385, 1.000000000000000000, 0.9238795325112850731, 1.000000000000001776 ) ) 
 REPRESENTATION_ITEM ( '' )  );
#4821=CARTESIAN_POINT ( 'NONE',  ( 65.00000000000000000, 38.02343749999999289, 13.57481594606304576 ) ) ;
#4824=CARTESIAN_POINT ( 'NONE',  ( 195.0000000000000000, 33.21132812608393436, -13.14518615778179544 ) ) ;
#4825=AXIS2_PLACEMENT_3D ( 'NONE', #13822, #19094, #10386 ) ;
#4826=CARTESIAN_POINT ( 'NONE',  ( 217.9999999999999716, 80.00000000000000000, 12.99999999999994316 ) ) ;
#4827=LINE ( 'NONE', #23679, #11706 ) ;
#4829=CARTESIAN_POINT ( 'NONE',  ( 99.99999999999995737, 81.25000000000000000, 4.999999999999990230 ) ) ;
#4832=CARTESIAN_POINT ( 'NONE',  ( 208.5748159460630688, 36.68398437500000142, -5.622872871577873966 ) ) ;
#4834=DIRECTION ( 'NONE',  ( -0.000000000000000000, 1.000000000000000000, -0.000000000000000000 ) ) ;
#4837=CARTESIAN_POINT ( 'NONE',  ( 204.5988444088204403, 33.55859375000000000, -9.598844408820458085 ) ) ;
#4839=DIRECTION ( 'NONE',  ( 0.000000000000000000, -1.000000000000000000, 0.000000000000000000 ) ) ;
#4841=CARTESIAN_POINT ( 'NONE',  ( 51.85481384221820633, 36.63437500108393152, 5.444914386472304635 ) ) ;
#4844=CARTESIAN_POINT ( 'NONE',  ( 9.598844408820459861, 37.32890624999999574, 9.598844408820456309 ) ) ;
#4845=CARTESIAN_POINT ( 'NONE',  ( 139.2950502721270425, 38.07304687608393579, -9.295050272127046043 ) ) ;
#4847=DIRECTION ( 'NONE',  ( 0.8660254037844407060, 0.4999999999999963363, 0.000000000000000000 ) ) ;
#4849=CARTESIAN_POINT ( 'NONE',  ( 102.0710678118654329, 81.43750000273121259, 4.999999999999989342 ) ) ;
#4851=CARTESIAN_POINT ( 'NONE',  ( 68.08926091379791501, 35.99999999999998579, -13.21136010216353540 ) ) ;
#4853=CARTESIAN_POINT ( 'NONE',  ( 74.59884440882045453, 40.50390624999999289, 9.598844408820456309 ) ) ;
#4854=EDGE_LOOP ( 'NONE', ( #25979, #27722, #23942, #15444 ) ) ;
#4860=CARTESIAN_POINT ( 'NONE',  ( 181.4251840539369596, 34.79882812716787299, 5.622872871577880183 ) ) ;
#4861=CIRCLE ( 'NONE', #10749, 5.000000000000004441 ) ;
#4865=CARTESIAN_POINT ( 'NONE',  ( 116.8548138422182205, 36.73359375108393010, -5.444914386472297529 ) ) ;
#4867=CARTESIAN_POINT ( 'NONE',  ( -9.295050272127046043, 34.30273437608393294, -9.295050272127046043 ) ) ;
#4868=CARTESIAN_POINT ( 'NONE',  ( 124.5550856135277087, 33.26093750108393721, -13.14518615778179900 ) ) ;
#4869=CARTESIAN_POINT ( 'NONE',  ( 51.42518405393695957, 36.18789062499999432, -5.622872871577873077 ) ) ;
#4873=CYLINDRICAL_SURFACE ( 'NONE', #321, 5.000000000000004441 ) ;
#4876=FACE_OUTER_BOUND ( 'NONE', #23451, .T. ) ;
#4879=CARTESIAN_POINT ( 'NONE',  ( 2.414731522848535132E-15, 37.77539062608393294, 13.14518615778179544 ) ) ;
#4886=CARTESIAN_POINT ( 'NONE',  ( 195.0000000000000000, 37.18007812608393436, -13.14518615778179544 ) ) ;
#4887=VERTEX_POINT ( 'NONE', #4077 ) ;
#4888=CARTESIAN_POINT ( 'NONE',  ( 196.6052718765765803, 53.60388944777320575, -15.00000000000000000 ) ) ;
#4894=CARTESIAN_POINT ( 'NONE',  ( 116.8548138422182063, 39.71015625108393010, -5.444914386472297529 ) ) ;
#4895=CARTESIAN_POINT ( 'NONE',  ( 1.662435489736055498E-15, -7.395377635281828788, -13.57481594606304398 ) ) ;
#4896=CARTESIAN_POINT ( 'NONE',  ( -13.14518615778179189, 35.84062500108394289, 5.444914386472304635 ) ) ;
#4898=VECTOR ( 'NONE', #27472, 1000.000000000000000 ) ;
#4899=CARTESIAN_POINT ( 'NONE',  ( 70.44491438647230552, 38.61875000108393152, 13.14518615778179189 ) ) ;
#4900=AXIS2_PLACEMENT_3D ( 'NONE', #13801, #26807, #14470 ) ;
#4901=CARTESIAN_POINT ( 'NONE',  ( 56.23061032792084291, 50.37710889401579806, -14.99999999999737632 ) ) ;
#4903=CARTESIAN_POINT ( 'NONE',  ( 185.4011555911795313, 40.90078124999999432, -9.598844408820458085 ) ) ;
#4904=CARTESIAN_POINT ( 'NONE',  ( 71.10665865494748061, 36.00000000000002132, 11.74215035806574825 ) ) ;
#4908=CARTESIAN_POINT ( 'NONE',  ( 70.44491438647229131, 37.92421875108393436, -13.14518615778179722 ) ) ;
#4909=CARTESIAN_POINT ( 'NONE',  ( 59.37712712842203189, 38.46992187499999005, -13.57481594606295339 ) ) ;
#4915=CARTESIAN_POINT ( 'NONE',  ( 189.5550856135277229, 36.93203125108394147, 13.14518615778179722 ) ) ;
#4917=ORIENTED_EDGE ( 'NONE', *, *, #16163, .T. ) ;
#4920=ORIENTED_EDGE ( 'NONE', *, *, #608, .F. ) ;
#4921=CARTESIAN_POINT ( 'NONE',  ( 135.4449143864723055, 34.65000000108393863, 13.14518615778179189 ) ) ;
#4922=CARTESIAN_POINT ( 'NONE',  ( 74.29505027212704249, 40.45429687608393721, -9.295050272127046043 ) ) ;
#4923=CARTESIAN_POINT ( 'NONE',  ( 185.7049497278729575, 35.29492187608393294, 9.295050272127047819 ) ) ;
#4926=CARTESIAN_POINT ( 'NONE',  ( -5.444914386472297529, 32.46718750108393436, -13.14518615778179900 ) ) ;
#4933=VERTEX_POINT ( 'NONE', #26150 ) ;
#4939=CARTESIAN_POINT ( 'NONE',  ( 200.6228728715777834, 38.07304687499999574, 13.57481594606313813 ) ) ;
#4941=CARTESIAN_POINT ( 'NONE',  ( -12.99948823019060384, 36.00000000000000000, 1.999176114741853194 ) ) ;
#4942=CARTESIAN_POINT ( 'NONE',  ( 55.70494972787295751, 31.92148437608393508, -9.295050272127046043 ) ) ;
#4944=CARTESIAN_POINT ( 'NONE',  ( 2.414731522848535132E-15, 36.78320312608393294, 13.14518615778179544 ) ) ;
#4947=CARTESIAN_POINT ( 'NONE',  ( 7.621963534195377754, 54.91641323977498956, 14.99999999999999289 ) ) ;
#4949=CARTESIAN_POINT ( 'NONE',  ( 124.3771271284221314, 36.38632812499999858, 13.57481594606304753 ) ) ;
#4953=EDGE_CURVE ( 'NONE', #12988, #18339, #9315, .T. ) ;
#4958=CARTESIAN_POINT ( 'NONE',  ( 135.4449143864723055, 33.65781250108393152, 13.14518615778179189 ) ) ;
#4959=CARTESIAN_POINT ( 'NONE',  ( 78.57481594606304043, 32.81445312716787299, -5.622872871577873077 ) ) ;
#4960=VERTEX_POINT ( 'NONE', #6342 ) ;
#4961=CARTESIAN_POINT ( 'NONE',  ( 13.57481594606304931, 37.47773437716787015, 5.622872871577868636 ) ) ;
#4962=CARTESIAN_POINT ( 'NONE',  ( -13.57481594606304576, 32.41757812716787157, 5.622872871577880183 ) ) ;
#4963=VECTOR ( 'NONE', #27904, 1000.000000000000000 ) ;
#4964=CARTESIAN_POINT ( 'NONE',  ( 55.40115559117954547, 37.92421874999999432, 9.598844408820459861 ) ) ;
#4968=CARTESIAN_POINT ( 'NONE',  ( 200.4449143864723055, 35.24531250108393010, 13.14518615778179189 ) ) ;
#4969=LINE ( 'NONE', #18209, #2002 ) ;
#4972=CARTESIAN_POINT ( 'NONE',  ( 116.4251840539369596, 36.28710937716787299, -5.622872871577872189 ) ) ;
#4980=CARTESIAN_POINT ( 'NONE',  ( 101.8468681455906903, 83.75000000136560629, 4.458734124999987891 ) ) ;
#4981=CARTESIAN_POINT ( 'NONE',  ( 74.29505027212704249, 34.50117187608393010, 9.295050272127046043 ) ) ;
#4986=CARTESIAN_POINT ( 'NONE',  ( 5.622872871577870413, 37.57695312499999574, -13.57481594606304753 ) ) ;
#4987=CARTESIAN_POINT ( 'NONE',  ( 2.493653234604083739E-15, 33.26093749999999716, 13.57481594606304576 ) ) ;
#4988=CARTESIAN_POINT ( 'NONE',  ( 135.4449143864723055, 37.32890625108393579, -13.14518615778179900 ) ) ;
#4990=CARTESIAN_POINT ( 'NONE',  ( 99.99999999999995737, 80.25000000000000000, 4.999999999999990230 ) ) ;
#4993=CARTESIAN_POINT ( 'NONE',  ( 96.46446609406721961, 81.00000000273119838, -3.535533905932755072 ) ) ;
#4999=CARTESIAN_POINT ( 'NONE',  ( 59.55508561352770158, 32.66562500108393863, -13.14518615778179900 ) ) ;
#5004=ORIENTED_EDGE ( 'NONE', *, *, #3446, .T. ) ;
#5006=CARTESIAN_POINT ( 'NONE',  ( 189.3771271284221314, 35.39414062716787157, -13.57481594606304753 ) ) ;
#5009=CARTESIAN_POINT ( 'NONE',  ( 5.444914386472302859, 33.85625000108393579, 13.14518615778179189 ) ) ;
#5010=CARTESIAN_POINT ( 'NONE',  ( 135.4449143864723055, 32.86406250108392868, 13.14518615778179189 ) ) ;
#5013=CARTESIAN_POINT ( 'NONE',  ( 74.59884440882045453, 36.63437500216787157, 9.598844408820456309 ) ) ;
#5015=CARTESIAN_POINT ( 'NONE',  ( 132.1298106584280561, 36.02027164734403897, -13.57481594606306174 ) ) ;
#5019=CYLINDRICAL_SURFACE ( 'NONE', #260, 5.000000000000004441 ) ;
#5021=CARTESIAN_POINT ( 'NONE',  ( -9.295050272127044266, 37.67617187608393436, 9.295050272127047819 ) ) ;
#5025=CARTESIAN_POINT ( 'NONE',  ( -9.598844408820454532, 36.33671874999999574, 9.598844408820459861 ) ) ;
#5027=CARTESIAN_POINT ( 'NONE',  ( 189.5550856135277229, 36.73359375108393010, 13.14518615778179722 ) ) ;
#5029=CARTESIAN_POINT ( 'NONE',  ( 198.8654143754131951, 54.10683252460147941, -15.00000000000000178 ) ) ;
#5031=ORIENTED_EDGE ( 'NONE', *, *, #18246, .F. ) ;
#5034=CARTESIAN_POINT ( 'NONE',  ( 94.99999999999995737, 79.12500000273118417, -1.387778780781445676E-14 ) ) ;
#5035=CARTESIAN_POINT ( 'NONE',  ( 124.5550856135277087, 37.52734375108393294, 13.14518615778179722 ) ) ;
#5036=CARTESIAN_POINT ( 'NONE',  ( 2.414731522848535132E-15, 40.15664062608393436, 13.14518615778179544 ) ) ;
#5037=CARTESIAN_POINT ( 'NONE',  ( -5.444914386472297529, 34.84843750108393579, -13.14518615778179900 ) ) ;
#5038=VECTOR ( 'NONE', #5954, 1000.000000000000000 ) ;
#5040=CARTESIAN_POINT ( 'NONE',  ( 59.55508561352770158, 38.22187500108393010, -13.14518615778179900 ) ) ;
#5041=CARTESIAN_POINT ( 'NONE',  ( 66.60253313061534186, 53.60343507247940664, -15.00000000000000000 ) ) ;
#5043=CARTESIAN_POINT ( 'NONE',  ( 181.8548138422181921, 32.86406250108393579, 5.444914386472304635 ) ) ;
#5047=CARTESIAN_POINT ( 'NONE',  ( 51.85481384221820633, 38.91640625108393436, -5.444914386472297529 ) ) ;
#5051=ORIENTED_EDGE ( 'NONE', *, *, #17246, .F. ) ;
#5054=CARTESIAN_POINT ( 'NONE',  ( 181.8548138422182205, 37.52734375108393294, -5.444914386472297529 ) ) ;
#5060=ORIENTED_EDGE ( 'NONE', *, *, #14583, .F. ) ;
#5061=CARTESIAN_POINT ( 'NONE',  ( 143.1451861577818079, 33.26093750108393721, -5.444914386472297529 ) ) ;
#5062=CARTESIAN_POINT ( 'NONE',  ( 71.94442379715272295, 31.55306878032414986, -11.16113333171310451 ) ) ;
#5063=CARTESIAN_POINT ( 'NONE',  ( 189.5550856135277229, 32.66562500108393863, -13.14518615778179900 ) ) ;
#5064=ORIENTED_EDGE ( 'NONE', *, *, #15621, .T. ) ;
#5066=CARTESIAN_POINT ( 'NONE',  ( 8.402315781223892444, 54.99999999485618929, -15.00000000000000000 ) ) ;
#5067=CIRCLE ( 'NONE', #27815, 5.000000000000000888 ) ;
#5068=CARTESIAN_POINT ( 'NONE',  ( 120.4011555911795455, 38.61875000216787157, -9.598844408820458085 ) ) ;
#5074=CARTESIAN_POINT ( 'NONE',  ( 66.50549218155768472, 53.60078691996477573, 14.99999999999997868 ) ) ;
#5075=ORIENTED_EDGE ( 'NONE', *, *, #15588, .F. ) ;
#5076=PRESENTATION_STYLE_ASSIGNMENT (( #24597 ) ) ;
#5080=CARTESIAN_POINT ( 'NONE',  ( 133.9798144458084721, 50.00000000123269928, 13.01613927312840779 ) ) ;
#5083=CARTESIAN_POINT ( 'NONE',  ( 59.55508561352770158, 33.45937500108394147, -13.14518615778179900 ) ) ;
#5086=CARTESIAN_POINT ( 'NONE',  ( 13.14518615778179722, 37.82500000108392868, -5.444914386472297529 ) ) ;
#5088=CARTESIAN_POINT ( 'NONE',  ( -3.114697745540297547, 53.90847045361019951, 15.00000000000000000 ) ) ;
#5090=CARTESIAN_POINT ( 'NONE',  ( 116.4251840539369596, 35.44374999999999432, 0.000000000000000000 ) ) ;
#5092=FACE_BOUND ( 'NONE', #17419, .T. ) ;
#5096=CARTESIAN_POINT ( 'NONE',  ( 124.5550856135277087, 33.26093750108393721, -13.14518615778179900 ) ) ;
#5097=CARTESIAN_POINT ( 'NONE',  ( 51.42518405393695957, 31.57421875216786944, 0.000000000000000000 ) ) ;
#5098=CARTESIAN_POINT ( 'NONE',  ( 51.42518405393695957, 37.08085937716787583, -5.622872871577872189 ) ) ;
#5099=CARTESIAN_POINT ( 'NONE',  ( 13.14518615778179900, 40.10703125108393152, 5.444914386472293977 ) ) ;
#5104=CARTESIAN_POINT ( 'NONE',  ( 204.2950502721270425, 32.31835937608393294, -9.295050272127046043 ) ) ;
#5105=DIRECTION ( 'NONE',  ( 0.000000000000000000, 0.000000000000000000, 1.000000000000000000 ) ) ;
#5116=DIRECTION ( 'NONE',  ( -0.000000000000000000, 1.000000000000000000, -0.000000000000000000 ) ) ;
#5117=CARTESIAN_POINT ( 'NONE',  ( 74.29505027212704249, 40.25585937608393294, 9.295050272127046043 ) ) ;
#5118=( BOUNDED_CURVE ( )  B_SPLINE_CURVE ( 2, ( #8648, #21206, #10348, #19055, #3962, #25752, #12622, #4099, #21348, #1826, #12762, #21482, #1962, #10631, #2099, #28039, #8506, #17191, #25898, #6368, #15040, #12893, #10767, #19478, #20048, #17613, #13461, #4802, #2522, #26467, #15892, #26753, #11183, #15325, #15614, #7196, #22186, #527, #17471, #20188, #24181, #22332, #6921, #15467, #17902, #24316, #13748, #2666, #13321, #24608, #26321, #24460, #672, #24038, #2388, #5086, #11327, #22473, #6782, #4517, #20330, #21913, #9346, #19756, #18039, #9208, #26611, #2802, #7057, #2936, #26173, #15756, #13609, #13174, #11607, #22046, #4944, #8925, #4659, #11046, #385, #11469, #8784, #238, #6640, #19901, #9069, #17764, #11754, #9767, #14311, #22617, #18476 ),
 .UNSPECIFIED., .F., .F. ) 
 B_SPLINE_CURVE_WITH_KNOTS ( ( 3, 2, 2, 2, 2, 2, 2, 2, 2, 2, 2, 2, 2, 2, 2, 2, 2, 2, 2, 2, 2, 2, 2, 2, 2, 2, 2, 2, 2, 2, 2, 2, 2, 2, 2, 2, 2, 2, 2, 2, 2, 2, 2, 2, 2, 2, 3 ),
 ( 0.000000000000000000, 0.01041666666666666609, 0.02083333333333333218, 0.03125000000000000000, 0.04166666666666666435, 0.05208333333333333565, 0.06250000000000000000, 0.07291666666666667129, 0.08333333333333332871, 0.09375000000000000000, 0.1041666666666666713, 0.1145833333333333287, 0.1250000000000000000, 0.1354166666666666574, 0.1458333333333333426, 0.1562500000000000000, 0.1666666666666666574, 0.1770833333333333426, 0.1875000000000000000, 0.1979166666666666574, 0.2083333333333333426, 0.2187500000000000000, 0.2291666666666666574, 0.2395833333333333426, 0.2500000000000000000, 0.2604166666666666852, 0.2708333333333333148, 0.2812500000000000000, 0.2916666666666666852, 0.3020833333333333148, 0.3125000000000000000, 0.3229166666666666852, 0.3333333333333333148, 0.3437500000000000000, 0.3541666666666666852, 0.3645833333333333148, 0.3750000000000000000, 0.3854166666666666852, 0.3958333333333333148, 0.4062500000000000000, 0.4166666666666666852, 0.4270833333333333148, 0.4375000000000000000, 0.4479166666666666852, 0.4583333333333333148, 0.4687500000000000000, 0.4779971559588572227 ),
 .UNSPECIFIED. ) 
 CURVE ( )  GEOMETRIC_REPRESENTATION_ITEM ( )  RATIONAL_B_SPLINE_CURVE ( ( 1.000000000000000000, 0.9238795325112867385, 1.000000000000000000, 0.9238795325112867385, 1.000000000000000000, 0.9238795325112867385, 1.000000000000000000, 0.9238795325112867385, 1.000000000000000000, 0.9238795325112867385, 1.000000000000000000, 0.9238795325112867385, 1.000000000000000000, 0.9238795325112867385, 1.000000000000000000, 0.9238795325112867385, 1.000000000000000000, 0.9238795325112867385, 1.000000000000000000, 0.9238795325112867385, 1.000000000000000000, 0.9238795325112867385, 1.000000000000000000, 0.9238795325112867385, 1.000000000000000000, 0.9238795325112867385, 1.000000000000000000, 0.9238795325112867385, 1.000000000000000000, 0.9238795325112867385, 1.000000000000000000, 0.9238795325112867385, 1.000000000000000000, 0.9238795325112867385, 1.000000000000000000, 0.9238795325112867385, 1.000000000000000000, 0.9238795325112867385, 1.000000000000000000, 0.9238795325112867385, 1.000000000000000000, 0.9238795325112867385, 1.000000000000000000, 0.9238795325112867385, 1.000000000000000000, 0.9238795325112867385, 1.000000000000000000, 0.9238795325112867385, 1.000000000000000000, 0.9238795325112867385, 1.000000000000000000, 0.9238795325112867385, 1.000000000000000000, 0.9238795325112867385, 1.000000000000000000, 0.9238795325112867385, 1.000000000000000000, 0.9238795325112867385, 1.000000000000000000, 0.9238795325112867385, 1.000000000000000000, 0.9238795325112867385, 1.000000000000000000, 0.9238795325112867385, 1.000000000000000000, 0.9238795325112867385, 1.000000000000000000, 0.9238795325112867385, 1.000000000000000000, 0.9238795325112867385, 1.000000000000000000, 0.9238795325112867385, 1.000000000000000000, 0.9238795325112867385, 1.000000000000000000, 0.9238795325112867385, 1.000000000000000000, 0.9238795325112867385, 1.000000000000000000, 0.9238795325112867385, 1.000000000000000000, 0.9238795325112867385, 1.000000000000000000, 0.9238795325112867385, 1.000000000000000000, 0.9238795325112867385, 1.000000000000000000, 0.9238795325112867385, 1.000000000000000000, 0.9238795325112867385, 1.000000000000000000, 0.9324258078851919151, 0.9848264816800302857 ) ) 
 REPRESENTATION_ITEM ( '' )  );
#5122=CARTESIAN_POINT ( 'NONE',  ( 5.622872871577871301, 32.81445312499999289, -13.57481594606304753 ) ) ;
#5123=CARTESIAN_POINT ( 'NONE',  ( 139.2950502721270425, 34.69960937608393436, 9.295050272127046043 ) ) ;
#5124=EDGE_LOOP ( 'NONE', ( #18452, #7101 ) ) ;
#5125=CARTESIAN_POINT ( 'NONE',  ( 103.5355339059327093, 81.62500000000000000, -3.535533905932755072 ) ) ;
#5126=CARTESIAN_POINT ( 'NONE',  ( 70.62287287157791127, 38.17226562716787441, 13.57481594606301023 ) ) ;
#5127=CARTESIAN_POINT ( 'NONE',  ( 104.4587341249999639, 82.93750000136560629, -1.442382525525748735E-14 ) ) ;
#5129=CARTESIAN_POINT ( 'NONE',  ( 78.57481594606304043, 39.16445312716788152, -5.622872871577873077 ) ) ;
#5132=CARTESIAN_POINT ( 'NONE',  ( 55.70494972787295751, 32.71523437608393436, -9.295050272127046043 ) ) ;
#5133=CARTESIAN_POINT ( 'NONE',  ( 74.29505027212704249, 36.28710937608393294, 9.295050272127046043 ) ) ;
#5134=VERTEX_POINT ( 'NONE', #27021 ) ;
#5140=CARTESIAN_POINT ( 'NONE',  ( 181.4251840539369596, 35.59257812716788294, 5.622872871577880183 ) ) ;
#5141=EDGE_CURVE ( 'NONE', #15733, #506, #16161, .T. ) ;
#5146=CARTESIAN_POINT ( 'NONE',  ( 13.14518615778179900, 35.54296875108394715, 5.444914386472293977 ) ) ;
#5147=EDGE_CURVE ( 'NONE', #22018, #747, #14312, .T. ) ;
#5160=CARTESIAN_POINT ( 'NONE',  ( 13.14518615778179900, 34.74921875108395142, 5.444914386472293977 ) ) ;
#5162=EDGE_CURVE ( 'NONE', #5134, #18802, #7382, .T. ) ;
#5166=CARTESIAN_POINT ( 'NONE',  ( 181.8548138422182205, 37.37851562608393863, 0.000000000000000000 ) ) ;
#5168=CARTESIAN_POINT ( 'NONE',  ( 5.622872871577863307, 39.75976562716787299, 13.57481594606306174 ) ) ;
#5171=ORIENTED_EDGE ( 'NONE', *, *, #3048, .F. ) ;
#5175=DIRECTION ( 'NONE',  ( -1.000000000000000000, 0.000000000000000000, 2.385244779468110248E-16 ) ) ;
#5176=CARTESIAN_POINT ( 'NONE',  ( 120.7049497278729575, 39.06523437608392868, 9.295050272127047819 ) ) ;
#5177=CARTESIAN_POINT ( 'NONE',  ( -5.444914386472299306, 36.93203125108394147, 13.14518615778179722 ) ) ;
#5179=CARTESIAN_POINT ( 'NONE',  ( 9.295050272127047819, 36.88242187608393152, 9.295050272127046043 ) ) ;
#5182=CARTESIAN_POINT ( 'NONE',  ( -13.57481594606304576, 36.33671875216787583, 0.000000000000000000 ) ) ;
#5185=CARTESIAN_POINT ( 'NONE',  ( 77.00957333851108899, 35.99999999999999289, 5.901833544882738813 ) ) ;
#5188=CARTESIAN_POINT ( 'NONE',  ( 51.85481384221821344, 38.22187500108393721, 5.444914386472304635 ) ) ;
#5190=CARTESIAN_POINT ( 'NONE',  ( 200.9085077471931413, 36.04503594658366694, 12.68159279706094367 ) ) ;
#5192=VERTEX_POINT ( 'NONE', #7617 ) ;
#5195=CARTESIAN_POINT ( 'NONE',  ( 189.5550856135277229, 37.72578125108394431, 13.14518615778179722 ) ) ;
#5201=CARTESIAN_POINT ( 'NONE',  ( 130.0000000000000000, 33.01289062608393721, 13.14518615778179544 ) ) ;
#5202=CARTESIAN_POINT ( 'NONE',  ( 70.44491438647229131, 40.50390625108394005, -13.14518615778179722 ) ) ;
#5204=CARTESIAN_POINT ( 'NONE',  ( 181.8548138422181921, 34.35234375108393579, -5.444914386472297529 ) ) ;
#5207=CARTESIAN_POINT ( 'NONE',  ( 3.863925265119776853, 54.10645156200111927, -15.00000000000000000 ) ) ;
#5210=CARTESIAN_POINT ( 'NONE',  ( 116.4251840539369454, 37.87460937716787868, -5.622872871577873077 ) ) ;
#5214=CARTESIAN_POINT ( 'NONE',  ( 185.7049497278729575, 40.05742187608393579, 9.295050272127047819 ) ) ;
#5216=SURFACE_STYLE_FILL_AREA ( #19890 ) ;
#5218=ORIENTED_EDGE ( 'NONE', *, *, #2230, .F. ) ;
#5219=CARTESIAN_POINT ( 'NONE',  ( -11.93524237669063126, 36.00000000000001421, -5.809862729998008568 ) ) ;
#5221=CARTESIAN_POINT ( 'NONE',  ( 133.6364962467980035, 51.46815297079191254, 14.99999999999789857 ) ) ;
#5223=CARTESIAN_POINT ( 'NONE',  ( 59.55508561352770158, 32.96328125108393436, 13.14518615778179722 ) ) ;
#5225=FACE_OUTER_BOUND ( 'NONE', #26873, .T. ) ;
#5226=CARTESIAN_POINT ( 'NONE',  ( 2.493653234604083739E-15, 40.40468749999999432, 13.57481594606304576 ) ) ;
#5227=CARTESIAN_POINT ( 'NONE',  ( 65.00000000000000000, -7.395377635281828788, -7.517135062566165128E-15 ) ) ;
#5228=CARTESIAN_POINT ( 'NONE',  ( -9.180175813647988292, 50.00000000000000711, 15.00000000000000355 ) ) ;
#5229=CARTESIAN_POINT ( 'NONE',  ( 51.42518405393695957, 40.95039062499999005, -5.622872871577872189 ) ) ;
#5230=CARTESIAN_POINT ( 'NONE',  ( 116.4251840539369596, 33.11210937499999574, 5.622872871577880183 ) ) ;
#5232=CARTESIAN_POINT ( 'NONE',  ( -15.00000000000000178, 75.00000000000000000, 1.734723475976807489E-15 ) ) ;
#5235=( BOUNDED_SURFACE ( )  B_SPLINE_SURFACE ( 1, 2, ( 
 ( #21520, #19517, #27664, #28078, #15217, #16822, #4416, #8126, #25518, #12799, #5997, #4136, #14662, #10666, #27938, #21245, #10388, #8260, #8397, #16947, #17086, #19374, #25648, #6132, #14797, #23521, #25789, #14939, #8542, #17228, #22087, #2426, #11227, #15656, #13214, #26652, #15933, #19943, #2564, #568, #422, #13508, #9108, #26214, #2841, #17802, #15798, #26506, #24356, #4699, #6962, #9385, #13653, #24501, #4845, #24650, #22229, #2708, #4554, #11368, #13070, #20090, #17654, #9250, #10943, #13360, #8823, #18082, #19655, #4988, #280, #21807, #2285, #17942, #7100, #11086, #21948, #22368, #20228, #24220, #11509, #710, #26795, #6675, #137, #7241, #17513, #15362, #24076, #19796, #8966, #26362, #6820, #15510, #16077, #16513, #11938, #1145, #27362, #5557, #25206, #13790, #12073, #9943, #860, #3551, #18658, #11652, #25070, #7821, #16369, #16650, #22940, #16227, #18230, #20375, #9532, #14081, #5692, #24927, #14222, #24785, #5123, #27079, #26940, #7384, #5413, #9812, #12208, #22801, #22659, #3270, #7677, #5266, #14359, #7952, #20660, #18518, #20798, #27223, #3403, #1278, #13932, #23075, #20935, #1419, #10078, #18790, #27497, #22511, #2977, #3131, #11797, #20520, #1002, #9671, #18374, #7531, #25485, #1695, #10497, #23627, #10213, #14631, #21072, #19341, #10635, #14767, #23486, #12483, #8651, #8091, #16786, #27769, #8512, #12898, #25617, #12627, #28181, #25345, #3967, #10352, #8367 ),
 ( #25756, #18923, #12354, #27906, #6100, #1967, #17052, #28045, #21353, #5830, #14498, #25902, #5963, #17195, #1833, #19204, #6372, #6238, #15045, #23215, #4103, #23762, #1560, #4239, #21629, #3690, #14906, #2104, #12768, #27631, #21486, #8227, #23350, #3823, #21210, #10772, #19483, #16917, #19061, #105, #17340, #11051, #2251, #23901, #243, #13325, #15760, #26326, #6643, #15471, #19907, #17476, #2670, #20192, #24185, #6786, #4807, #4663, #17768, #22052, #10912, #7063, #2526, #20053, #11188, #390, #8929, #9072, #13613, #17906, #531, #26471, #677, #15183, #24466, #6925, #26177, #21917, #15619, #24321, #19622, #15329, #13037, #11331, #9212, #13465, #22190, #4520, #26037, #8788, #24044, #19760, #26616, #4949, #17618, #22336, #6507, #4381, #2806, #2392, #11473, #13178, #21773, #1105, #822, #18481, #12169, #20619, #13895, #7491, #7200, #962, #5090, #5652, #15895, #20757, #24749, #20898, #18043, #16187, #14041, #7347, #9490, #1242, #14181, #9772, #22898, #18337, #9352, #26758, #9905, #20335, #18618, #24893, #5374, #3362, #27188, #27323, #24612, #16333, #12034, #13752, #7780, #16467, #22477, #7639, #25161, #25031, #2941, #5514, #20483, #11612, #18191, #26901, #27044, #14315, #9632, #23037, #16038, #5230, #3091, #22621, #11758, #22764, #3229, #3508, #11896, #18881, #27732, #3927, #1517, #14870, #4203, #8192, #10311, #17014, #19018, #1794, #16882, #14457, #19308, #25581, #4068 ) ),
 .UNSPECIFIED., .F., .F., .T. ) 
 B_SPLINE_SURFACE_WITH_KNOTS ( ( 2, 2 ),
 ( 3, 2, 2, 2, 2, 2, 2, 2, 2, 2, 2, 2, 2, 2, 2, 2, 2, 2, 2, 2, 2, 2, 2, 2, 2, 2, 2, 2, 2, 2, 2, 2, 2, 2, 2, 2, 2, 2, 2, 2, 2, 2, 2, 2, 2, 2, 2, 2, 2, 2, 2, 2, 2, 2, 2, 2, 2, 2, 2, 2, 2, 2, 2, 2, 2, 2, 2, 2, 2, 2, 2, 2, 2, 2, 2, 2, 2, 2, 2, 2, 2, 2, 2, 2, 2, 2, 2, 2, 2, 2, 2, 3 ),
 ( 0.000000000000000000, 1.000000000000000000 ),
 ( 0.000000000000000000, 0.01041666666666666609, 0.02083333333333333218, 0.03125000000000000000, 0.04166666666666666435, 0.05208333333333333565, 0.06250000000000000000, 0.07291666666666667129, 0.08333333333333332871, 0.09375000000000000000, 0.1041666666666666713, 0.1145833333333333287, 0.1250000000000000000, 0.1354166666666666574, 0.1458333333333333426, 0.1562500000000000000, 0.1666666666666666574, 0.1770833333333333426, 0.1875000000000000000, 0.1979166666666666574, 0.2083333333333333426, 0.2187500000000000000, 0.2291666666666666574, 0.2395833333333333426, 0.2500000000000000000, 0.2604166666666666852, 0.2708333333333333148, 0.2812500000000000000, 0.2916666666666666852, 0.3020833333333333148, 0.3125000000000000000, 0.3229166666666666852, 0.3333333333333333148, 0.3437500000000000000, 0.3541666666666666852, 0.3645833333333333148, 0.3750000000000000000, 0.3854166666666666852, 0.3958333333333333148, 0.4062500000000000000, 0.4166666666666666852, 0.4270833333333333148, 0.4375000000000000000, 0.4479166666666666852, 0.4583333333333333148, 0.4687500000000000000, 0.4791666666666666852, 0.4895833333333333148, 0.5000000000000000000, 0.5104166666666666297, 0.5208333333333333703, 0.5312500000000000000, 0.5416666666666666297, 0.5520833333333333703, 0.5625000000000000000, 0.5729166666666666297, 0.5833333333333333703, 0.5937500000000000000, 0.6041666666666666297, 0.6145833333333333703, 0.6250000000000000000, 0.6354166666666666297, 0.6458333333333333703, 0.6562500000000000000, 0.6666666666666666297, 0.6770833333333333703, 0.6875000000000000000, 0.6979166666666666297, 0.7083333333333333703, 0.7187500000000000000, 0.7291666666666666297, 0.7395833333333333703, 0.7500000000000000000, 0.7604166666666666297, 0.7708333333333333703, 0.7812500000000000000, 0.7916666666666666297, 0.8020833333333333703, 0.8125000000000000000, 0.8229166666666666297, 0.8333333333333333703, 0.8437500000000000000, 0.8541666666666666297, 0.8645833333333333703, 0.8750000000000000000, 0.8854166666666666297, 0.8958333333333333703, 0.9062500000000000000, 0.9166666666666666297, 0.9270833333333333703, 0.9375000000000000000, 0.9448586968893691873 ),
 .UNSPECIFIED. ) 
 GEOMETRIC_REPRESENTATION_ITEM ( )  RATIONAL_B_SPLINE_SURFACE ( (
 ( 1.000000000000000000, 0.9238795325112867385, 1.000000000000000000, 0.9238795325112867385, 1.000000000000000000, 0.9238795325112867385, 1.000000000000000000, 0.9238795325112867385, 1.000000000000000000, 0.9238795325112867385, 1.000000000000000000, 0.9238795325112867385, 1.000000000000000000, 0.9238795325112867385, 1.000000000000000000, 0.9238795325112867385, 1.000000000000000000, 0.9238795325112867385, 1.000000000000000000, 0.9238795325112867385, 1.000000000000000000, 0.9238795325112867385, 1.000000000000000000, 0.9238795325112867385, 1.000000000000000000, 0.9238795325112867385, 1.000000000000000000, 0.9238795325112867385, 1.000000000000000000, 0.9238795325112867385, 1.000000000000000000, 0.9238795325112867385, 1.000000000000000000, 0.9238795325112867385, 1.000000000000000000, 0.9238795325112867385, 1.000000000000000000, 0.9238795325112867385, 1.000000000000000000, 0.9238795325112867385, 1.000000000000000000, 0.9238795325112867385, 1.000000000000000000, 0.9238795325112867385, 1.000000000000000000, 0.9238795325112867385, 1.000000000000000000, 0.9238795325112867385, 1.000000000000000000, 0.9238795325112867385, 1.000000000000000000, 0.9238795325112867385, 1.000000000000000000, 0.9238795325112867385, 1.000000000000000000, 0.9238795325112867385, 1.000000000000000000, 0.9238795325112867385, 1.000000000000000000, 0.9238795325112867385, 1.000000000000000000, 0.9238795325112867385, 1.000000000000000000, 0.9238795325112867385, 1.000000000000000000, 0.9238795325112867385, 1.000000000000000000, 0.9238795325112867385, 1.000000000000000000, 0.9238795325112867385, 1.000000000000000000, 0.9238795325112867385, 1.000000000000000000, 0.9238795325112867385, 1.000000000000000000, 0.9238795325112867385, 1.000000000000000000, 0.9238795325112867385, 1.000000000000000000, 0.9238795325112867385, 1.000000000000000000, 0.9238795325112867385, 1.000000000000000000, 0.9238795325112867385, 1.000000000000000000, 0.9238795325112867385, 1.000000000000000000, 0.9238795325112867385, 1.000000000000000000, 0.9238795325112867385, 1.000000000000000000, 0.9238795325112867385, 1.000000000000000000, 0.9238795325112867385, 1.000000000000000000, 0.9238795325112867385, 1.000000000000000000, 0.9238795325112867385, 1.000000000000000000, 0.9238795325112867385, 1.000000000000000000, 0.9238795325112867385, 1.000000000000000000, 0.9238795325112867385, 1.000000000000000000, 0.9238795325112867385, 1.000000000000000000, 0.9238795325112867385, 1.000000000000000000, 0.9238795325112867385, 1.000000000000000000, 0.9238795325112867385, 1.000000000000000000, 0.9238795325112867385, 1.000000000000000000, 0.9238795325112867385, 1.000000000000000000, 0.9238795325112867385, 1.000000000000000000, 0.9238795325112867385, 1.000000000000000000, 0.9238795325112867385, 1.000000000000000000, 0.9238795325112867385, 1.000000000000000000, 0.9238795325112867385, 1.000000000000000000, 0.9238795325112867385, 1.000000000000000000, 0.9238795325112867385, 1.000000000000000000, 0.9238795325112867385, 1.000000000000000000, 0.9238795325112867385, 1.000000000000000000, 0.9238795325112867385, 1.000000000000000000, 0.9238795325112867385, 1.000000000000000000, 0.9238795325112867385, 1.000000000000000000, 0.9238795325112867385, 1.000000000000000000, 0.9238795325112867385, 1.000000000000000000, 0.9238795325112867385, 1.000000000000000000, 0.9238795325112867385, 1.000000000000000000, 0.9238795325112867385, 1.000000000000000000, 0.9238795325112867385, 1.000000000000000000, 0.9238795325112867385, 1.000000000000000000, 0.9238795325112867385, 1.000000000000000000, 0.9238795325112867385, 1.000000000000000000, 0.9238795325112867385, 1.000000000000000000, 0.9238795325112867385, 1.000000000000000000, 0.9238795325112867385, 1.000000000000000000, 0.9238795325112867385, 1.000000000000000000, 0.9238795325112867385, 1.000000000000000000, 0.9238795325112867385, 1.000000000000000000, 0.9238795325112867385, 1.000000000000000000, 0.9238795325112867385, 1.000000000000000000, 0.9238795325112867385, 1.000000000000000000, 0.9238795325112867385, 1.000000000000000000, 0.9238795325112867385, 1.000000000000000000, 0.9462258450566536361, 0.9684275698016389100),
 ( 1.000000000000000000, 0.9238795325112867385, 1.000000000000000000, 0.9238795325112867385, 1.000000000000000000, 0.9238795325112867385, 1.000000000000000000, 0.9238795325112867385, 1.000000000000000000, 0.9238795325112867385, 1.000000000000000000, 0.9238795325112867385, 1.000000000000000000, 0.9238795325112867385, 1.000000000000000000, 0.9238795325112867385, 1.000000000000000000, 0.9238795325112867385, 1.000000000000000000, 0.9238795325112867385, 1.000000000000000000, 0.9238795325112867385, 1.000000000000000000, 0.9238795325112867385, 1.000000000000000000, 0.9238795325112867385, 1.000000000000000000, 0.9238795325112867385, 1.000000000000000000, 0.9238795325112867385, 1.000000000000000000, 0.9238795325112867385, 1.000000000000000000, 0.9238795325112867385, 1.000000000000000000, 0.9238795325112867385, 1.000000000000000000, 0.9238795325112867385, 1.000000000000000000, 0.9238795325112867385, 1.000000000000000000, 0.9238795325112867385, 1.000000000000000000, 0.9238795325112867385, 1.000000000000000000, 0.9238795325112867385, 1.000000000000000000, 0.9238795325112867385, 1.000000000000000000, 0.9238795325112867385, 1.000000000000000000, 0.9238795325112867385, 1.000000000000000000, 0.9238795325112867385, 1.000000000000000000, 0.9238795325112867385, 1.000000000000000000, 0.9238795325112867385, 1.000000000000000000, 0.9238795325112867385, 1.000000000000000000, 0.9238795325112867385, 1.000000000000000000, 0.9238795325112867385, 1.000000000000000000, 0.9238795325112867385, 1.000000000000000000, 0.9238795325112867385, 1.000000000000000000, 0.9238795325112867385, 1.000000000000000000, 0.9238795325112867385, 1.000000000000000000, 0.9238795325112867385, 1.000000000000000000, 0.9238795325112867385, 1.000000000000000000, 0.9238795325112867385, 1.000000000000000000, 0.9238795325112867385, 1.000000000000000000, 0.9238795325112867385, 1.000000000000000000, 0.9238795325112867385, 1.000000000000000000, 0.9238795325112867385, 1.000000000000000000, 0.9238795325112867385, 1.000000000000000000, 0.9238795325112867385, 1.000000000000000000, 0.9238795325112867385, 1.000000000000000000, 0.9238795325112867385, 1.000000000000000000, 0.9238795325112867385, 1.000000000000000000, 0.9238795325112867385, 1.000000000000000000, 0.9238795325112867385, 1.000000000000000000, 0.9238795325112867385, 1.000000000000000000, 0.9238795325112867385, 1.000000000000000000, 0.9238795325112867385, 1.000000000000000000, 0.9238795325112867385, 1.000000000000000000, 0.9238795325112867385, 1.000000000000000000, 0.9238795325112867385, 1.000000000000000000, 0.9238795325112867385, 1.000000000000000000, 0.9238795325112867385, 1.000000000000000000, 0.9238795325112867385, 1.000000000000000000, 0.9238795325112867385, 1.000000000000000000, 0.9238795325112867385, 1.000000000000000000, 0.9238795325112867385, 1.000000000000000000, 0.9238795325112867385, 1.000000000000000000, 0.9238795325112867385, 1.000000000000000000, 0.9238795325112867385, 1.000000000000000000, 0.9238795325112867385, 1.000000000000000000, 0.9238795325112867385, 1.000000000000000000, 0.9238795325112867385, 1.000000000000000000, 0.9238795325112867385, 1.000000000000000000, 0.9238795325112867385, 1.000000000000000000, 0.9238795325112867385, 1.000000000000000000, 0.9238795325112867385, 1.000000000000000000, 0.9238795325112867385, 1.000000000000000000, 0.9238795325112867385, 1.000000000000000000, 0.9238795325112867385, 1.000000000000000000, 0.9238795325112867385, 1.000000000000000000, 0.9238795325112867385, 1.000000000000000000, 0.9238795325112867385, 1.000000000000000000, 0.9238795325112867385, 1.000000000000000000, 0.9238795325112867385, 1.000000000000000000, 0.9238795325112867385, 1.000000000000000000, 0.9238795325112867385, 1.000000000000000000, 0.9238795325112867385, 1.000000000000000000, 0.9238795325112867385, 1.000000000000000000, 0.9238795325112867385, 1.000000000000000000, 0.9238795325112867385, 1.000000000000000000, 0.9238795325112867385, 1.000000000000000000, 0.9238795325112867385, 1.000000000000000000, 0.9238795325112867385, 1.000000000000000000, 0.9238795325112867385, 1.000000000000000000, 0.9462258450566536361, 0.9684275698016389100) ) ) 
 REPRESENTATION_ITEM ( '' )  SURFACE ( )  );
#5237=CARTESIAN_POINT ( 'NONE',  ( 116.8548138422182063, 32.56640625108394005, -5.444914386472297529 ) ) ;
#5238=CARTESIAN_POINT ( 'NONE',  ( 65.00000000000000000, 31.37578125216787583, -13.57481594606304576 ) ) ;
#5239=DIRECTION ( 'NONE',  ( -0.000000000000000000, 1.000000000000000000, -0.000000000000000000 ) ) ;
#5240=CARTESIAN_POINT ( 'NONE',  ( -5.444914386472299306, 37.52734375108393294, 13.14518615778179722 ) ) ;
#5246=CARTESIAN_POINT ( 'NONE',  ( 181.8548138422181921, 32.56640625108394005, -5.444914386472297529 ) ) ;
#5250=CARTESIAN_POINT ( 'NONE',  ( 129.8277102352230656, 36.00000000000000000, -13.51468191220836523 ) ) ;
#5259=CARTESIAN_POINT ( 'NONE',  ( -8.312177448680279460E-16, 37.62656249999999858, -13.57481594606304576 ) ) ;
#5260=CARTESIAN_POINT ( 'NONE',  ( 95.54126587499995082, 82.37500000136562051, -1.846868145590750077 ) ) ;
#5261=CARTESIAN_POINT ( 'NONE',  ( 59.55508561352770158, 32.76484375108393010, 13.14518615778179722 ) ) ;
#5264=CARTESIAN_POINT ( 'NONE',  ( 13.57481594606304753, 37.47773437500001137, -5.622872871577873966 ) ) ;
#5265=CARTESIAN_POINT ( 'NONE',  ( -8.312177448680279460E-16, 32.86406249999999574, -13.57481594606304576 ) ) ;
#5266=CARTESIAN_POINT ( 'NONE',  ( 135.4449143864723055, 34.15390625108393863, -13.14518615778179900 ) ) ;
#5271=CARTESIAN_POINT ( 'NONE',  ( 98.15313185440925281, 83.25000000136560629, -4.458734125000016313 ) ) ;
#5273=CARTESIAN_POINT ( 'NONE',  ( 204.5988444088204403, 37.52734375000000000, -9.598844408820458085 ) ) ;
#5275=CARTESIAN_POINT ( 'NONE',  ( 189.5550856135277229, 39.80937500108392868, -13.14518615778179900 ) ) ;
#5276=CARTESIAN_POINT ( 'NONE',  ( 2.493653234604083739E-15, 38.91640625216786731, 13.57481594606304576 ) ) ;
#5279=ORIENTED_EDGE ( 'NONE', *, *, #899, .T. ) ;
#5280=CARTESIAN_POINT ( 'NONE',  ( 193.1834995827137504, 36.00000000000001421, -13.35830014193466653 ) ) ;
#5282=ORIENTED_EDGE ( 'NONE', *, *, #14339, .T. ) ;
#5284=CARTESIAN_POINT ( 'NONE',  ( 189.5550856135277229, 39.90859375108393436, 13.14518615778179722 ) ) ;
#5288=CARTESIAN_POINT ( 'NONE',  ( 9.295050272127046043, 33.31054687608394005, -9.295050272127046043 ) ) ;
#5289=( BOUNDED_CURVE ( )  B_SPLINE_CURVE ( 2, ( #22354, #26783, #267, #26639, #17500, #19642, #24207, #412, #7086 ),
 .UNSPECIFIED., .F., .T. ) 
 B_SPLINE_CURVE_WITH_KNOTS ( ( 3, 2, 2, 2, 3 ),
 ( 0.2708333333333330928, 0.2812499999999998890, 0.2916666666666666852, 0.3020833333333334259, 0.3125000000000002220 ),
 .UNSPECIFIED. ) 
 CURVE ( )  GEOMETRIC_REPRESENTATION_ITEM ( )  RATIONAL_B_SPLINE_CURVE ( ( 1.000000000000001554, 0.9238795325112850731, 1.000000000000000000, 0.9238795325112867385, 1.000000000000000000, 0.9238795325112867385, 1.000000000000000000, 0.9238795325112850731, 1.000000000000001554 ) ) 
 REPRESENTATION_ITEM ( '' )  );
#5290=CARTESIAN_POINT ( 'NONE',  ( 139.2950502721270425, 32.11992187608393579, 9.295050272127046043 ) ) ;
#5294=CARTESIAN_POINT ( 'NONE',  ( -13.36000105192242060, 40.87597656304196647, 0.000000000000000000 ) ) ;
#5301=DIRECTION ( 'NONE',  ( -0.000000000000000000, 1.000000000000000000, 0.000000000000000000 ) ) ;
#5303=CARTESIAN_POINT ( 'NONE',  ( 2.414731522848535132E-15, 34.60039062608393579, 13.14518615778179544 ) ) ;
#5310=CARTESIAN_POINT ( 'NONE',  ( 200.4449143864723055, 35.54296875108393294, -13.14518615778179900 ) ) ;
#5312=CARTESIAN_POINT ( 'NONE',  ( 193.1078166429076077, 53.66387243067951829, -15.00000000000000178 ) ) ;
#5314=ORIENTED_EDGE ( 'NONE', *, *, #24130, .T. ) ;
#5318=CARTESIAN_POINT ( 'NONE',  ( 195.0000000000000000, 38.51953125216787299, -13.57481594606304576 ) ) ;
#5319=CARTESIAN_POINT ( 'NONE',  ( 130.0000000000000000, -7.395377635281828788, -13.57481594606305997 ) ) ;
#5320=EDGE_CURVE ( 'NONE', #5488, #3371, #21257, .T. ) ;
#5321=CARTESIAN_POINT ( 'NONE',  ( 130.0000000000000000, 37.97382812608393721, -13.14518615778179544 ) ) ;
#5322=CARTESIAN_POINT ( 'NONE',  ( 13.14518615778179722, 36.43593750108394147, -5.444914386472297529 ) ) ;
#5323=CARTESIAN_POINT ( 'NONE',  ( 5.444914386472302859, 35.24531250108393010, 13.14518615778179189 ) ) ;
#5325=CARTESIAN_POINT ( 'NONE',  ( 73.21131401517213533, 50.68678854790645261, -15.00000000000000000 ) ) ;
#5330=CARTESIAN_POINT ( 'NONE',  ( 59.55508561352770158, 36.73359375108393010, 13.14518615778179722 ) ) ;
#5332=CARTESIAN_POINT ( 'NONE',  ( 51.42518405393695957, 38.66835937499999432, 5.622872871577880183 ) ) ;
#5333=CARTESIAN_POINT ( 'NONE',  ( 185.7049497278729575, 37.27929687608393294, -9.295050272127046043 ) ) ;
#5336=EDGE_CURVE ( 'NONE', #12117, #8914, #3398, .T. ) ;
#5338=CARTESIAN_POINT ( 'NONE',  ( 200.4449143864723055, 37.03125000108393294, 13.14518615778179189 ) ) ;
#5342=ORIENTED_EDGE ( 'NONE', *, *, #24287, .F. ) ;
#5343=CARTESIAN_POINT ( 'NONE',  ( 120.7049497278729575, 32.91367187608393152, 9.295050272127047819 ) ) ;
#5345=ADVANCED_FACE ( 'NONE', ( #4010 ), #28091, .T. ) ;
#5346=FACE_OUTER_BOUND ( 'NONE', #663, .T. ) ;
#5347=CARTESIAN_POINT ( 'NONE',  ( 208.1451861577817795, 34.05468750108394005, -5.444914386472297529 ) ) ;
#5348=ORIENTED_EDGE ( 'NONE', *, *, #7139, .T. ) ;
#5351=CARTESIAN_POINT ( 'NONE',  ( 120.8198241863519939, 49.99999999999998579, -14.99999999999999645 ) ) ;
#5352=VECTOR ( 'NONE', #24906, 1000.000000000000000 ) ;
#5354=CARTESIAN_POINT ( 'NONE',  ( 130.0000000000000000, 37.72578125216787726, -13.57481594606304576 ) ) ;
#5357=CARTESIAN_POINT ( 'NONE',  ( 68.97981444581395749, 50.00000000123263533, 13.01613927312710040 ) ) ;
#5361=CARTESIAN_POINT ( 'NONE',  ( -3.420220812170877700, 35.99999999999999289, -13.02105590829194348 ) ) ;
#5363=CARTESIAN_POINT ( 'NONE',  ( 139.1801758136480203, 55.00000000000000711, 14.99999999999996092 ) ) ;
#5365=CARTESIAN_POINT ( 'NONE',  ( 51.85481384221819923, 32.76484375108393010, -5.444914386472297529 ) ) ;
#5368=CARTESIAN_POINT ( 'NONE',  ( -5.622872871577839327, 38.76757812499998579, 13.57481594606308128 ) ) ;
#5372=CARTESIAN_POINT ( 'NONE',  ( -6.450879342660423177, 50.00000000106947340, 11.97362904075749235 ) ) ;
#5374=CARTESIAN_POINT ( 'NONE',  ( 139.5988444088204403, 34.35234374999999574, -9.598844408820458085 ) ) ;
#5376=CARTESIAN_POINT ( 'NONE',  ( -8.312177448680279460E-16, 40.10703125216787157, -13.57481594606304576 ) ) ;
#5380=CARTESIAN_POINT ( 'NONE',  ( 116.8548138422182063, 33.36015625108393579, -5.444914386472297529 ) ) ;
#5381=CARTESIAN_POINT ( 'NONE',  ( 55.40115559117954547, 31.47500000216787441, -9.598844408820458085 ) ) ;
#5383=CARTESIAN_POINT ( 'NONE',  ( -13.14518615778179189, 39.80937500108392868, 5.444914386472304635 ) ) ;
#5385=CARTESIAN_POINT ( 'NONE',  ( 195.0000000000000000, -7.395377635281828788, 13.57481594606302266 ) ) ;
#5387=ORIENTED_EDGE ( 'NONE', *, *, #24994, .F. ) ;
#5389=CARTESIAN_POINT ( 'NONE',  ( 189.5550856135277229, 31.97109375108393436, 13.14518615778179722 ) ) ;
#5390=CARTESIAN_POINT ( 'NONE',  ( 139.0314404224549207, 36.00000000000000000, 9.765766397118452957 ) ) ;
#5394=CARTESIAN_POINT ( 'NONE',  ( 118.3096217544866704, 36.00000000000001421, -6.307928093363107891 ) ) ;
#5401=CARTESIAN_POINT ( 'NONE',  ( 204.5988444088204687, 32.56640625000000000, 9.598844408820456309 ) ) ;
#5404=CARTESIAN_POINT ( 'NONE',  ( 104.4587341249999639, 83.93750000136560629, -1.442382525525748735E-14 ) ) ;
#5405=CARTESIAN_POINT ( 'NONE',  ( 78.14518615778179367, 32.21914062608393436, -1.609821015232357215E-15 ) ) ;
#5406=FACE_OUTER_BOUND ( 'NONE', #26194, .T. ) ;
#5409=ORIENTED_EDGE ( 'NONE', *, *, #25699, .F. ) ;
#5411=CARTESIAN_POINT ( 'NONE',  ( 214.9999999999999716, 80.00000000000000000, 9.999999999999946709 ) ) ;
#5413=CARTESIAN_POINT ( 'NONE',  ( 120.7049497278729575, 34.50117187608393721, 9.295050272127047819 ) ) ;
#5415=CARTESIAN_POINT ( 'NONE',  ( 94.99999999999995737, 81.00000000000000000, -1.387778780781445676E-14 ) ) ;
#5417=CARTESIAN_POINT ( 'NONE',  ( 97.92893218813451028, 79.31250000273121259, 4.999999999999989342 ) ) ;
#5419=CARTESIAN_POINT ( 'NONE',  ( 78.57481594606305464, 39.90859375216787441, -1.662435489736055892E-15 ) ) ;
#5422=CARTESIAN_POINT ( 'NONE',  ( 204.2950502721270425, 40.45429687608393721, -9.295050272127046043 ) ) ;
#5423=CARTESIAN_POINT ( 'NONE',  ( -13.57481594606304576, 37.92421875216787441, 0.000000000000000000 ) ) ;
#5428=CARTESIAN_POINT ( 'NONE',  ( 208.5748159460630120, 32.81445312716787299, -5.622872871577873077 ) ) ;
#5431=CARTESIAN_POINT ( 'NONE',  ( 124.5550856135277087, 39.90859375108392726, 13.14518615778179722 ) ) ;
#5432=CARTESIAN_POINT ( 'NONE',  ( 9.295050272127047819, 32.31835937608393294, 9.295050272127046043 ) ) ;
#5437=FACE_OUTER_BOUND ( 'NONE', #780, .T. ) ;
#5445=CARTESIAN_POINT ( 'NONE',  ( 219.9999999999999716, 50.00000000000000000, -10.00000000000000000 ) ) ;
#5446=CARTESIAN_POINT ( 'NONE',  ( -5.444914386472297529, 32.66562500108393863, -13.14518615778179900 ) ) ;
#5449=DIRECTION ( 'NONE',  ( 0.000000000000000000, -1.000000000000000000, 0.000000000000000000 ) ) ;
#5450=CARTESIAN_POINT ( 'NONE',  ( 208.1451861577817795, 33.75703125108393010, 5.444914386472293977 ) ) ;
#5451=ORIENTED_EDGE ( 'NONE', *, *, #6166, .T. ) ;
#5452=CARTESIAN_POINT ( 'NONE',  ( 185.8198241863519513, 50.00000000000000000, -9.999999999999960920 ) ) ;
#5454=ORIENTED_EDGE ( 'NONE', *, *, #26500, .T. ) ;
#5459=CARTESIAN_POINT ( 'NONE',  ( 2.493653234604083739E-15, 38.81718749999999574, 13.57481594606304576 ) ) ;
#5460=CARTESIAN_POINT ( 'NONE',  ( 116.8548138422182063, 38.12265625108393152, -5.444914386472297529 ) ) ;
#5461=CARTESIAN_POINT ( 'NONE',  ( -13.14518615778179544, 37.57695312608393579, 0.000000000000000000 ) ) ;
#5462=CARTESIAN_POINT ( 'NONE',  ( 13.14518615778179900, 40.30546875108393579, 5.444914386472293977 ) ) ;
#5465=EDGE_CURVE ( 'NONE', #152, #5192, #1153, .T. ) ;
#5469=CARTESIAN_POINT ( 'NONE',  ( 96.84719886470459471, 82.81250000136560629, 3.152801135295355994 ) ) ;
#5471=CARTESIAN_POINT ( 'NONE',  ( 61.88340791953426390, 53.90895096933308395, 14.99999999999998046 ) ) ;
#5472=CARTESIAN_POINT ( 'NONE',  ( 208.1451861577818079, 36.98164062608393010, -1.609821015232357215E-15 ) ) ;
#5473=VERTEX_POINT ( 'NONE', #296 ) ;
#5476=CARTESIAN_POINT ( 'NONE',  ( 195.0000000000000000, -7.395377635281828788, -2.255140518769849538E-14 ) ) ;
#5477=CARTESIAN_POINT ( 'NONE',  ( 208.1451861577818079, 36.43593750108394147, -5.444914386472297529 ) ) ;
#5479=AXIS2_PLACEMENT_3D ( 'NONE', #14592, #6197, #14867 ) ;
#5484=CARTESIAN_POINT ( 'NONE',  ( 195.0000000000000000, 37.32890625216786873, 13.57481594606304576 ) ) ;
#5485=DIRECTION ( 'NONE',  ( -0.000000000000000000, 1.000000000000000000, -0.000000000000000000 ) ) ;
#5486=CARTESIAN_POINT ( 'NONE',  ( 200.4449143864723055, 34.94765625108394147, -13.14518615778179900 ) ) ;
#5487=EDGE_CURVE ( 'NONE', #3022, #22301, #17987, .T. ) ;
#5488=VERTEX_POINT ( 'NONE', #834 ) ;
#5490=CARTESIAN_POINT ( 'NONE',  ( 6.161062174842293793, 51.27996893916987631, -14.99999999999999289 ) ) ;
#5491=CARTESIAN_POINT ( 'NONE',  ( 195.7197605961091824, 53.51499872091921617, 14.99999999999995026 ) ) ;
#5492=( BOUNDED_CURVE ( )  B_SPLINE_CURVE ( 2, ( #24043, #4238, #19759, #8928, #15182, #13464, #22051, #19482, #2525 ),
 .UNSPECIFIED., .F., .F. ) 
 B_SPLINE_CURVE_WITH_KNOTS ( ( 3, 2, 2, 2, 3 ),
 ( 0.4500000000000003997, 0.4750000000000003664, 0.5000000000000004441, 0.5250000000000004663, 0.5500000000000004885 ),
 .UNSPECIFIED. ) 
 CURVE ( )  GEOMETRIC_REPRESENTATION_ITEM ( )  RATIONAL_B_SPLINE_CURVE ( ( 0.9999999999999987788, 0.9238795325112879597, 1.000000000000000000, 0.9238795325112867385, 1.000000000000000000, 0.9238795325112867385, 1.000000000000000000, 0.9238795325112854062, 1.000000000000001332 ) ) 
 REPRESENTATION_ITEM ( '' )  );
#5493=CARTESIAN_POINT ( 'NONE',  ( 116.4251840539369454, 37.08085937716786873, -5.622872871577873077 ) ) ;
#5497=CARTESIAN_POINT ( 'NONE',  ( 208.1451861577817795, 37.13046875108393863, 5.444914386472293977 ) ) ;
#5498=ORIENTED_EDGE ( 'NONE', *, *, #10126, .T. ) ;
#5500=EDGE_CURVE ( 'NONE', #9895, #5976, #10183, .T. ) ;
#5504=LINE ( 'NONE', #12577, #12122 ) ;
#5506=CARTESIAN_POINT ( 'NONE',  ( -0.5932557025505245107, 35.99999999999998579, 13.13889047851773029 ) ) ;
#5507=CARTESIAN_POINT ( 'NONE',  ( 59.55508561352770158, 32.16953125108393152, 13.14518615778179722 ) ) ;
#5508=PRESENTATION_STYLE_ASSIGNMENT (( #3085 ) ) ;
#5513=CARTESIAN_POINT ( 'NONE',  ( -5.365496568044598291, 54.48174559707608466, 14.99999999999999645 ) ) ;
#5514=CARTESIAN_POINT ( 'NONE',  ( 135.6228728715778686, 33.60820312499998863, -13.57481594606304753 ) ) ;
#5515=ADVANCED_FACE ( 'NONE', ( #28115 ), #25827, .T. ) ;
#5516=VERTEX_POINT ( 'NONE', #23417 ) ;
#5521=CARTESIAN_POINT ( 'NONE',  ( 143.1451861577818079, 40.35507812608393863, -1.609821015232357215E-15 ) ) ;
#5522=CARTESIAN_POINT ( 'NONE',  ( 78.14518615778179367, 40.15664062608393436, -1.609821015232357215E-15 ) ) ;
#5524=CARTESIAN_POINT ( 'NONE',  ( 102.0710678118653760, 80.31250000000001421, 5.000000000000054179 ) ) ;
#5525=CARTESIAN_POINT ( 'NONE',  ( 9.295050272127047819, 40.05742187608392868, 9.295050272127046043 ) ) ;
#5527=LINE ( 'NONE', #22913, #26698 ) ;
#5533=CARTESIAN_POINT ( 'NONE',  ( 9.295050272127046043, 40.25585937608393294, -9.295050272127046043 ) ) ;
#5534=CARTESIAN_POINT ( 'NONE',  ( 138.1931556449105472, 36.00000000000000000, 10.45682415286355038 ) ) ;
#5537=( BOUNDED_CURVE ( )  B_SPLINE_CURVE ( 2, ( #26699, #7148, #15842, #24552, #5034 ),
 .UNSPECIFIED., .F., .T. ) 
 B_SPLINE_CURVE_WITH_KNOTS ( ( 3, 2, 3 ),
 ( 0.9500000000000009548, 0.9750000000000005329, 1.000000000000000000 ),
 .UNSPECIFIED. ) 
 CURVE ( )  GEOMETRIC_REPRESENTATION_ITEM ( )  RATIONAL_B_SPLINE_CURVE ( ( 0.9999999999999970024, 0.9238795325112897361, 1.000000000000000000, 0.9238795325112867385, 1.000000000000000000 ) ) 
 REPRESENTATION_ITEM ( '' )  );
#5542=ORIENTED_EDGE ( 'NONE', *, *, #18415, .F. ) ;
#5551=CARTESIAN_POINT ( 'NONE',  ( 70.44491438647230552, 40.50390625108394005, -13.14518615778179900 ) ) ;
#5554=CARTESIAN_POINT ( 'NONE',  ( 130.0000000000000000, 38.12265625216787157, 13.57481594606304576 ) ) ;
#5555=CARTESIAN_POINT ( 'NONE',  ( 5.622872871577878406, 32.51679687499999716, 13.57481594606304576 ) ) ;
#5557=CARTESIAN_POINT ( 'NONE',  ( 124.5550856135277087, 35.84062500108394289, -13.14518615778179900 ) ) ;
#5560=CYLINDRICAL_SURFACE ( 'NONE', #6796, 5.000000000000000888 ) ;
#5562=CARTESIAN_POINT ( 'NONE',  ( 99.99999999999995737, 83.68750000136560629, 4.458734124999988779 ) ) ;
#5563=CARTESIAN_POINT ( 'NONE',  ( 139.2950502721270425, 39.26367187608393294, 9.295050272127046043 ) ) ;
#5564=CARTESIAN_POINT ( 'NONE',  ( 55.40115559117954547, 39.41250000216787441, -9.598844408820458085 ) ) ;
#5566=CARTESIAN_POINT ( 'NONE',  ( 200.4449143864723055, 40.50390625108394005, -13.14518615778179900 ) ) ;
#5567=CARTESIAN_POINT ( 'NONE',  ( 2.493653234604083739E-15, 39.71015625216787015, 13.57481594606304576 ) ) ;
#5572=CARTESIAN_POINT ( 'NONE',  ( 208.5748159460630120, 32.02070312716787015, -5.622872871577873077 ) ) ;
#5580=CARTESIAN_POINT ( 'NONE',  ( 185.7049497278729575, 32.91367187608393152, 9.295050272127047819 ) ) ;
#5581=CARTESIAN_POINT ( 'NONE',  ( 120.2864525059511180, 35.99999999999999289, 8.898183052316758435 ) ) ;
#5583=CARTESIAN_POINT ( 'NONE',  ( -9.598844408820454532, 38.02343750216788010, 9.598844408820459861 ) ) ;
#5587=DIRECTION ( 'NONE',  ( -1.000000000000000000, -0.000000000000000000, -0.000000000000000000 ) ) ;
#5589=CARTESIAN_POINT ( 'NONE',  ( 13.14518615778179900, 32.36796875108393579, 5.444914386472293977 ) ) ;
#5593=AXIS2_PLACEMENT_3D ( 'NONE', #22743, #11878, #16449 ) ;
#5594=CARTESIAN_POINT ( 'NONE',  ( 185.7049497278729575, 34.10429687608393579, -9.295050272127046043 ) ) ;
#5596=CARTESIAN_POINT ( 'NONE',  ( 186.7403884711090143, 50.00000000056305538, -10.79618466885647265 ) ) ;
#5598=ORIENTED_EDGE ( 'NONE', *, *, #23880, .T. ) ;
#5601=CARTESIAN_POINT ( 'NONE',  ( 65.00000000000000000, 36.13828125216787157, -13.57481594606304576 ) ) ;
#5603=CARTESIAN_POINT ( 'NONE',  ( 5.444914386472302859, 38.61875000108392442, 13.14518615778179189 ) ) ;
#5604=CARTESIAN_POINT ( 'NONE',  ( 2.414731522848535132E-15, 40.15664062608393436, 13.14518615778179544 ) ) ;
#5611=CARTESIAN_POINT ( 'NONE',  ( 104.4587341249999781, 83.12500000136560629, 1.846868145590721655 ) ) ;
#5613=CARTESIAN_POINT ( 'NONE',  ( 65.00000000000000000, 38.91640625216786731, 13.57481594606304576 ) ) ;
#5614=CARTESIAN_POINT ( 'NONE',  ( 64.15789240453534603, 53.50112910130382460, 14.99999999999998224 ) ) ;
#5615=ORIENTED_EDGE ( 'NONE', *, *, #9353, .F. ) ;
#5618=LINE ( 'NONE', #3472, #18498 ) ;
#5620=CARTESIAN_POINT ( 'NONE',  ( -8.312177448680279460E-16, 40.00781250000000000, -13.57481594606304576 ) ) ;
#5622=EDGE_CURVE ( 'NONE', #8262, #16552, #2037, .T. ) ;
#5626=DIRECTION ( 'NONE',  ( 0.000000000000000000, 0.000000000000000000, -1.000000000000000000 ) ) ;
#5627=CARTESIAN_POINT ( 'NONE',  ( 59.55508561352770158, 39.31328125108392868, 13.14518615778179722 ) ) ;
#5628=CARTESIAN_POINT ( 'NONE',  ( 196.1371678245420753, 35.99999999999999289, 13.09590655363592582 ) ) ;
#5631=ORIENTED_EDGE ( 'NONE', *, *, #23286, .F. ) ;
#5633=CARTESIAN_POINT ( 'NONE',  ( -0.4460412567800353667, 49.99999999978076204, -13.57776691409236136 ) ) ;
#5635=CARTESIAN_POINT ( 'NONE',  ( 130.0000000000000000, 38.51953125216787299, -13.57481594606304576 ) ) ;
#5638=CARTESIAN_POINT ( 'NONE',  ( 181.8548138422181921, 37.52734375108393294, -5.444914386472297529 ) ) ;
#5642=DIRECTION ( 'NONE',  ( 0.000000000000000000, 0.000000000000000000, -1.000000000000000000 ) ) ;
#5649=CARTESIAN_POINT ( 'NONE',  ( 99.99999999999995737, 81.25000000000000000, 4.999999999999990230 ) ) ;
#5651=CARTESIAN_POINT ( 'NONE',  ( 94.99999999999995737, 83.06250000000001421, 2.071067811865466624 ) ) ;
#5652=CARTESIAN_POINT ( 'NONE',  ( 116.4251840539369454, 35.39414062499999147, -5.622872871577873077 ) ) ;
#5659=CARTESIAN_POINT ( 'NONE',  ( 120.7049497278729575, 39.85898437608393152, -9.295050272127046043 ) ) ;
#5660=EDGE_CURVE ( 'NONE', #17873, #27982, #19134, .T. ) ;
#5661=CARTESIAN_POINT ( 'NONE',  ( 70.44491438647230552, 37.92421875108392726, -13.14518615778179900 ) ) ;
#5663=CARTESIAN_POINT ( 'NONE',  ( 116.8548138422182205, 40.75195312608393294, 0.000000000000000000 ) ) ;
#5664=CARTESIAN_POINT ( 'NONE',  ( -9.295050272127044266, 39.06523437608392868, 9.295050272127047819 ) ) ;
#5666=CARTESIAN_POINT ( 'NONE',  ( 185.2864525059512459, 36.00000000000002132, 8.898183052316857911 ) ) ;
#5670=CARTESIAN_POINT ( 'NONE',  ( 135.3649479647156966, 36.00000000000000000, 12.09311862596028142 ) ) ;
#5672=EDGE_CURVE ( 'NONE', #1781, #22301, #13879, .T. ) ;
#5675=CYLINDRICAL_SURFACE ( 'NONE', #12667, 5.000000000000004441 ) ;
#5685=CARTESIAN_POINT ( 'NONE',  ( 95.54126587499995082, 80.50000000136560629, 1.846868145590724986 ) ) ;
#5686=CARTESIAN_POINT ( 'NONE',  ( 70.44491438647230552, 40.20625000108394431, 13.14518615778179189 ) ) ;
#5690=CARTESIAN_POINT ( 'NONE',  ( 130.0000000000000000, 38.81718749999999574, 13.57481594606304576 ) ) ;
#5692=CARTESIAN_POINT ( 'NONE',  ( 139.2950502721270425, 34.89804687608393863, -9.295050272127046043 ) ) ;
#5695=CARTESIAN_POINT ( 'NONE',  ( 143.5748159460630688, 37.57695312716787583, -5.622872871577873966 ) ) ;
#5697=CARTESIAN_POINT ( 'NONE',  ( 94.99999999999995737, 79.12500000273118417, -1.387778780781445676E-14 ) ) ;
#5698=CARTESIAN_POINT ( 'NONE',  ( 139.2950502721270425, 40.05742187608392868, 9.295050272127046043 ) ) ;
#5699=CARTESIAN_POINT ( 'NONE',  ( 51.42518405393695957, 40.25585937716787299, -5.622872871577873077 ) ) ;
#5700=VECTOR ( 'NONE', #1940, 1000.000000000000000 ) ;
#5702=CARTESIAN_POINT ( 'NONE',  ( -9.598844408820458085, 37.82500000216787583, -9.598844408820458085 ) ) ;
#5703=ORIENTED_EDGE ( 'NONE', *, *, #26777, .T. ) ;
#5707=( BOUNDED_CURVE ( )  B_SPLINE_CURVE ( 2, ( #14547, #25396, #9861, #13978, #14267, #5877, #20847, #18701, #5318 ),
 .UNSPECIFIED., .F., .T. ) 
 B_SPLINE_CURVE_WITH_KNOTS ( ( 3, 2, 2, 2, 3 ),
 ( 0.1458333333333336757, 0.1562500000000002776, 0.1666666666666669072, 0.1770833333333335369, 0.1875000000000001388 ),
 .UNSPECIFIED. ) 
 CURVE ( )  GEOMETRIC_REPRESENTATION_ITEM ( )  RATIONAL_B_SPLINE_CURVE ( ( 0.9999999999999975575, 0.9238795325112891810, 1.000000000000000000, 0.9238795325112867385, 1.000000000000000000, 0.9238795325112867385, 1.000000000000000000, 0.9238795325112857393, 1.000000000000001110 ) ) 
 REPRESENTATION_ITEM ( '' )  );
#5709=CARTESIAN_POINT ( 'NONE',  ( 195.0000000000000000, 39.16445312608392726, 13.14518615778179544 ) ) ;
#5710=CARTESIAN_POINT ( 'NONE',  ( 5.622872871577946796, 36.58476562716786873, 13.57481594606297115 ) ) ;
#5712=CARTESIAN_POINT ( 'NONE',  ( 135.4449143864723339, 39.21406250108392300, 13.14518615778179189 ) ) ;
#5713=CARTESIAN_POINT ( 'NONE',  ( -18.00000000000000711, 52.00000000000000711, 2.081668171172169302E-15 ) ) ;
#5714=PLANE ( 'NONE',  #7218 ) ;
#5717=CARTESIAN_POINT ( 'NONE',  ( 181.4251840539369596, 40.20624999999999005, 0.000000000000000000 ) ) ;
#5719=CARTESIAN_POINT ( 'NONE',  ( 51.42518405393695957, 39.46210937499999005, 5.622872871577880183 ) ) ;
#5722=VECTOR ( 'NONE', #12649, 1000.000000000000000 ) ;
#5727=CARTESIAN_POINT ( 'NONE',  ( 5.622872871577871301, 39.95820312499999716, -13.57481594606304753 ) ) ;
#5728=ORIENTED_EDGE ( 'NONE', *, *, #239, .T. ) ;
#5729=FACE_OUTER_BOUND ( 'NONE', #20241, .T. ) ;
#5730=AXIS2_PLACEMENT_3D ( 'NONE', #2444, #26237, #17677 ) ;
#5733=EDGE_LOOP ( 'NONE', ( #3451, #26022, #9175, #10773, #1680, #16736, #4317, #2748, #23807, #5598 ) ) ;
#5735=CARTESIAN_POINT ( 'NONE',  ( 199.0625835405769237, 50.00000000116060761, -12.98908657125174493 ) ) ;
#5737=ORIENTED_EDGE ( 'NONE', *, *, #17160, .F. ) ;
#5740=CARTESIAN_POINT ( 'NONE',  ( 208.5748159460630120, 39.95820312716787726, -5.622872871577873077 ) ) ;
#5742=CARTESIAN_POINT ( 'NONE',  ( -8.049105076161786076E-16, 38.17226562608394147, -13.14518615778179544 ) ) ;
#5743=CARTESIAN_POINT ( 'NONE',  ( 9.295050272127046043, 32.31835937608393294, -9.295050272127046043 ) ) ;
#5744=CARTESIAN_POINT ( 'NONE',  ( 59.37712712842213136, 39.26367187499999289, -13.57481594606304753 ) ) ;
#5745=VECTOR ( 'NONE', #16331, 1000.000000000000000 ) ;
#5747=ORIENTED_EDGE ( 'NONE', *, *, #24474, .F. ) ;
#5748=CARTESIAN_POINT ( 'NONE',  ( 78.57481594606305464, 38.17226562499999432, 5.622872871577868636 ) ) ;
#5751=CARTESIAN_POINT ( 'NONE',  ( 103.1528011352953342, 81.31250000136559208, -3.152801135295383084 ) ) ;
#5759=DIRECTION ( 'NONE',  ( 0.000000000000000000, 0.000000000000000000, 1.000000000000000000 ) ) ;
#5764=CARTESIAN_POINT ( 'NONE',  ( 74.29505027212704249, 38.86679687608393863, -9.295050272127046043 ) ) ;
#5766=CARTESIAN_POINT ( 'NONE',  ( -9.598844408820454532, 39.51171874999999289, 9.598844408820459861 ) ) ;
#5768=CARTESIAN_POINT ( 'NONE',  ( 74.59884440882045453, 37.52734375000000000, -9.598844408820458085 ) ) ;
#5770=CARTESIAN_POINT ( 'NONE',  ( 130.0000000000000000, 36.53515625216787299, 13.57481594606304576 ) ) ;
#5771=CARTESIAN_POINT ( 'NONE',  ( 135.6228728715778971, 33.40976562716787157, 13.57481594606304576 ) ) ;
#5774=CARTESIAN_POINT ( 'NONE',  ( 181.8548138422181921, 38.42031250108393436, 5.444914386472304635 ) ) ;
#5777=ORIENTED_EDGE ( 'NONE', *, *, #1705, .F. ) ;
#5779=AXIS2_PLACEMENT_3D ( 'NONE', #24021, #13299, #4500 ) ;
#5781=CARTESIAN_POINT ( 'NONE',  ( 5.622872871577796694, 39.95820312499999716, -13.57481594606312036 ) ) ;
#5783=CARTESIAN_POINT ( 'NONE',  ( 101.8468681455907046, 83.12500000136560629, -4.458734125000016313 ) ) ;
#5785=CARTESIAN_POINT ( 'NONE',  ( 130.0000000000000000, 40.10703125216787157, -13.57481594606304576 ) ) ;
#5787=CARTESIAN_POINT ( 'NONE',  ( 2.493653234604083739E-15, 38.81718749999999574, 13.57481594606304576 ) ) ;
#5788=CARTESIAN_POINT ( 'NONE',  ( 6.831134457304148810, 36.00000000000000000, 11.35217666746037501 ) ) ;
#5789=CARTESIAN_POINT ( 'NONE',  ( 130.0000000000000000, 50.00000000000000000, -1.503427012513233026E-14 ) ) ;
#5791=VERTEX_POINT ( 'NONE', #6999 ) ;
#5792=ORIENTED_EDGE ( 'NONE', *, *, #18415, .T. ) ;
#5799=CARTESIAN_POINT ( 'NONE',  ( 139.2950502721270425, 39.46210937608393721, 9.295050272127046043 ) ) ;
#5800=CARTESIAN_POINT ( 'NONE',  ( 51.85481384221819923, 35.74140625108393721, -5.444914386472297529 ) ) ;
#5801=ORIENTED_EDGE ( 'NONE', *, *, #6518, .T. ) ;
#5802=CARTESIAN_POINT ( 'NONE',  ( 55.88434273820531928, 36.00000000000001421, 9.510219181138525713 ) ) ;
#5803=CARTESIAN_POINT ( 'NONE',  ( 13.14518615778179900, 35.34453125108392868, 5.444914386472293977 ) ) ;
#5804=CARTESIAN_POINT ( 'NONE',  ( 55.40115559117954547, 36.33671874999999574, 9.598844408820459861 ) ) ;
#5806=DIRECTION ( 'NONE',  ( -0.000000000000000000, 1.000000000000000000, -0.000000000000000000 ) ) ;
#5807=CARTESIAN_POINT ( 'NONE',  ( -13.14518615778179900, 38.91640625108393436, -5.444914386472297529 ) ) ;
#5808=CARTESIAN_POINT ( 'NONE',  ( 142.2511908804447387, 36.00000000000001421, 5.405483146087447288 ) ) ;
#5811=CARTESIAN_POINT ( 'NONE',  ( 99.99999999999995737, 85.00000000000000000, -1.387778780781445676E-14 ) ) ;
#5812=CARTESIAN_POINT ( 'NONE',  ( -8.312177448680279460E-16, 38.42031249999999432, -13.57481594606304576 ) ) ;
#5814=CARTESIAN_POINT ( 'NONE',  ( 99.99999999999995737, 82.25000000000000000, 4.999999999999990230 ) ) ;
#5821=CARTESIAN_POINT ( 'NONE',  ( 95.54126587499995082, 79.50000000136560629, 1.846868145590724986 ) ) ;
#5822=CARTESIAN_POINT ( 'NONE',  ( 55.70494972787295751, 39.26367187608393294, 9.295050272127047819 ) ) ;
#5823=EDGE_CURVE ( 'NONE', #12988, #12573, #22944, .T. ) ;
#5825=CARTESIAN_POINT ( 'NONE',  ( -9.396418828207704684E-17, 52.00000000000000711, -12.99999999999999822 ) ) ;
#5830=CARTESIAN_POINT ( 'NONE',  ( 143.5748159460630404, 40.55351562499998863, 5.622872871577869525 ) ) ;
#5832=CARTESIAN_POINT ( 'NONE',  ( -8.392215291638379426, 54.99999999999999289, -14.99999999999999822 ) ) ;
#5836=CARTESIAN_POINT ( 'NONE',  ( 74.59884440882045453, 37.62656250216787157, -9.598844408820458085 ) ) ;
#5838=CARTESIAN_POINT ( 'NONE',  ( 13.57481594606304931, 38.27148437716787299, 5.622872871577869525 ) ) ;
#5841=EDGE_CURVE ( 'NONE', #8652, #26290, #23836, .T. ) ;
#5843=CARTESIAN_POINT ( 'NONE',  ( 200.4449143864723055, 40.30546875108393579, -13.14518615778179900 ) ) ;
#5845=CARTESIAN_POINT ( 'NONE',  ( 139.2950502721270425, 37.08085937608393579, -9.295050272127046043 ) ) ;
#5848=PLANE ( 'NONE',  #17407 ) ;
#5851=ADVANCED_FACE ( 'NONE', ( #13108 ), #26110, .T. ) ;
#5852=CARTESIAN_POINT ( 'NONE',  ( 181.4251840539369596, 36.98164062499999005, -5.622872871577873077 ) ) ;
#5856=CARTESIAN_POINT ( 'NONE',  ( 78.14518615778179367, 38.56914062608393579, -1.609821015232357215E-15 ) ) ;
#5860=CARTESIAN_POINT ( 'NONE',  ( 99.99999999999995737, 78.00000000000000000, -3.000000000000018208 ) ) ;
#5861=CARTESIAN_POINT ( 'NONE',  ( 65.00000000000000000, 36.00000000000000000, -7.517135062566165128E-15 ) ) ;
#5862=CARTESIAN_POINT ( 'NONE',  ( -13.57481594606304576, 39.41249999999999432, 0.000000000000000000 ) ) ;
#5866=DIRECTION ( 'NONE',  ( -1.000000000000000000, -1.387778780781407810E-15, 7.228014483236696740E-18 ) ) ;
#5867=DIRECTION ( 'NONE',  ( 0.000000000000000000, 0.000000000000000000, 1.000000000000000000 ) ) ;
#5872=CARTESIAN_POINT ( 'NONE',  ( 196.0141308260785706, 51.45790058219387220, -14.99999999999864642 ) ) ;
#5877=CARTESIAN_POINT ( 'NONE',  ( 181.4251840539369596, 38.66835937716787441, -5.622872871577872189 ) ) ;
#5881=CARTESIAN_POINT ( 'NONE',  ( 116.8548138422182205, 38.32109375108394289, -5.444914386472297529 ) ) ;
#5882=CARTESIAN_POINT ( 'NONE',  ( -13.14518615778179544, 32.61601562608393579, 0.000000000000000000 ) ) ;
#5884=VECTOR ( 'NONE', #22028, 1000.000000000000000 ) ;
#5885=CARTESIAN_POINT ( 'NONE',  ( 70.62287287157788285, 37.27929687499999289, 13.57481594606304576 ) ) ;
#5887=DIRECTION ( 'NONE',  ( 0.000000000000000000, 0.000000000000000000, -1.000000000000000000 ) ) ;
#5891=CARTESIAN_POINT ( 'NONE',  ( 98.15313185440923860, 82.50000000136560629, -4.458734125000016313 ) ) ;
#5893=CARTESIAN_POINT ( 'NONE',  ( 13.14518615778179900, 39.61093750108393863, -5.444914386472297529 ) ) ;
#5896=EDGE_LOOP ( 'NONE', ( #5064, #25393, #10460, #20794 ) ) ;
#5898=CARTESIAN_POINT ( 'NONE',  ( 0.000000000000000000, 50.00000000000000000, 0.000000000000000000 ) ) ;
#5904=( BOUNDED_CURVE ( )  B_SPLINE_CURVE ( 2, ( #26235, #11246, #6693, #7118, #19964 ),
 .UNSPECIFIED., .F., .F. ) 
 B_SPLINE_CURVE_WITH_KNOTS ( ( 3, 2, 3 ),
 ( 0.000000000000000000, 0.01041666666666679446, 0.02083333333333358892 ),
 .UNSPECIFIED. ) 
 CURVE ( )  GEOMETRIC_REPRESENTATION_ITEM ( )  RATIONAL_B_SPLINE_CURVE ( ( 1.000000000000000000, 0.9238795325112867385, 1.000000000000000000, 0.9238795325112848511, 1.000000000000001776 ) ) 
 REPRESENTATION_ITEM ( '' )  );
#5906=CARTESIAN_POINT ( 'NONE',  ( 70.44491438647229131, 38.12265625108393863, -13.14518615778179722 ) ) ;
#5907=CIRCLE ( 'NONE', #17257, 4.999999999999999112 ) ;
#5910=ORIENTED_EDGE ( 'NONE', *, *, #3900, .T. ) ;
#5912=CARTESIAN_POINT ( 'NONE',  ( -2.529583995168191990, 49.99999999938367523, -13.34625891065979353 ) ) ;
#5913=CARTESIAN_POINT ( 'NONE',  ( 130.0000000000000000, 36.93203125216787441, -13.57481594606304576 ) ) ;
#5914=CARTESIAN_POINT ( 'NONE',  ( 116.4251840539369596, 33.21132812716787441, 5.622872871577880183 ) ) ;
#5917=CARTESIAN_POINT ( 'NONE',  ( 185.7049497278729575, 39.06523437608392868, -9.295050272127046043 ) ) ;
#5921=CARTESIAN_POINT ( 'NONE',  ( 13.57481594606304931, 39.75976562499999289, 5.622872871577868636 ) ) ;
#5924=CARTESIAN_POINT ( 'NONE',  ( 143.5748159460630688, 39.85898437716787157, 5.622872871577868636 ) ) ;
#5926=CARTESIAN_POINT ( 'NONE',  ( 13.24545034676870969, 36.00000000000000000, 2.307131236161232835 ) ) ;
#5927=DIRECTION ( 'NONE',  ( 0.000000000000000000, -1.000000000000000000, 0.000000000000000000 ) ) ;
#5933=CARTESIAN_POINT ( 'NONE',  ( 143.1451861577818079, 37.97382812608393721, -1.609821015232357215E-15 ) ) ;
#5934=CARTESIAN_POINT ( 'NONE',  ( 59.55508561352770158, 35.64218750108392442, -13.14518615778179900 ) ) ;
#5936=CARTESIAN_POINT ( 'NONE',  ( 99.99999999999995737, 80.25000000000000000, 4.999999999999990230 ) ) ;
#5937=CARTESIAN_POINT ( 'NONE',  ( 2.414731522848535132E-15, 34.40195312608393152, 13.14518615778179544 ) ) ;
#5938=CARTESIAN_POINT ( 'NONE',  ( 181.8508260188482097, 35.99999999999998579, -1.058935892997001194 ) ) ;
#5942=CARTESIAN_POINT ( 'NONE',  ( -13.14518615778179544, 38.96601562608393721, 0.000000000000000000 ) ) ;
#5943=CARTESIAN_POINT ( 'NONE',  ( 143.0198548647682344, 35.99999999999997868, 3.369129432478993103 ) ) ;
#5945=CYLINDRICAL_SURFACE ( 'NONE', #20067, 13.57481594606304398 ) ;
#5951=VERTEX_POINT ( 'NONE', #10376 ) ;
#5954=DIRECTION ( 'NONE',  ( -0.000000000000000000, 1.000000000000000000, -0.000000000000000000 ) ) ;
#5956=CARTESIAN_POINT ( 'NONE',  ( 104.4587341249999781, 80.00000000136559208, -1.846868145590750299 ) ) ;
#5957=CARTESIAN_POINT ( 'NONE',  ( 59.55508561352770158, 39.31328125108394289, 13.14518615778179722 ) ) ;
#5959=DIRECTION ( 'NONE',  ( 0.000000000000000000, 0.000000000000000000, 1.000000000000000000 ) ) ;
#5961=CARTESIAN_POINT ( 'NONE',  ( 55.40115559117954547, 38.61875000216787157, -9.598844408820458085 ) ) ;
#5963=CARTESIAN_POINT ( 'NONE',  ( 130.0000000000000000, 40.40468749999999432, 13.57481594606304576 ) ) ;
#5965=CARTESIAN_POINT ( 'NONE',  ( 6.116560239716792857, 54.66944451632674173, -15.00000000000000000 ) ) ;
#5969=CARTESIAN_POINT ( 'NONE',  ( 59.37712712842213136, 37.77539062716788010, -13.57481594606304753 ) ) ;
#5970=EDGE_CURVE ( 'NONE', #10403, #152, #19083, .T. ) ;
#5971=AXIS2_PLACEMENT_3D ( 'NONE', #10755, #15025, #23745 ) ;
#5973=CARTESIAN_POINT ( 'NONE',  ( 9.598844408820456309, 34.45156250216787441, -9.598844408820458085 ) ) ;
#5974=ORIENTED_EDGE ( 'NONE', *, *, #15277, .F. ) ;
#5976=VERTEX_POINT ( 'NONE', #1986 ) ;
#5977=CARTESIAN_POINT ( 'NONE',  ( 65.00000000000000000, 36.00000000000000000, -7.517135062566165128E-15 ) ) ;
#5978=CARTESIAN_POINT ( 'NONE',  ( 189.5550856135277229, 38.02343750108394005, -13.14518615778179900 ) ) ;
#5980=CARTESIAN_POINT ( 'NONE',  ( 139.2950502721270425, 39.26367187608393294, 9.295050272127046043 ) ) ;
#5982=CARTESIAN_POINT ( 'NONE',  ( 51.63999894807758295, 40.87597656304196647, 0.000000000000000000 ) ) ;
#5987=CARTESIAN_POINT ( 'NONE',  ( 189.3771271284221314, 36.88242187499999858, -13.57481594606304753 ) ) ;
#5988=SHAPE_DEFINITION_REPRESENTATION ( #24710, #14045 ) ;
#5991=CARTESIAN_POINT ( 'NONE',  ( 55.70494972787295751, 38.86679687608393863, -9.295050272127046043 ) ) ;
#5996=CARTESIAN_POINT ( 'NONE',  ( 13.57481594606304576, 40.60312499999999858, -1.662435489736055892E-15 ) ) ;
#5997=CARTESIAN_POINT ( 'NONE',  ( 139.2950502721270425, 40.25585937608393294, 9.295050272127046043 ) ) ;
#5998=ORIENTED_EDGE ( 'NONE', *, *, #19646, .T. ) ;
#5999=CARTESIAN_POINT ( 'NONE',  ( 104.4587341249999781, 82.25000000136559208, -1.846868145590750299 ) ) ;
#6005=CARTESIAN_POINT ( 'NONE',  ( 139.1801758136479918, 55.00000000000000000, -15.00000000000000000 ) ) ;
#6008=ORIENTED_EDGE ( 'NONE', *, *, #15615, .T. ) ;
#6011=CARTESIAN_POINT ( 'NONE',  ( 208.5748159460630120, 37.57695312716787583, -5.622872871577873077 ) ) ;
#6013=EDGE_CURVE ( 'NONE', #3638, #7806, #18897, .T. ) ;
#6015=CARTESIAN_POINT ( 'NONE',  ( 197.0246277255383234, 50.00000000050969362, 13.43320860980889897 ) ) ;
#6016=CARTESIAN_POINT ( 'NONE',  ( 143.1451861577818363, 38.02343750108395426, -5.444914386472297529 ) ) ;
#6017=CARTESIAN_POINT ( 'NONE',  ( -13.14518615778179900, 32.56640625108394005, -5.444914386472297529 ) ) ;
#6018=VERTEX_POINT ( 'NONE', #19505 ) ;
#6019=CARTESIAN_POINT ( 'NONE',  ( 55.40115559117954547, 36.33671874999999574, 9.598844408820459861 ) ) ;
#6021=EDGE_CURVE ( 'NONE', #18802, #26308, #4144, .T. ) ;
#6022=CARTESIAN_POINT ( 'NONE',  ( 206.2065315021356753, 36.00000000000000000, 7.323573988460882589 ) ) ;
#6026=CARTESIAN_POINT ( 'NONE',  ( 96.84719886470459471, 82.56250000136559208, -3.152801135295383084 ) ) ;
#6028=CARTESIAN_POINT ( 'NONE',  ( 9.295050272127046043, 40.45429687608393721, -9.295050272127046043 ) ) ;
#6029=CARTESIAN_POINT ( 'NONE',  ( 195.0000000000000000, 38.42031249999999432, -13.57481594606304576 ) ) ;
#6036=EDGE_CURVE ( 'NONE', #11583, #21223, #3986, .T. ) ;
#6039=CARTESIAN_POINT ( 'NONE',  ( 51.85481384221820633, 39.16445312608393436, 0.000000000000000000 ) ) ;
#6041=CARTESIAN_POINT ( 'NONE',  ( 68.86541437541316668, 54.10683252460148651, -15.00000000000000178 ) ) ;
#6044=ADVANCED_FACE ( 'NONE', ( #27926 ), #23370, .T. ) ;
#6045=CARTESIAN_POINT ( 'NONE',  ( 181.6399989480775901, 40.87597656304196647, 0.000000000000000000 ) ) ;
#6046=CARTESIAN_POINT ( 'NONE',  ( 191.1345856245867765, 54.10683252460147230, 14.99999999999994493 ) ) ;
#6047=EDGE_CURVE ( 'NONE', #24596, #9425, #12919, .T. ) ;
#6049=CARTESIAN_POINT ( 'NONE',  ( 143.5748159460630688, 35.93984375216787441, -1.662435489736055892E-15 ) ) ;
#6051=CARTESIAN_POINT ( 'NONE',  ( 134.1572863549629062, 35.99999999999997868, -12.92256159328817411 ) ) ;
#6052=CARTESIAN_POINT ( 'NONE',  ( 130.0000000000000000, 37.72578125216787726, -13.57481594606304576 ) ) ;
#6053=CARTESIAN_POINT ( 'NONE',  ( 189.5550856135277229, 39.31328125108394289, 13.14518615778179722 ) ) ;
#6062=FACE_OUTER_BOUND ( 'NONE', #28198, .T. ) ;
#6065=ORIENTED_EDGE ( 'NONE', *, *, #8879, .T. ) ;
#6069=CARTESIAN_POINT ( 'NONE',  ( 135.4449143864723055, 38.91640625108393436, -13.14518615778179900 ) ) ;
#6070=CARTESIAN_POINT ( 'NONE',  ( 65.00000000000000000, 38.37070312608393152, 13.14518615778179544 ) ) ;
#6072=CARTESIAN_POINT ( 'NONE',  ( 189.5550856135277229, 40.60312500108393863, -13.14518615778179900 ) ) ;
#6073=PLANE ( 'NONE',  #25696 ) ;
#6074=CARTESIAN_POINT ( 'NONE',  ( 5.444914386472302859, 36.83281250108392868, 13.14518615778179189 ) ) ;
#6075=CARTESIAN_POINT ( 'NONE',  ( 65.00000000000000000, 36.03906250000000000, -13.57481594606304576 ) ) ;
#6077=CYLINDRICAL_SURFACE ( 'NONE', #8524, 13.57481594606304398 ) ;
#6078=CARTESIAN_POINT ( 'NONE',  ( -9.295050272127044266, 39.06523437608392868, 9.295050272127047819 ) ) ;
#6083=VECTOR ( 'NONE', #24732, 1000.000000000000000 ) ;
#6091=CARTESIAN_POINT ( 'NONE',  ( 99.99999999999995737, 80.25000000000000000, 4.999999999999990230 ) ) ;
#6092=CARTESIAN_POINT ( 'NONE',  ( 96.84719886470459471, 80.31250000136559208, -3.152801135295383084 ) ) ;
#6093=CARTESIAN_POINT ( 'NONE',  ( 55.70494972787295751, 38.27148437608393294, -9.295050272127046043 ) ) ;
#6096=VERTEX_POINT ( 'NONE', #14785 ) ;
#6097=DIRECTION ( 'NONE',  ( 0.000000000000000000, 0.000000000000000000, -1.000000000000000000 ) ) ;
#6098=FACE_OUTER_BOUND ( 'NONE', #8377, .T. ) ;
#6100=CARTESIAN_POINT ( 'NONE',  ( 130.0000000000000000, 40.80156249999999574, -13.57481594606304576 ) ) ;
#6101=ORIENTED_EDGE ( 'NONE', *, *, #13351, .T. ) ;
#6102=CARTESIAN_POINT ( 'NONE',  ( 3.116592080465746761, 53.90895096933311237, -15.00000000000000178 ) ) ;
#6105=CARTESIAN_POINT ( 'NONE',  ( 135.4449143864723055, 40.30546875108393579, -13.14518615778179900 ) ) ;
#6106=CARTESIAN_POINT ( 'NONE',  ( 74.59884440882045453, 37.42812500216787441, 9.598844408820456309 ) ) ;
#6108=CARTESIAN_POINT ( 'NONE',  ( 5.622872871577871301, 36.88242187716787157, -13.57481594606304753 ) ) ;
#6109=EDGE_LOOP ( 'NONE', ( #6544, #18119, #12285, #19575 ) ) ;
#6112=AXIS2_PLACEMENT_3D ( 'NONE', #7570, #5449, #10252 ) ;
#6113=CARTESIAN_POINT ( 'NONE',  ( 200.4449143864723055, 36.03906250108394005, 13.14518615778179189 ) ) ;
#6115=CARTESIAN_POINT ( 'NONE',  ( 139.2950502721270425, 37.87460937608393152, -9.295050272127046043 ) ) ;
#6118=DIRECTION ( 'NONE',  ( -0.000000000000000000, 1.000000000000000000, -0.000000000000000000 ) ) ;
#6121=CARTESIAN_POINT ( 'NONE',  ( 208.5748159460630120, 36.68398437499999432, -5.622872871577873077 ) ) ;
#6125=CARTESIAN_POINT ( 'NONE',  ( 51.85481384221820633, 39.75976562608393294, 0.000000000000000000 ) ) ;
#6128=DIRECTION ( 'NONE',  ( 0.000000000000000000, 0.000000000000000000, -1.000000000000000000 ) ) ;
#6131=CARTESIAN_POINT ( 'NONE',  ( -5.622872871577873077, 40.05742187499999574, -13.57481594606304753 ) ) ;
#6132=CARTESIAN_POINT ( 'NONE',  ( 143.1451861577818079, 39.61093750108393863, -5.444914386472297529 ) ) ;
#6134=CARTESIAN_POINT ( 'NONE',  ( 104.4587341249999639, 84.18750000136560629, -1.442382525525748735E-14 ) ) ;
#6136=ORIENTED_EDGE ( 'NONE', *, *, #14706, .T. ) ;
#6137=CARTESIAN_POINT ( 'NONE',  ( 130.0000000000000000, 38.91640625216786731, 13.57481594606304576 ) ) ;
#6138=CARTESIAN_POINT ( 'NONE',  ( 51.85481384221819923, 35.14609375108393152, -5.444914386472297529 ) ) ;
#6139=( BOUNDED_CURVE ( )  B_SPLINE_CURVE ( 2, ( #5785, #14452, #19161, #27865, #1646, #5924, #25857, #12858, #16879 ),
 .UNSPECIFIED., .F., .T. ) 
 B_SPLINE_CURVE_WITH_KNOTS ( ( 3, 2, 2, 2, 3 ),
 ( 0.02083333333333358892, 0.03125000000000020123, 0.04166666666666681007, 0.05208333333333342585, 0.06250000000000004163 ),
 .UNSPECIFIED. ) 
 CURVE ( )  GEOMETRIC_REPRESENTATION_ITEM ( )  RATIONAL_B_SPLINE_CURVE ( ( 0.9999999999999981126, 0.9238795325112886259, 1.000000000000000000, 0.9238795325112867385, 1.000000000000000000, 0.9238795325112867385, 1.000000000000000000, 0.9238795325112864054, 1.000000000000000222 ) ) 
 REPRESENTATION_ITEM ( '' )  );
#6140=ORIENTED_EDGE ( 'NONE', *, *, #8955, .T. ) ;
#6146=CARTESIAN_POINT ( 'NONE',  ( 208.5748159460630120, 39.06523437716786873, 5.622872871577869525 ) ) ;
#6149=CARTESIAN_POINT ( 'NONE',  ( 192.8300434168937727, 49.99999999883907975, 13.43548448457828037 ) ) ;
#6150=CARTESIAN_POINT ( 'NONE',  ( 139.2950502721270425, 38.66835937608393436, 9.295050272127046043 ) ) ;
#6151=CARTESIAN_POINT ( 'NONE',  ( 9.295050272127047819, 37.87460937608393863, 9.295050272127046043 ) ) ;
#6153=ORIENTED_EDGE ( 'NONE', *, *, #21226, .T. ) ;
#6154=CARTESIAN_POINT ( 'NONE',  ( 51.42518405393695957, 38.56914062500000284, -5.622872871577873077 ) ) ;
#6155=CYLINDRICAL_SURFACE ( 'NONE', #494, 13.57481594606304398 ) ;
#6156=CARTESIAN_POINT ( 'NONE',  ( 207.0095733385116716, 36.00000000000000711, 5.901833544881684546 ) ) ;
#6161=CARTESIAN_POINT ( 'NONE',  ( 103.1528011352953342, 80.06250000136559208, 3.152801135295355106 ) ) ;
#6163=CARTESIAN_POINT ( 'NONE',  ( 2.414731522848535132E-15, 40.15664062608393436, 13.14518615778179544 ) ) ;
#6165=ORIENTED_EDGE ( 'NONE', *, *, #22907, .T. ) ;
#6166=EDGE_CURVE ( 'NONE', #861, #18432, #24833, .T. ) ;
#6168=DIRECTION ( 'NONE',  ( -0.000000000000000000, 1.000000000000000000, -0.000000000000000000 ) ) ;
#6169=CARTESIAN_POINT ( 'NONE',  ( 94.99999999999995737, 81.06250000273119838, -2.071067811865491048 ) ) ;
#6171=VECTOR ( 'NONE', #1531, 1000.000000000000000 ) ;
#6174=CARTESIAN_POINT ( 'NONE',  ( 70.44491438647229131, 37.82500000108392868, 13.14518615778179189 ) ) ;
#6175=EDGE_CURVE ( 'NONE', #5976, #444, #2414, .T. ) ;
#6176=CARTESIAN_POINT ( 'NONE',  ( -13.57481594606304753, 39.36289062499999858, -5.622872871577872189 ) ) ;
#6179=CARTESIAN_POINT ( 'NONE',  ( -3.044609456930747804, 53.89089363584124470, -15.00000000000000000 ) ) ;
#6182=CARTESIAN_POINT ( 'NONE',  ( 124.3771271284221314, 33.80664062716786589, -13.57481594606304753 ) ) ;
#6183=CARTESIAN_POINT ( 'NONE',  ( 181.4251840539369596, 40.95039062499999005, -5.622872871577872189 ) ) ;
#6185=CARTESIAN_POINT ( 'NONE',  ( 181.8548138422181921, 35.24531250108393721, 5.444914386472304635 ) ) ;
#6187=( BOUNDED_CURVE ( )  B_SPLINE_CURVE ( 2, ( #22182, #1341, #27414, #11323, #25126, #7877, #523, #3613, #5613 ),
 .UNSPECIFIED., .F., .F. ) 
 B_SPLINE_CURVE_WITH_KNOTS ( ( 3, 2, 2, 2, 3 ),
 ( 0.1041666666666664909, 0.1145833333333332732, 0.1250000000000000833, 0.1354166666666668517, 0.1458333333333336757 ),
 .UNSPECIFIED. ) 
 CURVE ( )  GEOMETRIC_REPRESENTATION_ITEM ( )  RATIONAL_B_SPLINE_CURVE ( ( 1.000000000000001332, 0.9238795325112854062, 1.000000000000000000, 0.9238795325112867385, 1.000000000000000000, 0.9238795325112867385, 1.000000000000000000, 0.9238795325112842960, 1.000000000000002442 ) ) 
 REPRESENTATION_ITEM ( '' )  );
#6188=ORIENTED_EDGE ( 'NONE', *, *, #19611, .F. ) ;
#6189=VERTEX_POINT ( 'NONE', #17929 ) ;
#6192=EDGE_CURVE ( 'NONE', #24599, #11583, #5289, .T. ) ;
#6197=DIRECTION ( 'NONE',  ( -0.000000000000000000, -1.000000000000000000, -0.000000000000000000 ) ) ;
#6199=CARTESIAN_POINT ( 'NONE',  ( 195.0000000000000000, 40.15664062608393436, 13.14518615778179544 ) ) ;
#6202=EDGE_LOOP ( 'NONE', ( #23639, #1547, #23288 ) ) ;
#6206=CARTESIAN_POINT ( 'NONE',  ( 116.8548138422182063, 36.03906250108394005, 5.444914386472304635 ) ) ;
#6207=CARTESIAN_POINT ( 'NONE',  ( 78.14518615778179367, 37.03125000108393294, -5.444914386472297529 ) ) ;
#6208=ADVANCED_FACE ( 'NONE', ( #13203 ), #26199, .T. ) ;
#6209=CARTESIAN_POINT ( 'NONE',  ( 189.5550856135277229, 32.76484375108393010, 13.14518615778179722 ) ) ;
#6210=CARTESIAN_POINT ( 'NONE',  ( 52.16024876314180858, 35.99999999999999289, 2.850296047819762091 ) ) ;
#6211=CARTESIAN_POINT ( 'NONE',  ( -13.14518615778179189, 36.63437500108393152, 5.444914386472304635 ) ) ;
#6214=CARTESIAN_POINT ( 'NONE',  ( 192.7020394139928499, 35.99999999999997868, 12.97104423350699420 ) ) ;
#6215=DIRECTION ( 'NONE',  ( 0.000000000000000000, 0.000000000000000000, -1.000000000000000000 ) ) ;
#6216=CARTESIAN_POINT ( 'NONE',  ( 13.14518615778179900, 37.82500000108392868, -5.444914386472297529 ) ) ;
#6230=DIRECTION ( 'NONE',  ( 1.000000000000000000, 0.000000000000000000, -0.000000000000000000 ) ) ;
#6231=CARTESIAN_POINT ( 'NONE',  ( 104.4587341249999639, 84.18750000136560629, -1.442382525525748735E-14 ) ) ;
#6232=CARTESIAN_POINT ( 'NONE',  ( 70.44491438647230552, 37.82500000108392868, 13.14518615778179189 ) ) ;
#6235=VECTOR ( 'NONE', #19825, 1000.000000000000000 ) ;
#6236=CARTESIAN_POINT ( 'NONE',  ( 0.000000000000000000, 52.00000000000000711, 0.000000000000000000 ) ) ;
#6238=CARTESIAN_POINT ( 'NONE',  ( 116.4251840539369454, 40.15664062500000142, -5.622872871577873077 ) ) ;
#6239=EDGE_CURVE ( 'NONE', #26226, #4887, #26493, .T. ) ;
#6240=ORIENTED_EDGE ( 'NONE', *, *, #8435, .T. ) ;
#6243=CARTESIAN_POINT ( 'NONE',  ( 120.7049497278729575, 37.47773437608393010, 9.295050272127047819 ) ) ;
#6244=CARTESIAN_POINT ( 'NONE',  ( 65.00000000000000000, 37.32890625216786873, 13.57481594606304576 ) ) ;
#6246=CARTESIAN_POINT ( 'NONE',  ( 5.622872871577878406, 34.20351562716788862, 13.57481594606304576 ) ) ;
#6248=CARTESIAN_POINT ( 'NONE',  ( 189.5550856135277229, 37.52734375108393294, 13.14518615778179722 ) ) ;
#6250=DIRECTION ( 'NONE',  ( 1.000000000000000000, 0.000000000000000000, -7.228014483236696740E-18 ) ) ;
#6251=CARTESIAN_POINT ( 'NONE',  ( 130.0000000000000000, 39.56132812608393579, -13.14518615778179544 ) ) ;
#6252=DIRECTION ( 'NONE',  ( 0.000000000000000000, 0.000000000000000000, 1.000000000000000000 ) ) ;
#6254=LINE ( 'NONE', #10233, #16039 ) ;
#6255=CARTESIAN_POINT ( 'NONE',  ( 59.37712712842228058, 36.88242187499999858, -13.57481594606318254 ) ) ;
#6257=CARTESIAN_POINT ( 'NONE',  ( 204.5988444088204687, 36.53515624999999289, 9.598844408820456309 ) ) ;
#6258=DIRECTION ( 'NONE',  ( -0.000000000000000000, -1.000000000000000000, -0.000000000000000000 ) ) ;
#6260=CARTESIAN_POINT ( 'NONE',  ( 78.14518615778179367, 40.10703125108393152, 5.444914386472293977 ) ) ;
#6265=CARTESIAN_POINT ( 'NONE',  ( -9.598844408820458085, 38.51953124999999289, -9.598844408820458085 ) ) ;
#6266=FACE_OUTER_BOUND ( 'NONE', #8026, .T. ) ;
#6268=CARTESIAN_POINT ( 'NONE',  ( 104.4587341249999781, 80.25000000136559208, -1.846868145590750299 ) ) ;
#6269=CARTESIAN_POINT ( 'NONE',  ( 65.00000000000000000, -7.395377635281828788, -7.517135062566165128E-15 ) ) ;
#6271=CARTESIAN_POINT ( 'NONE',  ( 214.9999999999999716, 50.00000000000000000, 14.99999999999994316 ) ) ;
#6272=CARTESIAN_POINT ( 'NONE',  ( 74.29505027212704249, 34.10429687608393579, -9.295050272127046043 ) ) ;
#6273=EDGE_LOOP ( 'NONE', ( #14539, #1807, #13451, #20733 ) ) ;
#6274=DIRECTION ( 'NONE',  ( 0.000000000000000000, 0.000000000000000000, -1.000000000000000000 ) ) ;
#6280=CARTESIAN_POINT ( 'NONE',  ( 200.6228728715778686, 37.37851562716787157, 13.57481594606304576 ) ) ;
#6282=FACE_BOUND ( 'NONE', #20105, .T. ) ;
#6283=DIRECTION ( 'NONE',  ( -1.000000000000000000, -0.000000000000000000, -0.000000000000000000 ) ) ;
#6284=CARTESIAN_POINT ( 'NONE',  ( 139.2950502721270425, 39.66054687608393436, -9.295050272127046043 ) ) ;
#6285=CARTESIAN_POINT ( 'NONE',  ( -8.049105076161786076E-16, 39.75976562608394005, -13.14518615778179544 ) ) ;
#6286=CARTESIAN_POINT ( 'NONE',  ( 139.2950502721270425, 33.70742187608393436, 9.295050272127046043 ) ) ;
#6287=CARTESIAN_POINT ( 'NONE',  ( 78.57481594606304043, 37.47773437500001137, -5.622872871577873077 ) ) ;
#6297=CARTESIAN_POINT ( 'NONE',  ( 5.444914386472297529, 38.12265625108393152, -13.14518615778179900 ) ) ;
#6301=( BOUNDED_CURVE ( )  B_SPLINE_CURVE ( 2, ( #10557, #8708, #27966, #8284, #19545 ),
 .UNSPECIFIED., .F., .F. ) 
 B_SPLINE_CURVE_WITH_KNOTS ( ( 3, 2, 3 ),
 ( 0.000000000000000000, 0.02500000000000002220, 0.05000000000000004441 ),
 .UNSPECIFIED. ) 
 CURVE ( )  GEOMETRIC_REPRESENTATION_ITEM ( )  RATIONAL_B_SPLINE_CURVE ( ( 1.000000000000000000, 0.9238795325112867385, 1.000000000000000000, 0.9238795325112866275, 1.000000000000000222 ) ) 
 REPRESENTATION_ITEM ( '' )  );
#6304=CARTESIAN_POINT ( 'NONE',  ( 189.3771271284220745, 36.38632812499999858, 13.57481594606300135 ) ) ;
#6305=CARTESIAN_POINT ( 'NONE',  ( 103.5355339059327093, 84.62500000000000000, -3.535533905932755072 ) ) ;
#6306=CARTESIAN_POINT ( 'NONE',  ( 200.4449143864723055, 39.51171875108392584, -13.14518615778179900 ) ) ;
#6312=ORIENTED_EDGE ( 'NONE', *, *, #1361, .T. ) ;
#6314=CARTESIAN_POINT ( 'NONE',  ( -8.201446187645640151, 50.69246985422426377, -15.00000000000000000 ) ) ;
#6315=AXIS2_PLACEMENT_3D ( 'NONE', #13054, #6661, #12916 ) ;
#6316=CARTESIAN_POINT ( 'NONE',  ( 130.0000000000000000, 34.15390625216787157, 13.57481594606304576 ) ) ;
#6317=CARTESIAN_POINT ( 'NONE',  ( 55.70494972787295751, 40.05742187608393579, 9.295050272127047819 ) ) ;
#6319=CARTESIAN_POINT ( 'NONE',  ( 208.1451861577818079, 34.79882812608394005, -1.609821015232357215E-15 ) ) ;
#6322=ORIENTED_EDGE ( 'NONE', *, *, #23377, .T. ) ;
#6326=CARTESIAN_POINT ( 'NONE',  ( 103.1528011352953342, 81.81250000136559208, 3.152801135295355106 ) ) ;
#6327=CARTESIAN_POINT ( 'NONE',  ( 189.5550856135277229, 37.52734375108393294, 13.14518615778179722 ) ) ;
#6329=CYLINDRICAL_SURFACE ( 'NONE', #5479, 5.000000000000004441 ) ;
#6331=AXIS2_PLACEMENT_3D ( 'NONE', #26109, #11264, #15692 ) ;
#6334=ORIENTED_EDGE ( 'NONE', *, *, #23255, .T. ) ;
#6339=CARTESIAN_POINT ( 'NONE',  ( 120.7049497278729575, 35.29492187608393294, 9.295050272127047819 ) ) ;
#6340=CARTESIAN_POINT ( 'NONE',  ( 65.00000000000000000, 33.21132812608393436, -13.14518615778179544 ) ) ;
#6341=CARTESIAN_POINT ( 'NONE',  ( 181.8548138422182205, 37.57695312608393579, 0.000000000000000000 ) ) ;
#6342=CARTESIAN_POINT ( 'NONE',  ( 195.0000000000000000, 37.22968749999999716, 13.57481594606304576 ) ) ;
#6343=CARTESIAN_POINT ( 'NONE',  ( -5.444914386472299306, 35.93984375108392726, 13.14518615778179722 ) ) ;
#6346=CARTESIAN_POINT ( 'NONE',  ( 219.9999999999999716, 75.00000000000000000, 9.999999999999946709 ) ) ;
#6349=CARTESIAN_POINT ( 'NONE',  ( -5.444914386472299306, 39.90859375108393436, 13.14518615778179722 ) ) ;
#6353=CARTESIAN_POINT ( 'NONE',  ( 63.98586917393215145, 51.45790058219657936, 15.00000000000065548 ) ) ;
#6356=CYLINDRICAL_SURFACE ( 'NONE', #22603, 5.000000000000004441 ) ;
#6358=CARTESIAN_POINT ( 'NONE',  ( 124.3771271284222308, 40.85117187499999147, -13.57481594606315412 ) ) ;
#6360=CARTESIAN_POINT ( 'NONE',  ( 51.42518405393695957, 37.97382812716787726, 5.622872871577880183 ) ) ;
#6361=AXIS2_PLACEMENT_3D ( 'NONE', #12998, #2211, #208 ) ;
#6362=ADVANCED_FACE ( 'NONE', ( #10066 ), #18778, .T. ) ;
#6365=CARTESIAN_POINT ( 'NONE',  ( 95.54126587499995082, 79.75000000136560629, 1.846868145590724986 ) ) ;
#6366=CARTESIAN_POINT ( 'NONE',  ( 78.14518615778179367, 37.18007812608393436, -1.609821015232357215E-15 ) ) ;
#6368=CARTESIAN_POINT ( 'NONE',  ( -5.444914386472297529, 39.61093750108393152, -13.14518615778179722 ) ) ;
#6372=CARTESIAN_POINT ( 'NONE',  ( 116.4251840539369596, 40.20624999999999005, 0.000000000000000000 ) ) ;
#6373=ORIENTED_EDGE ( 'NONE', *, *, #4442, .F. ) ;
#6374=CARTESIAN_POINT ( 'NONE',  ( -20.00000000000000000, 50.00000000000000000, 10.00000000000000178 ) ) ;
#6375=DIRECTION ( 'NONE',  ( 0.000000000000000000, 0.000000000000000000, 1.000000000000000000 ) ) ;
#6376=CARTESIAN_POINT ( 'NONE',  ( 99.99999999999995737, 79.68750000136559208, 4.458734124999988779 ) ) ;
#6377=CARTESIAN_POINT ( 'NONE',  ( 116.8548138422182063, 35.84062500108394289, 5.444914386472304635 ) ) ;
#6378=CARTESIAN_POINT ( 'NONE',  ( 59.37712712842213136, 36.18789062716787441, -13.57481594606304753 ) ) ;
#6382=CARTESIAN_POINT ( 'NONE',  ( 9.598844408820456309, 36.83281250216787583, -9.598844408820458085 ) ) ;
#6387=CARTESIAN_POINT ( 'NONE',  ( 185.7049497278729575, 38.27148437608393294, 9.295050272127047819 ) ) ;
#6389=CARTESIAN_POINT ( 'NONE',  ( 70.62287287157793969, 39.16445312500000142, -13.57481594606299247 ) ) ;
#6391=CARTESIAN_POINT ( 'NONE',  ( 143.1451861577818079, 36.18789062608393436, -1.609821015232357215E-15 ) ) ;
#6392=CARTESIAN_POINT ( 'NONE',  ( 195.0000000000000000, 37.72578125216787726, -13.57481594606304576 ) ) ;
#6394=CARTESIAN_POINT ( 'NONE',  ( 133.0393970508025916, 53.88964894337313183, 14.99999999999997158 ) ) ;
#6398=CARTESIAN_POINT ( 'NONE',  ( 208.5748159460630120, 37.47773437500001137, -5.622872871577873077 ) ) ;
#6401=CARTESIAN_POINT ( 'NONE',  ( 51.85481384221820633, 37.37851562608393863, 0.000000000000000000 ) ) ;
#6407=CARTESIAN_POINT ( 'NONE',  ( -8.312177448680279460E-16, 37.62656249999999858, -13.57481594606304576 ) ) ;
#6410=CARTESIAN_POINT ( 'NONE',  ( 95.54126587499996504, 80.68750000136559208, -1.387778780781445676E-14 ) ) ;
#6414=CARTESIAN_POINT ( 'NONE',  ( 78.14518615778179367, 34.05468750108394005, -5.444914386472297529 ) ) ;
#6416=VERTEX_POINT ( 'NONE', #7665 ) ;
#6417=CARTESIAN_POINT ( 'NONE',  ( 136.1165602397167902, 54.66944451632673463, -15.00000000000000000 ) ) ;
#6419=ORIENTED_EDGE ( 'NONE', *, *, #16651, .T. ) ;
#6422=CARTESIAN_POINT ( 'NONE',  ( 189.3771271284221314, 36.98164062716787015, -13.57481594606304753 ) ) ;
#6424=PLANE ( 'NONE',  #17575 ) ;
#6425=LINE ( 'NONE', #23814, #3087 ) ;
#6426=CARTESIAN_POINT ( 'NONE',  ( 135.4449143864723339, 37.32890625108393579, -13.14518615778179722 ) ) ;
#6427=CARTESIAN_POINT ( 'NONE',  ( 2.414731522848535132E-15, 36.98164062608393721, 13.14518615778179544 ) ) ;
#6428=CARTESIAN_POINT ( 'NONE',  ( 116.8548138422182063, 33.45937500108392726, 5.444914386472304635 ) ) ;
#6429=CARTESIAN_POINT ( 'NONE',  ( 74.59884440882045453, 33.55859375000000000, -9.598844408820458085 ) ) ;
#6432=CYLINDRICAL_SURFACE ( 'NONE', #7115, 13.57481594606304398 ) ;
#6437=CARTESIAN_POINT ( 'NONE',  ( 99.99999999999995737, 80.93750000136559208, 4.458734124999988779 ) ) ;
#6439=CARTESIAN_POINT ( 'NONE',  ( -5.444914386472299306, 40.10703125108393152, 13.14518615778179722 ) ) ;
#6445=CARTESIAN_POINT ( 'NONE',  ( 204.2950502721270425, 40.05742187608392868, 9.295050272127046043 ) ) ;
#6449=CARTESIAN_POINT ( 'NONE',  ( 130.0000000000000000, 39.61093749999999147, 13.57481594606304576 ) ) ;
#6454=CARTESIAN_POINT ( 'NONE',  ( 135.4449143864723055, 39.51171875108392584, -13.14518615778179900 ) ) ;
#6458=CARTESIAN_POINT ( 'NONE',  ( 204.2950502721270425, 33.90585937608393863, 9.295050272127046043 ) ) ;
#6460=ORIENTED_EDGE ( 'NONE', *, *, #23415, .T. ) ;
#6465=CARTESIAN_POINT ( 'NONE',  ( 70.44491438647229131, 39.21406250108392300, 13.14518615778179189 ) ) ;
#6466=CARTESIAN_POINT ( 'NONE',  ( 95.54126587499996504, 79.43750000136559208, -1.387778780781445676E-14 ) ) ;
#6467=CARTESIAN_POINT ( 'NONE',  ( 189.5550856135277229, 39.90859375108392726, 13.14518615778179722 ) ) ;
#6470=CARTESIAN_POINT ( 'NONE',  ( 77.07727640983618755, 35.99999999999999289, -6.197985357348143154 ) ) ;
#6473=ORIENTED_EDGE ( 'NONE', *, *, #18158, .T. ) ;
#6477=CARTESIAN_POINT ( 'NONE',  ( 135.4449143864723055, 34.94765625108394147, -13.14518615778179900 ) ) ;
#6478=CARTESIAN_POINT ( 'NONE',  ( 74.29505027212704249, 32.31835937608393294, -9.295050272127046043 ) ) ;
#6479=CIRCLE ( 'NONE', #9685, 13.57481594606304398 ) ;
#6480=CARTESIAN_POINT ( 'NONE',  ( 208.1451861577817795, 37.22968750108393721, -5.444914386472297529 ) ) ;
#6482=CARTESIAN_POINT ( 'NONE',  ( 3.755638265659908104, 31.58960998161716560, -13.14518615778179900 ) ) ;
#6483=CARTESIAN_POINT ( 'NONE',  ( 131.0141308260786559, 51.45790058219927232, -14.99999999999932676 ) ) ;
#6487=CARTESIAN_POINT ( 'NONE',  ( -8.049105076161786076E-16, 34.79882812608393294, -13.14518615778179544 ) ) ;
#6488=CARTESIAN_POINT ( 'NONE',  ( -15.00000000000000000, 55.00000000000000000, 10.00000000000000000 ) ) ;
#6496=CARTESIAN_POINT ( 'NONE',  ( 120.8198241863519939, 55.00000000000001421, 14.99999999999996625 ) ) ;
#6499=CARTESIAN_POINT ( 'NONE',  ( 98.15313185440925281, 82.87500000136560629, 4.458734124999987891 ) ) ;
#6500=CARTESIAN_POINT ( 'NONE',  ( 78.14518615778179367, 36.43593750108392726, -5.444914386472297529 ) ) ;
#6506=CARTESIAN_POINT ( 'NONE',  ( 0.000000000000000000, 36.00000000000000000, 0.000000000000000000 ) ) ;
#6507=CARTESIAN_POINT ( 'NONE',  ( 116.4251840539369596, 36.23749999999999005, 0.000000000000000000 ) ) ;
#6513=CARTESIAN_POINT ( 'NONE',  ( 130.0000000000000000, 37.57695312608392868, 13.14518615778179544 ) ) ;
#6514=CARTESIAN_POINT ( 'NONE',  ( 59.37712712842213136, 34.10429687716786873, 13.57481594606304753 ) ) ;
#6515=CARTESIAN_POINT ( 'NONE',  ( 103.5355339059327093, 83.62500000000000000, -3.535533905932755072 ) ) ;
#6516=CARTESIAN_POINT ( 'NONE',  ( -9.598844408820458085, 31.47500000216787441, -9.598844408820458085 ) ) ;
#6518=EDGE_CURVE ( 'NONE', #23304, #19109, #12510, .T. ) ;
#6520=CARTESIAN_POINT ( 'NONE',  ( 185.7049497278729575, 37.27929687608393294, -9.295050272127046043 ) ) ;
#6521=DIRECTION ( 'NONE',  ( -1.000000000000000000, -3.469446951953617147E-16, 2.385244779468109755E-16 ) ) ;
#6524=CARTESIAN_POINT ( 'NONE',  ( 195.0000000000000000, 36.83281249999999574, -13.57481594606304576 ) ) ;
#6526=CARTESIAN_POINT ( 'NONE',  ( 51.42518405393695957, 37.03124999999999289, 0.000000000000000000 ) ) ;
#6529=CARTESIAN_POINT ( 'NONE',  ( 204.5988444088204687, 35.74140624999999716, 9.598844408820456309 ) ) ;
#6530=EDGE_CURVE ( 'NONE', #23121, #26178, #21849, .T. ) ;
#6533=CARTESIAN_POINT ( 'NONE',  ( 59.55508561352770158, 36.43593750108392726, -13.14518615778179900 ) ) ;
#6535=DIRECTION ( 'NONE',  ( 0.000000000000000000, -1.000000000000000000, 0.000000000000000000 ) ) ;
#6538=CARTESIAN_POINT ( 'NONE',  ( -8.312177448680279460E-16, 36.83281249999999574, -13.57481594606304576 ) ) ;
#6539=DIRECTION ( 'NONE',  ( -1.000000000000000000, 0.000000000000000000, 2.385244779468110248E-16 ) ) ;
#6540=VERTEX_POINT ( 'NONE', #28169 ) ;
#6541=CARTESIAN_POINT ( 'NONE',  ( 94.99999999999995737, 83.06250000000001421, 2.071067811865466624 ) ) ;
#6543=CARTESIAN_POINT ( 'NONE',  ( 65.37454041347797329, 36.00000000000002842, -13.51869779562200691 ) ) ;
#6544=ORIENTED_EDGE ( 'NONE', *, *, #14200, .T. ) ;
#6547=CARTESIAN_POINT ( 'NONE',  ( 65.00000000000000000, 34.60039062608393579, 13.14518615778179544 ) ) ;
#6549=( BOUNDED_CURVE ( )  B_SPLINE_CURVE ( 2, ( #7538, #27367, #20667, #26947, #18525, #12080, #18380, #1151, #22948 ),
 .UNSPECIFIED., .F., .T. ) 
 B_SPLINE_CURVE_WITH_KNOTS ( ( 3, 2, 2, 2, 3 ),
 ( 0.2291666666666665741, 0.2395833333333332316, 0.2499999999999998335, 0.2604166666666665186, 0.2708333333333330928 ),
 .UNSPECIFIED. ) 
 CURVE ( )  GEOMETRIC_REPRESENTATION_ITEM ( )  RATIONAL_B_SPLINE_CURVE ( ( 1.000000000000000666, 0.9238795325112861834, 1.000000000000000000, 0.9238795325112867385, 1.000000000000000000, 0.9238795325112867385, 1.000000000000000000, 0.9238795325112884038, 0.9999999999999983347 ) ) 
 REPRESENTATION_ITEM ( '' )  );
#6554=CARTESIAN_POINT ( 'NONE',  ( 181.4251840539369596, 37.08085937716786873, -5.622872871577873077 ) ) ;
#6557=CARTESIAN_POINT ( 'NONE',  ( 200.6228728715778971, 39.75976562716787299, 13.57481594606306174 ) ) ;
#6558=ORIENTED_EDGE ( 'NONE', *, *, #14372, .F. ) ;
#6559=CARTESIAN_POINT ( 'NONE',  ( -8.049105076161786076E-16, 38.17226562608394147, -13.14518615778179544 ) ) ;
#6560=CARTESIAN_POINT ( 'NONE',  ( 143.1451861577818079, 36.18789062608393436, -1.609821015232357215E-15 ) ) ;
#6561=CARTESIAN_POINT ( 'NONE',  ( 70.62287287157786864, 34.40195312499999858, -13.57481594606304753 ) ) ;
#6564=CARTESIAN_POINT ( 'NONE',  ( 200.3649479647158671, 36.00000000000000000, 12.09311862596019260 ) ) ;
#6569=CARTESIAN_POINT ( 'NONE',  ( 95.54126587499996504, 79.75000000136560629, 1.846868145590724986 ) ) ;
#6571=CARTESIAN_POINT ( 'NONE',  ( -5.444914386472297529, 36.63437500108393152, -13.14518615778179900 ) ) ;
#6573=ORIENTED_EDGE ( 'NONE', *, *, #2740, .T. ) ;
#6578=CARTESIAN_POINT ( 'NONE',  ( 185.7049497278729575, 37.47773437608393010, 9.295050272127047819 ) ) ;
#6579=ORIENTED_EDGE ( 'NONE', *, *, #9687, .T. ) ;
#6585=VECTOR ( 'NONE', #10404, 1000.000000000000000 ) ;
#6586=CARTESIAN_POINT ( 'NONE',  ( 120.4011555911795455, 37.72578124999999005, -9.598844408820458085 ) ) ;
#6587=CARTESIAN_POINT ( 'NONE',  ( 97.92893218813446765, 81.31250000273119838, 4.999999999999962697 ) ) ;
#6588=CARTESIAN_POINT ( 'NONE',  ( 130.0000000000000000, 40.35507812608393152, -13.14518615778179544 ) ) ;
#6589=CARTESIAN_POINT ( 'NONE',  ( -13.14518615778179722, 39.90859375108393436, -5.444914386472297529 ) ) ;
#6590=( BOUNDED_CURVE ( )  B_SPLINE_CURVE ( 2, ( #22612, #18033, #3082, #17896, #26746, #7188, #18472, #15886, #24602 ),
 .UNSPECIFIED., .F., .F. ) 
 B_SPLINE_CURVE_WITH_KNOTS ( ( 3, 2, 2, 2, 3 ),
 ( 0.1875000000000001388, 0.1979166666666667407, 0.2083333333333333703, 0.2187499999999999722, 0.2291666666666665741 ),
 .UNSPECIFIED. ) 
 CURVE ( )  GEOMETRIC_REPRESENTATION_ITEM ( )  RATIONAL_B_SPLINE_CURVE ( ( 0.9999999999999990008, 0.9238795325112877377, 1.000000000000000000, 0.9238795325112867385, 1.000000000000000000, 0.9238795325112867385, 1.000000000000000000, 0.9238795325112872936, 0.9999999999999994449 ) ) 
 REPRESENTATION_ITEM ( '' )  );
#6592=CARTESIAN_POINT ( 'NONE',  ( 59.55508561352770158, 39.31328125108394289, 13.14518615778179722 ) ) ;
#6593=DIRECTION ( 'NONE',  ( 1.000000000000000000, 0.000000000000000000, 0.000000000000000000 ) ) ;
#6594=CARTESIAN_POINT ( 'NONE',  ( 185.7049497278729575, 33.50898437608393010, -9.295050272127046043 ) ) ;
#6595=ORIENTED_EDGE ( 'NONE', *, *, #27563, .T. ) ;
#6597=ORIENTED_EDGE ( 'NONE', *, *, #22907, .F. ) ;
#6600=CARTESIAN_POINT ( 'NONE',  ( 74.29505027212704249, 39.46210937608393010, -9.295050272127046043 ) ) ;
#6601=CARTESIAN_POINT ( 'NONE',  ( 98.15313185440923860, 81.25000000136559208, -4.458734125000016313 ) ) ;
#6602=CARTESIAN_POINT ( 'NONE',  ( 181.8548138422182205, 39.80937500108393579, 5.444914386472304635 ) ) ;
#6604=CARTESIAN_POINT ( 'NONE',  ( 188.5491206573239253, 50.00000000106884102, 11.97362904074905998 ) ) ;
#6605=DIRECTION ( 'NONE',  ( 0.000000000000000000, -1.000000000000000000, 0.000000000000000000 ) ) ;
#6612=AXIS2_PLACEMENT_3D ( 'NONE', #6236, #16647, #7818 ) ;
#6614=CARTESIAN_POINT ( 'NONE',  ( 120.7049497278729575, 37.67617187608393436, 9.295050272127047819 ) ) ;
#6615=CARTESIAN_POINT ( 'NONE',  ( 59.55508561352770158, 32.46718750108393436, -13.14518615778179900 ) ) ;
#6616=CARTESIAN_POINT ( 'NONE',  ( 189.5550856135277229, 37.42812500108394147, -13.14518615778179900 ) ) ;
#6617=EDGE_LOOP ( 'NONE', ( #27946, #26541, #2874 ) ) ;
#6618=CARTESIAN_POINT ( 'NONE',  ( 65.70502410996888898, 35.99999999999997158, 13.13343125082108287 ) ) ;
#6619=CARTESIAN_POINT ( 'NONE',  ( 132.1699565831061420, 49.99999999883939950, -13.43548448457870670 ) ) ;
#6620=CARTESIAN_POINT ( 'NONE',  ( -8.312177448680279460E-16, 39.21406249999999716, -13.57481594606304576 ) ) ;
#6621=DIRECTION ( 'NONE',  ( 0.000000000000000000, 1.000000000000000000, 0.000000000000000000 ) ) ;
#6624=CARTESIAN_POINT ( 'NONE',  ( 13.14518615778179544, 35.39414062608393152, -1.609821015232357215E-15 ) ) ;
#6634=FACE_OUTER_BOUND ( 'NONE', #21300, .T. ) ;
#6637=DIRECTION ( 'NONE',  ( -0.000000000000000000, 1.000000000000000000, -0.000000000000000000 ) ) ;
#6638=CARTESIAN_POINT ( 'NONE',  ( 74.29505027212704249, 33.90585937608393863, 9.295050272127046043 ) ) ;
#6640=CARTESIAN_POINT ( 'NONE',  ( -8.049105076161786076E-16, 36.38632812608393152, -13.14518615778179544 ) ) ;
#6642=CARTESIAN_POINT ( 'NONE',  ( 120.4011555911795455, 36.33671874999999574, 9.598844408820459861 ) ) ;
#6643=CARTESIAN_POINT ( 'NONE',  ( 116.4251840539369596, 38.61874999999999147, 0.000000000000000000 ) ) ;
#6648=CARTESIAN_POINT ( 'NONE',  ( 135.4449143864723055, 37.13046875108393152, -13.14518615778179900 ) ) ;
#6649=CARTESIAN_POINT ( 'NONE',  ( 51.42518405393695957, 34.74921875216787726, 0.000000000000000000 ) ) ;
#6652=CARTESIAN_POINT ( 'NONE',  ( -5.622872871577873077, 32.21914062716787441, -13.57481594606304753 ) ) ;
#6655=CARTESIAN_POINT ( 'NONE',  ( 189.5550856135277229, 35.64218750108392442, -13.14518615778179900 ) ) ;
#6658=LINE ( 'NONE', #22494, #11409 ) ;
#6659=ORIENTED_EDGE ( 'NONE', *, *, #14238, .F. ) ;
#6660=EDGE_CURVE ( 'NONE', #17678, #2842, #2112, .T. ) ;
#6661=DIRECTION ( 'NONE',  ( -0.000000000000000000, 1.000000000000000000, -0.000000000000000000 ) ) ;
#6664=DIRECTION ( 'NONE',  ( 0.000000000000000000, 0.000000000000000000, 1.000000000000000000 ) ) ;
#6667=CARTESIAN_POINT ( 'NONE',  ( 189.3771271284221314, 34.79882812499998579, 13.57481594606304753 ) ) ;
#6669=CARTESIAN_POINT ( 'NONE',  ( 130.0000000000000000, 36.83281249999999574, -13.57481594606304576 ) ) ;
#6670=CARTESIAN_POINT ( 'NONE',  ( 51.85481384221820633, 34.20351562608393436, 0.000000000000000000 ) ) ;
#6674=CARTESIAN_POINT ( 'NONE',  ( -13.57481594606304753, 35.39414062499999147, -5.622872871577873077 ) ) ;
#6675=CARTESIAN_POINT ( 'NONE',  ( 124.5550856135277087, 36.63437500108393152, -13.14518615778179900 ) ) ;
#6676=ORIENTED_EDGE ( 'NONE', *, *, #5320, .T. ) ;
#6678=CARTESIAN_POINT ( 'NONE',  ( 102.0710678118654329, 84.68750000000001421, -5.000000000000018652 ) ) ;
#6679=CARTESIAN_POINT ( 'NONE',  ( 102.0710678118654329, 80.81250000273119838, -5.000000000000018652 ) ) ;
#6681=CARTESIAN_POINT ( 'NONE',  ( 54.45404289489643190, 35.99999999999996447, -8.172591786207583198 ) ) ;
#6684=CARTESIAN_POINT ( 'NONE',  ( 78.14518615778179367, 34.84843750108393579, -5.444914386472297529 ) ) ;
#6688=ORIENTED_EDGE ( 'NONE', *, *, #16115, .F. ) ;
#6690=CARTESIAN_POINT ( 'NONE',  ( 208.5748159460630688, 34.35234375216787583, -1.662435489736055892E-15 ) ) ;
#6691=EDGE_CURVE ( 'NONE', #11663, #1369, #23005, .T. ) ;
#6693=CARTESIAN_POINT ( 'NONE',  ( -9.598844408820458085, 40.90078124999999432, -9.598844408820458085 ) ) ;
#6694=CARTESIAN_POINT ( 'NONE',  ( 195.0000000000000000, 40.10703125216787157, -13.57481594606304576 ) ) ;
#6695=ORIENTED_EDGE ( 'NONE', *, *, #26955, .F. ) ;
#6696=CARTESIAN_POINT ( 'NONE',  ( -9.295050272127046043, 39.06523437608392868, -9.295050272127046043 ) ) ;
#6698=CARTESIAN_POINT ( 'NONE',  ( 120.7049497278729575, 35.09648437608392868, 9.295050272127047819 ) ) ;
#6699=CARTESIAN_POINT ( 'NONE',  ( 59.37712712842213136, 34.50117187499999005, -13.57481594606304753 ) ) ;
#6700=CARTESIAN_POINT ( 'NONE',  ( 13.57481594606304576, 38.32109375216786873, -1.662435489736055892E-15 ) ) ;
#6703=CARTESIAN_POINT ( 'NONE',  ( 189.3771271284221882, 37.18007812499999432, 13.57481594606311504 ) ) ;
#6707=VECTOR ( 'NONE', #24443, 1000.000000000000000 ) ;
#6708=CIRCLE ( 'NONE', #26296, 3.000000000000004441 ) ;
#6709=CARTESIAN_POINT ( 'NONE',  ( 130.0000000000000000, 37.62656249999999858, -13.57481594606304576 ) ) ;
#6711=CARTESIAN_POINT ( 'NONE',  ( -13.14518615778179900, 35.14609375108393152, -5.444914386472297529 ) ) ;
#6716=( BOUNDED_CURVE ( )  B_SPLINE_CURVE ( 2, ( #17765, #6922, #8650, #17338, #24318, #13034, #4804, #26034, #15326 ),
 .UNSPECIFIED., .F., .T. ) 
 B_SPLINE_CURVE_WITH_KNOTS ( ( 3, 2, 2, 2, 3 ),
 ( 0.6500000000000005773, 0.6750000000000005995, 0.7000000000000006217, 0.7250000000000006439, 0.7500000000000006661 ),
 .UNSPECIFIED. ) 
 CURVE ( )  GEOMETRIC_REPRESENTATION_ITEM ( )  RATIONAL_B_SPLINE_CURVE ( ( 0.9999999999999983347, 0.9238795325112884038, 1.000000000000000000, 0.9238795325112867385, 1.000000000000000000, 0.9238795325112867385, 1.000000000000000000, 0.9238795325112847401, 1.000000000000001998 ) ) 
 REPRESENTATION_ITEM ( '' )  );
#6719=CARTESIAN_POINT ( 'NONE',  ( 181.8548138422182205, 40.55351562608393579, 0.000000000000000000 ) ) ;
#6721=CARTESIAN_POINT ( 'NONE',  ( 51.90409344636400846, 35.99999999999999289, 1.137167824541468031 ) ) ;
#6722=CARTESIAN_POINT ( 'NONE',  ( 99.99999999999995737, 85.00000000000000000, 4.999999999999990230 ) ) ;
#6724=VERTEX_POINT ( 'NONE', #25022 ) ;
#6730=CARTESIAN_POINT ( 'NONE',  ( 135.6228728715778971, 32.61601562716786873, 13.57481594606304576 ) ) ;
#6731=CARTESIAN_POINT ( 'NONE',  ( 195.0000000000000000, 38.91640625216786731, 13.57481594606304576 ) ) ;
#6733=CARTESIAN_POINT ( 'NONE',  ( 78.14518615778179367, 37.18007812608393436, -1.609821015232357215E-15 ) ) ;
#6735=EDGE_CURVE ( 'NONE', #19811, #444, #713, .T. ) ;
#6736=CARTESIAN_POINT ( 'NONE',  ( 189.5550856135277229, 35.84062500108394289, -13.14518615778179900 ) ) ;
#6737=ORIENTED_EDGE ( 'NONE', *, *, #9118, .T. ) ;
#6738=ORIENTED_EDGE ( 'NONE', *, *, #20293, .T. ) ;
#6743=CARTESIAN_POINT ( 'NONE',  ( 95.54126587499996504, 80.43750000136559208, -1.387778780781445676E-14 ) ) ;
#6744=CARTESIAN_POINT ( 'NONE',  ( 208.1451861577818079, 40.20625000108393010, -5.444914386472297529 ) ) ;
#6748=CARTESIAN_POINT ( 'NONE',  ( 78.57481594606305464, 39.85898437499999858, -5.622872871577873966 ) ) ;
#6755=AXIS2_PLACEMENT_3D ( 'NONE', #4684, #7083, #7367 ) ;
#6756=ORIENTED_EDGE ( 'NONE', *, *, #1361, .F. ) ;
#6757=CARTESIAN_POINT ( 'NONE',  ( 143.1451861577818079, 37.22968750108393721, -5.444914386472297529 ) ) ;
#6758=CARTESIAN_POINT ( 'NONE',  ( 51.85481384221819923, 33.36015625108393579, -5.444914386472297529 ) ) ;
#6759=CARTESIAN_POINT ( 'NONE',  ( 189.5550856135277229, 38.22187500108393010, -13.14518615778179900 ) ) ;
#6762=CARTESIAN_POINT ( 'NONE',  ( 2.493653234604083739E-15, 37.32890625216786873, 13.57481594606304576 ) ) ;
#6763=CARTESIAN_POINT ( 'NONE',  ( 13.14518615778179900, 33.85625000108393579, -5.444914386472297529 ) ) ;
#6764=CARTESIAN_POINT ( 'NONE',  ( 137.6362410679823540, 54.91786508990713855, -15.00000000000000355 ) ) ;
#6765=CARTESIAN_POINT ( 'NONE',  ( 9.598844408820456309, 39.11484374999999858, -9.598844408820458085 ) ) ;
#6766=CARTESIAN_POINT ( 'NONE',  ( 116.4251840539369596, 39.51171875216787299, 0.000000000000000000 ) ) ;
#6770=ORIENTED_EDGE ( 'NONE', *, *, #4109, .F. ) ;
#6775=CARTESIAN_POINT ( 'NONE',  ( 131.5054921815522277, 53.60078691996476863, 14.99999999999996447 ) ) ;
#6778=FACE_OUTER_BOUND ( 'NONE', #8601, .T. ) ;
#6779=CARTESIAN_POINT ( 'NONE',  ( 104.4587341249999639, 80.18750000136559208, -1.442382525525748735E-14 ) ) ;
#6780=CARTESIAN_POINT ( 'NONE',  ( 65.00000000000000000, 34.20351562608394147, -13.14518615778179544 ) ) ;
#6782=CARTESIAN_POINT ( 'NONE',  ( 9.295050272127047819, 37.67617187608393436, 9.295050272127046043 ) ) ;
#6785=CARTESIAN_POINT ( 'NONE',  ( 135.6228728715779823, 40.75195312499999289, -13.57481594606294095 ) ) ;
#6786=CARTESIAN_POINT ( 'NONE',  ( 143.5748159460630404, 38.27148437500000711, -5.622872871577873077 ) ) ;
#6792=CARTESIAN_POINT ( 'NONE',  ( 130.0000000000000000, 36.78320312608393294, 13.14518615778179544 ) ) ;
#6793=CARTESIAN_POINT ( 'NONE',  ( 65.00000000000000000, 33.75703125216787726, -13.57481594606304576 ) ) ;
#6795=CARTESIAN_POINT ( 'NONE',  ( 2.493653234604083739E-15, 31.77265625216787370, 13.57481594606304576 ) ) ;
#6796=AXIS2_PLACEMENT_3D ( 'NONE', #10354, #14224, #14500 ) ;
#6799=CARTESIAN_POINT ( 'NONE',  ( 204.2950502721270425, 34.69960937608393436, -9.295050272127046043 ) ) ;
#6800=CYLINDRICAL_SURFACE ( 'NONE', #9274, 5.000000000000000888 ) ;
#6803=CARTESIAN_POINT ( 'NONE',  ( 195.0000000000000000, 40.40468749999999432, 13.57481594606304576 ) ) ;
#6804=ORIENTED_EDGE ( 'NONE', *, *, #24079, .F. ) ;
#6805=DIRECTION ( 'NONE',  ( 0.000000000000000000, -1.000000000000000000, 0.000000000000000000 ) ) ;
#6806=CARTESIAN_POINT ( 'NONE',  ( 135.3173515774758187, 54.47013368152368429, 14.99999999999996092 ) ) ;
#6811=CARTESIAN_POINT ( 'NONE',  ( 181.4251840539369596, 35.44374999999999432, 0.000000000000000000 ) ) ;
#6814=CARTESIAN_POINT ( 'NONE',  ( 78.14518615778179367, 36.98164062608393010, -1.609821015232357215E-15 ) ) ;
#6819=CARTESIAN_POINT ( 'NONE',  ( -13.57481594606304576, 36.28710937499999289, 5.622872871577880183 ) ) ;
#6820=CARTESIAN_POINT ( 'NONE',  ( 130.0000000000000000, 36.18789062608393436, 13.14518615778179544 ) ) ;
#6822=CARTESIAN_POINT ( 'NONE',  ( 104.9999999999999574, 84.43750000000002842, 2.071067811865462627 ) ) ;
#6824=EDGE_CURVE ( 'NONE', #12157, #8417, #18926, .T. ) ;
#6825=CARTESIAN_POINT ( 'NONE',  ( 103.5355339059327093, 82.50000000273119838, 3.535533905932726206 ) ) ;
#6829=CARTESIAN_POINT ( 'NONE',  ( 55.40115559117954547, 40.90078124999999432, -9.598844408820458085 ) ) ;
#6830=ORIENTED_EDGE ( 'NONE', *, *, #19411, .F. ) ;
#6836=CARTESIAN_POINT ( 'NONE',  ( 204.5988444088204403, 33.65781250216787157, -9.598844408820458085 ) ) ;
#6838=DIRECTION ( 'NONE',  ( 0.000000000000000000, 1.000000000000000000, 0.000000000000000000 ) ) ;
#6839=CARTESIAN_POINT ( 'NONE',  ( 120.7049497278729575, 37.67617187608393436, 9.295050272127047819 ) ) ;
#6840=CARTESIAN_POINT ( 'NONE',  ( -8.049105076161786076E-16, 34.99726562608393721, -13.14518615778179544 ) ) ;
#6842=CARTESIAN_POINT ( 'NONE',  ( 116.8548138422182205, 34.99726562608393721, 0.000000000000000000 ) ) ;
#6843=CARTESIAN_POINT ( 'NONE',  ( 51.42518405393695957, 33.90585937500000568, 5.622872871577880183 ) ) ;
#6844=CARTESIAN_POINT ( 'NONE',  ( 130.0000000000000000, -7.395377635281828788, -1.503427012513233026E-14 ) ) ;
#6846=CARTESIAN_POINT ( 'NONE',  ( 208.4064236467344813, 36.00000000000002132, 1.227293221035586912 ) ) ;
#6850=CARTESIAN_POINT ( 'NONE',  ( 74.18017581364799184, 55.00000000000000000, 9.999999999999978684 ) ) ;
#6851=FACE_OUTER_BOUND ( 'NONE', #10998, .T. ) ;
#6853=CARTESIAN_POINT ( 'NONE',  ( -5.444914386472299306, 36.93203125108394147, 13.14518615778179722 ) ) ;
#6855=ORIENTED_EDGE ( 'NONE', *, *, #22226, .F. ) ;
#6858=EDGE_CURVE ( 'NONE', #19690, #3877, #14999, .T. ) ;
#6861=ADVANCED_FACE ( 'NONE', ( #12435 ), #10163, .T. ) ;
#6862=CARTESIAN_POINT ( 'NONE',  ( 189.5550856135277229, 38.32109375108394289, 13.14518615778179722 ) ) ;
#6863=ORIENTED_EDGE ( 'NONE', *, *, #15915, .T. ) ;
#6873=EDGE_CURVE ( 'NONE', #4508, #23121, #14862, .T. ) ;
#6874=CARTESIAN_POINT ( 'NONE',  ( 130.0000000000000000, 32.56640625216787299, 13.57481594606304576 ) ) ;
#6877=CARTESIAN_POINT ( 'NONE',  ( 59.55508561352770158, 37.42812500108394147, -13.14518615778179900 ) ) ;
#6878=CARTESIAN_POINT ( 'NONE',  ( 71.90237857378353681, 51.13402819306926972, -15.00000000000000178 ) ) ;
#6879=CARTESIAN_POINT ( 'NONE',  ( 181.4251840539369596, 40.95039062499999005, -5.622872871577873077 ) ) ;
#6880=SPHERICAL_SURFACE ( 'NONE', #10280, 5.000000000000000000 ) ;
#6886=CARTESIAN_POINT ( 'NONE',  ( 78.14518615778180788, 40.10703125108393152, 5.444914386472293977 ) ) ;
#6888=CARTESIAN_POINT ( 'NONE',  ( 104.4587341249999639, 81.93750000136559208, -1.442382525525748735E-14 ) ) ;
#6889=CARTESIAN_POINT ( 'NONE',  ( 200.4449143864723055, 40.00781250108393294, 13.14518615778179189 ) ) ;
#6892=CARTESIAN_POINT ( 'NONE',  ( 200.4449143864723055, 38.91640625108393436, -13.14518615778179722 ) ) ;
#6898=CARTESIAN_POINT ( 'NONE',  ( 116.8548138422182205, 34.40195312608393152, 0.000000000000000000 ) ) ;
#6899=CARTESIAN_POINT ( 'NONE',  ( 55.70494972787295751, 35.09648437608392868, 9.295050272127047819 ) ) ;
#6901=CARTESIAN_POINT ( 'NONE',  ( 195.0000000000000000, 37.77539062608393294, 13.14518615778179544 ) ) ;
#6902=ORIENTED_EDGE ( 'NONE', *, *, #15277, .T. ) ;
#6904=CARTESIAN_POINT ( 'NONE',  ( 181.8548138422182205, 40.75195312608393294, 0.000000000000000000 ) ) ;
#6905=DIRECTION ( 'NONE',  ( 1.000000000000000000, 0.000000000000000000, 0.000000000000000000 ) ) ;
#6910=ORIENTED_EDGE ( 'NONE', *, *, #20818, .F. ) ;
#6918=CARTESIAN_POINT ( 'NONE',  ( 98.15313185440925281, 81.50000000136560629, -4.458734125000016313 ) ) ;
#6919=CARTESIAN_POINT ( 'NONE',  ( 70.44491438647230552, 36.53515625108393294, -13.14518615778179900 ) ) ;
#6921=CARTESIAN_POINT ( 'NONE',  ( 9.295050272127047819, 38.46992187608393010, 9.295050272127046043 ) ) ;
#6922=CARTESIAN_POINT ( 'NONE',  ( 102.0710678118654755, 80.81250000273119838, -4.999999999999983125 ) ) ;
#6925=CARTESIAN_POINT ( 'NONE',  ( 135.6228728715778971, 37.27929687499999289, 13.57481594606304576 ) ) ;
#6928=ORIENTED_EDGE ( 'NONE', *, *, #5500, .T. ) ;
#6929=FACE_OUTER_BOUND ( 'NONE', #4631, .T. ) ;
#6934=CARTESIAN_POINT ( 'NONE',  ( 120.7049497278729575, 32.71523437608393436, 9.295050272127047819 ) ) ;
#6935=CARTESIAN_POINT ( 'NONE',  ( 70.62287287157788285, 34.99726562716787726, 13.57481594606304576 ) ) ;
#6937=CARTESIAN_POINT ( 'NONE',  ( 13.57481594606304576, 33.55859375216787299, -1.662435489736055892E-15 ) ) ;
#6941=CARTESIAN_POINT ( 'NONE',  ( 185.7049497278729575, 35.09648437608392868, 9.295050272127047819 ) ) ;
#6943=CARTESIAN_POINT ( 'NONE',  ( 202.0894172723214126, 49.99999999943664619, 11.59823041029769541 ) ) ;
#6945=CARTESIAN_POINT ( 'NONE',  ( 103.5355339059327093, 81.37500000000000000, 3.535533905932726206 ) ) ;
#6946=CARTESIAN_POINT ( 'NONE',  ( 208.5748159460630688, 38.96601562499999005, 5.622872871577868636 ) ) ;
#6948=CARTESIAN_POINT ( 'NONE',  ( 51.42518405393695957, 40.30546875216787583, 0.000000000000000000 ) ) ;
#6953=CARTESIAN_POINT ( 'NONE',  ( 189.3771271284221314, 35.59257812499999574, 13.57481594606304753 ) ) ;
#6955=CARTESIAN_POINT ( 'NONE',  ( 135.6228728715778118, 36.48554687499999716, 13.57481594606309194 ) ) ;
#6956=CARTESIAN_POINT ( 'NONE',  ( 55.70494972787295751, 36.68398437608392726, 9.295050272127047819 ) ) ;
#6961=CARTESIAN_POINT ( 'NONE',  ( 13.57481594606304931, 36.58476562499999574, 5.622872871577869525 ) ) ;
#6962=CARTESIAN_POINT ( 'NONE',  ( 120.7049497278729575, 38.27148437608393294, -9.295050272127046043 ) ) ;
#6964=CARTESIAN_POINT ( 'NONE',  ( 103.5355339059327093, 81.37500000000000000, 3.535533905932726206 ) ) ;
#6966=CARTESIAN_POINT ( 'NONE',  ( 104.9999999999999574, 80.56250000273119838, 2.071067811865462627 ) ) ;
#6971=CARTESIAN_POINT ( 'NONE',  ( 51.42518405393695957, 40.95039062499999005, -5.622872871577873077 ) ) ;
#6972=ORIENTED_EDGE ( 'NONE', *, *, #8464, .F. ) ;
#6973=DIRECTION ( 'NONE',  ( 0.000000000000000000, 0.000000000000000000, -1.000000000000000000 ) ) ;
#6977=CARTESIAN_POINT ( 'NONE',  ( 200.6228728715778686, 33.70742187716787441, -13.57481594606304753 ) ) ;
#6980=CARTESIAN_POINT ( 'NONE',  ( 124.5550856135277087, 36.63437500108393863, -13.14518615778179722 ) ) ;
#6982=CARTESIAN_POINT ( 'NONE',  ( -13.14518615778179189, 34.45156250108394147, 5.444914386472304635 ) ) ;
#6983=EDGE_CURVE ( 'NONE', #12084, #12988, #12687, .T. ) ;
#6984=CARTESIAN_POINT ( 'NONE',  ( 139.2950502721270425, 32.91367187608393152, 9.295050272127046043 ) ) ;
#6985=CARTESIAN_POINT ( 'NONE',  ( 51.42518405393695957, 34.60039062499999574, -5.622872871577873077 ) ) ;
#6988=VECTOR ( 'NONE', #1398, 1000.000000000000000 ) ;
#6989=DIRECTION ( 'NONE',  ( 0.000000000000000000, 0.000000000000000000, 1.000000000000000000 ) ) ;
#6995=CARTESIAN_POINT ( 'NONE',  ( -13.14518615778179900, 35.93984375108393436, -5.444914386472297529 ) ) ;
#6999=CARTESIAN_POINT ( 'NONE',  ( -14.99999999999999822, 75.00000000000000000, 15.00000000000000000 ) ) ;
#7000=CARTESIAN_POINT ( 'NONE',  ( -15.00000000000000000, 75.00000000000000000, 9.999999999999998224 ) ) ;
#7001=CARTESIAN_POINT ( 'NONE',  ( 195.0000000000000000, 34.79882812608393294, -13.14518615778179544 ) ) ;
#7005=ORIENTED_EDGE ( 'NONE', *, *, #9687, .F. ) ;
#7009=CARTESIAN_POINT ( 'NONE',  ( 120.4011555911795455, 32.46718750216787441, 9.598844408820459861 ) ) ;
#7012=CARTESIAN_POINT ( 'NONE',  ( 51.85481384221820633, 36.78320312608393294, 0.000000000000000000 ) ) ;
#7013=CARTESIAN_POINT ( 'NONE',  ( 59.67620903604532145, 54.47170356488064868, -15.00000000000000000 ) ) ;
#7015=CARTESIAN_POINT ( 'NONE',  ( 200.4449143864723055, 32.26875000108393721, 13.14518615778179189 ) ) ;
#7021=CARTESIAN_POINT ( 'NONE',  ( 78.14518615778180788, 37.03125000108393294, -5.444914386472297529 ) ) ;
#7025=CARTESIAN_POINT ( 'NONE',  ( 200.4449143864723055, 37.82500000108392868, 13.14518615778179189 ) ) ;
#7032=CARTESIAN_POINT ( 'NONE',  ( 116.8548138422182205, 32.02070312608393010, 0.000000000000000000 ) ) ;
#7034=CARTESIAN_POINT ( 'NONE',  ( 185.7049497278729575, 33.50898437608393010, -9.295050272127046043 ) ) ;
#7035=ORIENTED_EDGE ( 'NONE', *, *, #13115, .F. ) ;
#7036=CARTESIAN_POINT ( 'NONE',  ( 5.444914386472297529, 32.36796875108393579, -13.14518615778179900 ) ) ;
#7043=CARTESIAN_POINT ( 'NONE',  ( 208.1451861577818079, 39.56132812608393579, -1.609821015232357215E-15 ) ) ;
#7044=VECTOR ( 'NONE', #25416, 1000.000000000000000 ) ;
#7045=ORIENTED_EDGE ( 'NONE', *, *, #23457, .T. ) ;
#7047=ORIENTED_EDGE ( 'NONE', *, *, #25412, .T. ) ;
#7050=CARTESIAN_POINT ( 'NONE',  ( 138.7693896720707301, 50.37710889400712233, 14.99999999999734079 ) ) ;
#7053=DIRECTION ( 'NONE',  ( 0.000000000000000000, -0.000000000000000000, 1.000000000000000000 ) ) ;
#7054=CYLINDRICAL_SURFACE ( 'NONE', #18354, 13.57481594606304398 ) ;
#7055=CARTESIAN_POINT ( 'NONE',  ( 51.85481384221819923, 35.14609375108393152, -5.444914386472297529 ) ) ;
#7057=CARTESIAN_POINT ( 'NONE',  ( -8.049105076161786076E-16, 37.18007812608393436, -13.14518615778179544 ) ) ;
#7059=AXIS2_PLACEMENT_3D ( 'NONE', #30, #17263, #25964 ) ;
#7061=CARTESIAN_POINT ( 'NONE',  ( 1.892183357089636475, 53.66387243067953960, 14.99999999999999645 ) ) ;
#7063=CARTESIAN_POINT ( 'NONE',  ( 124.3771271284221314, 37.97382812499999716, 13.57481594606304753 ) ) ;
#7064=ORIENTED_EDGE ( 'NONE', *, *, #8116, .F. ) ;
#7071=CARTESIAN_POINT ( 'NONE',  ( 135.4449143864723055, 33.95546875108393436, -13.14518615778179900 ) ) ;
#7072=CARTESIAN_POINT ( 'NONE',  ( 74.59884440882045453, 33.45937500216787441, 9.598844408820456309 ) ) ;
#7075=CARTESIAN_POINT ( 'NONE',  ( -13.57481594606304576, 33.21132812716787441, 5.622872871577880183 ) ) ;
#7079=CARTESIAN_POINT ( 'NONE',  ( 204.2950502721270425, 35.49335937608393010, -9.295050272127046043 ) ) ;
#7081=DIRECTION ( 'NONE',  ( 0.000000000000000000, 0.000000000000000000, 1.000000000000000000 ) ) ;
#7083=DIRECTION ( 'NONE',  ( 0.000000000000000000, 1.000000000000000000, 0.000000000000000000 ) ) ;
#7086=CARTESIAN_POINT ( 'NONE',  ( 130.0000000000000000, 38.02343749999999289, 13.57481594606304576 ) ) ;
#7089=CARTESIAN_POINT ( 'NONE',  ( 208.5748159460630120, 35.79101562499999289, 5.622872871577869525 ) ) ;
#7090=EDGE_CURVE ( 'NONE', #12549, #11568, #5907, .T. ) ;
#7093=CARTESIAN_POINT ( 'NONE',  ( 96.84719886470459471, 82.31250000136559208, -3.152801135295383084 ) ) ;
#7094=CARTESIAN_POINT ( 'NONE',  ( 78.14518615778179367, 35.39414062608393152, -1.609821015232357215E-15 ) ) ;
#7099=CARTESIAN_POINT ( 'NONE',  ( 9.598844408820456309, 33.55859375000000000, -9.598844408820458085 ) ) ;
#7100=CARTESIAN_POINT ( 'NONE',  ( 139.2950502721270425, 37.08085937608393579, 9.295050272127046043 ) ) ;
#7101=ORIENTED_EDGE ( 'NONE', *, *, #15580, .F. ) ;
#7102=CARTESIAN_POINT ( 'NONE',  ( 103.5355339059327093, 80.37500000000000000, 3.535533905932726206 ) ) ;
#7104=CARTESIAN_POINT ( 'NONE',  ( 96.46446609406721961, 82.00000000273119838, -3.535533905932755072 ) ) ;
#7105=AXIS2_PLACEMENT_3D ( 'NONE', #3757, #24997, #16295 ) ;
#7108=CARTESIAN_POINT ( 'NONE',  ( 68.75563815586001226, 31.78804748261757140, -13.14518615778179367 ) ) ;
#7110=B_SPLINE_CURVE_WITH_KNOTS ( 'NONE', 3,
 ( #8202, #16893, #20386, #16241, #21047, #3938, #1530, #10182, #12598, #5280, #873, #18892, #27602, #23324, #8062, #21324, #7255, #15945, #22671, #16757, #26953, #13944, #3143, #9684, #11810, #20533, #25457, #5938, #3797, #15157, #13156 ),
 .UNSPECIFIED., .F., .F.,
 ( 4, 2, 2, 2, 2, 2, 2, 2, 2, 2, 1, 2, 2, 2, 2, 4 ),
 ( 1.175569253024769036E-15, 0.001656255954914826172, 0.003312511909828477069, 0.004968767864742128400, 0.005796895842198994397, 0.006625023819655860395, 0.008281279774569594992, 0.009937535729483326988, 0.01325004763931079445, 0.01490630359422449695, 0.01656255954913820119, 0.01821881550405190370, 0.01987507145896560620, 0.02318758336879301468, 0.02484383932370672413, 0.02650009527862043010 ),
 .UNSPECIFIED. ) ;
#7114=CARTESIAN_POINT ( 'NONE',  ( 195.0000000000000000, 32.96328125216787441, -13.57481594606304576 ) ) ;
#7115=AXIS2_PLACEMENT_3D ( 'NONE', #12959, #25542, #19399 ) ;
#7116=ORIENTED_EDGE ( 'NONE', *, *, #25691, .T. ) ;
#7118=CARTESIAN_POINT ( 'NONE',  ( -5.622872871577767384, 40.85117187499999147, -13.57481594606315412 ) ) ;
#7120=CARTESIAN_POINT ( 'NONE',  ( 5.444914386472297529, 35.74140625108393721, -13.14518615778179900 ) ) ;
#7122=CARTESIAN_POINT ( 'NONE',  ( 59.37712712842213136, 32.11992187499999574, -13.57481594606304753 ) ) ;
#7123=AXIS2_PLACEMENT_3D ( 'NONE', #27227, #22516, #7680 ) ;
#7124=CARTESIAN_POINT ( 'NONE',  ( -13.14518615778179544, 40.55351562608393579, 0.000000000000000000 ) ) ;
#7133=CARTESIAN_POINT ( 'NONE',  ( -13.14518615778179544, 35.98945312608393721, 0.000000000000000000 ) ) ;
#7135=CARTESIAN_POINT ( 'NONE',  ( 120.4011555911795455, 36.93203124999999432, -9.598844408820458085 ) ) ;
#7139=EDGE_CURVE ( 'NONE', #12585, #4508, #17403, .T. ) ;
#7140=CARTESIAN_POINT ( 'NONE',  ( 181.8548138422182205, 34.99726562608393721, 0.000000000000000000 ) ) ;
#7141=ADVANCED_FACE ( 'NONE', ( #24247 ), #25819, .T. ) ;
#7142=ORIENTED_EDGE ( 'NONE', *, *, #2897, .F. ) ;
#7143=DIRECTION ( 'NONE',  ( -0.000000000000000000, -1.000000000000000000, -0.000000000000000000 ) ) ;
#7145=ORIENTED_EDGE ( 'NONE', *, *, #24323, .F. ) ;
#7148=CARTESIAN_POINT ( 'NONE',  ( 97.92893218813443923, 79.31250000273119838, 4.999999999999927169 ) ) ;
#7149=CARTESIAN_POINT ( 'NONE',  ( 116.8548138422182063, 36.63437500108393152, 5.444914386472304635 ) ) ;
#7150=CARTESIAN_POINT ( 'NONE',  ( 130.0000000000000000, 36.00000000000000000, -1.503427012513233026E-14 ) ) ;
#7151=CARTESIAN_POINT ( 'NONE',  ( 13.14518615778179900, 36.23750000108393010, -5.444914386472297529 ) ) ;
#7153=CARTESIAN_POINT ( 'NONE',  ( 74.29505027212704249, 36.48554687608393721, -9.295050272127046043 ) ) ;
#7154=CARTESIAN_POINT ( 'NONE',  ( 55.81982418635197973, 55.00000000000000000, -15.00000000000000000 ) ) ;
#7156=CARTESIAN_POINT ( 'NONE',  ( 204.5988444088204403, 40.70234374999999716, -9.598844408820458085 ) ) ;
#7161=CARTESIAN_POINT ( 'NONE',  ( 70.44491438647229131, 38.42031250108393436, 13.14518615778179189 ) ) ;
#7162=CARTESIAN_POINT ( 'NONE',  ( 51.42518405393695957, 38.56914062499999574, -5.622872871577872189 ) ) ;
#7166=CARTESIAN_POINT ( 'NONE',  ( 208.1451861577818079, 38.81718750108393579, -5.444914386472297529 ) ) ;
#7168=ORIENTED_EDGE ( 'NONE', *, *, #15254, .F. ) ;
#7172=CARTESIAN_POINT ( 'NONE',  ( 139.2950502721270425, 33.31054687608394005, -9.295050272127046043 ) ) ;
#7173=CARTESIAN_POINT ( 'NONE',  ( 51.85481384221820633, 31.82226562608393650, 0.000000000000000000 ) ) ;
#7174=CARTESIAN_POINT ( 'NONE',  ( 181.8548138422181921, 35.14609375108393152, -5.444914386472297529 ) ) ;
#7183=CARTESIAN_POINT ( 'NONE',  ( 74.18017581364802027, 50.00000000000000000, 9.999999999999966249 ) ) ;
#7186=CARTESIAN_POINT ( 'NONE',  ( -11.14554687309540348, 36.00000000000000711, -7.260818043107225783 ) ) ;
#7188=CARTESIAN_POINT ( 'NONE',  ( 143.5748159460630688, 38.27148437716787299, 5.622872871577868636 ) ) ;
#7189=AXIS2_PLACEMENT_3D ( 'NONE', #16041, #20055, #826 ) ;
#7191=CARTESIAN_POINT ( 'NONE',  ( 0.2703369776638426258, 35.99999999999999289, 13.14949859323921721 ) ) ;
#7192=CARTESIAN_POINT ( 'NONE',  ( 2.385244779468109360E-15, 75.00000000000000000, 9.999999999999996447 ) ) ;
#7194=EDGE_CURVE ( 'NONE', #19665, #8206, #320, .T. ) ;
#7196=CARTESIAN_POINT ( 'NONE',  ( -5.444914386472297529, 38.81718750108393579, -13.14518615778179722 ) ) ;
#7198=CARTESIAN_POINT ( 'NONE',  ( -8.211314015175641856, 50.68678854790643840, 15.00000000000000178 ) ) ;
#7200=CARTESIAN_POINT ( 'NONE',  ( 120.4011555911795455, 35.54296874999999289, 9.598844408820459861 ) ) ;
#7207=CARTESIAN_POINT ( 'NONE',  ( 143.1451861577818079, 33.75703125108393010, 5.444914386472293977 ) ) ;
#7209=CARTESIAN_POINT ( 'NONE',  ( 70.44491438647230552, 40.30546875108393579, -13.14518615778179900 ) ) ;
#7210=ADVANCED_FACE ( 'NONE', ( #4876 ), #2869, .T. ) ;
#7212=CARTESIAN_POINT ( 'NONE',  ( 99.99999999999995737, 80.75000000000000000, -5.000000000000018652 ) ) ;
#7213=CARTESIAN_POINT ( 'NONE',  ( -13.14518615778179189, 38.22187500108393010, 5.444914386472304635 ) ) ;
#7218=AXIS2_PLACEMENT_3D ( 'NONE', #5982, #7971, #3710 ) ;
#7219=CARTESIAN_POINT ( 'NONE',  ( 185.7049497278729575, 35.69179687608393436, -9.295050272127046043 ) ) ;
#7224=CARTESIAN_POINT ( 'NONE',  ( 195.0000000000000000, -7.395377635281828788, -2.255140518769849538E-14 ) ) ;
#7226=DIRECTION ( 'NONE',  ( -0.000000000000000000, -1.000000000000000000, -0.000000000000000000 ) ) ;
#7233=DIRECTION ( 'NONE',  ( 0.000000000000000000, 0.000000000000000000, -1.000000000000000000 ) ) ;
#7234=CARTESIAN_POINT ( 'NONE',  ( 101.8468681455906903, 82.75000000136560629, 4.458734124999987891 ) ) ;
#7235=CARTESIAN_POINT ( 'NONE',  ( 78.14518615778179367, 32.26875000108393721, -5.444914386472297529 ) ) ;
#7240=CARTESIAN_POINT ( 'NONE',  ( -13.57481594606304576, 33.11210937499999574, 5.622872871577880183 ) ) ;
#7241=CARTESIAN_POINT ( 'NONE',  ( 135.4449143864723055, 36.53515625108393294, -13.14518615778179900 ) ) ;
#7242=ADVANCED_FACE ( 'NONE', ( #22689 ), #17831, .F. ) ;
#7243=ORIENTED_EDGE ( 'NONE', *, *, #10229, .F. ) ;
#7246=CARTESIAN_POINT ( 'NONE',  ( 195.0000000000000000, 36.53515625216787299, 13.57481594606304576 ) ) ;
#7247=CARTESIAN_POINT ( 'NONE',  ( 96.84719886470459471, 83.31250000136560629, -3.152801135295383084 ) ) ;
#7250=CARTESIAN_POINT ( 'NONE',  ( 51.42518405393695957, 39.46210937716787726, -5.622872871577873077 ) ) ;
#7251=ADVANCED_FACE ( 'NONE', ( #11970 ), #15686, .T. ) ;
#7253=CARTESIAN_POINT ( 'NONE',  ( 59.37712712842213136, 40.05742187499999574, -13.57481594606304753 ) ) ;
#7255=CARTESIAN_POINT ( 'NONE',  ( 187.6059679576637507, 36.00000000000000000, -11.20317769887076764 ) ) ;
#7260=CARTESIAN_POINT ( 'NONE',  ( 189.3771271284221314, 33.80664062716786589, -13.57481594606304753 ) ) ;
#7263=DIRECTION ( 'NONE',  ( 0.8660254037844418162, 0.4999999999999947264, 0.000000000000000000 ) ) ;
#7264=CARTESIAN_POINT ( 'NONE',  ( -5.444914386472297529, 35.84062500108394289, -13.14518615778179900 ) ) ;
#7267=CARTESIAN_POINT ( 'NONE',  ( 78.57481594606304043, 32.61601562499999574, 5.622872871577869525 ) ) ;
#7272=CYLINDRICAL_SURFACE ( 'NONE', #8952, 13.57481594606304398 ) ;
#7275=DIRECTION ( 'NONE',  ( -0.000000000000000000, 1.000000000000000000, -0.000000000000000000 ) ) ;
#7276=CARTESIAN_POINT ( 'NONE',  ( 65.00000000000000000, -7.395377635281828788, -7.517135062566165128E-15 ) ) ;
#7277=CARTESIAN_POINT ( 'NONE',  ( 0.000000000000000000, 36.00000000000000000, 0.000000000000000000 ) ) ;
#7278=CARTESIAN_POINT ( 'NONE',  ( -9.295050272127046043, 31.92148437608393508, -9.295050272127046043 ) ) ;
#7280=ORIENTED_EDGE ( 'NONE', *, *, #16085, .F. ) ;
#7285=CARTESIAN_POINT ( 'NONE',  ( 181.8548138422181921, 36.63437500108393152, 5.444914386472304635 ) ) ;
#7286=ORIENTED_EDGE ( 'NONE', *, *, #973, .F. ) ;
#7289=AXIS2_PLACEMENT_3D ( 'NONE', #23861, #12581, #21307 ) ;
#7293=CARTESIAN_POINT ( 'NONE',  ( -20.00000000000000000, 55.00000000000000000, 10.00000000000000178 ) ) ;
#7295=CARTESIAN_POINT ( 'NONE',  ( 116.8548138422182205, 38.17226562608393436, 0.000000000000000000 ) ) ;
#7296=CARTESIAN_POINT ( 'NONE',  ( 9.295050272127047819, 37.08085937608393579, 9.295050272127046043 ) ) ;
#7297=CARTESIAN_POINT ( 'NONE',  ( -9.295050272127046043, 36.48554687608393721, -9.295050272127046043 ) ) ;
#7301=CARTESIAN_POINT ( 'NONE',  ( -9.598844408820454532, 36.43593750216787441, 9.598844408820459861 ) ) ;
#7303=CARTESIAN_POINT ( 'NONE',  ( 76.20653150213495053, 36.00000000000000000, 7.323573988461856032 ) ) ;
#7307=CARTESIAN_POINT ( 'NONE',  ( 78.14518615778180788, 38.51953125108393294, 5.444914386472293977 ) ) ;
#7309=CARTESIAN_POINT ( 'NONE',  ( 204.2950502721270425, 36.28710937608393294, -9.295050272127046043 ) ) ;
#7310=EDGE_LOOP ( 'NONE', ( #7887, #26941, #6804, #10999 ) ) ;
#7314=CARTESIAN_POINT ( 'NONE',  ( 204.2950502721270425, 37.27929687608394005, -9.295050272127046043 ) ) ;
#7319=ORIENTED_EDGE ( 'NONE', *, *, #14895, .F. ) ;
#7320=CARTESIAN_POINT ( 'NONE',  ( 139.2950502721270425, 33.90585937608393863, 9.295050272127046043 ) ) ;
#7321=CARTESIAN_POINT ( 'NONE',  ( 59.55508561352770158, 31.97109375108393436, 13.14518615778179722 ) ) ;
#7322=CARTESIAN_POINT ( 'NONE',  ( 204.2950502721270425, 34.69960937608393436, 9.295050272127046043 ) ) ;
#7325=CARTESIAN_POINT ( 'NONE',  ( 4.925026783667639130, 49.99999999893164215, -12.67776588291819095 ) ) ;
#7328=CARTESIAN_POINT ( 'NONE',  ( 139.5988444088204403, 37.62656250216787157, -9.598844408820458085 ) ) ;
#7332=CARTESIAN_POINT ( 'NONE',  ( 65.72387193802225624, 53.51529642094862282, 14.99999999999997868 ) ) ;
#7333=EDGE_CURVE ( 'NONE', #11913, #4741, #18474, .T. ) ;
#7335=VERTEX_POINT ( 'NONE', #27448 ) ;
#7336=CARTESIAN_POINT ( 'NONE',  ( -13.17415721692276165, 36.00000000000000000, 0.03826467346021143745 ) ) ;
#7341=CARTESIAN_POINT ( 'NONE',  ( 78.14518615778179367, 33.16171875108393863, 5.444914386472293977 ) ) ;
#7342=CARTESIAN_POINT ( 'NONE',  ( -5.622872871577767384, 40.15664062716787441, -13.57481594606315412 ) ) ;
#7343=PLANE ( 'NONE',  #9853 ) ;
#7345=CARTESIAN_POINT ( 'NONE',  ( -4.571591632531241345, 51.44262710532056815, 15.00000000000065548 ) ) ;
#7347=CARTESIAN_POINT ( 'NONE',  ( 143.5748159460630404, 34.99726562500000426, 5.622872871577869525 ) ) ;
#7350=FACE_BOUND ( 'NONE', #23140, .T. ) ;
#7354=CARTESIAN_POINT ( 'NONE',  ( 124.5550856135277087, 32.76484375108393010, 13.14518615778179722 ) ) ;
#7355=CARTESIAN_POINT ( 'NONE',  ( 51.42518405393695957, 32.31835937716786589, -5.622872871577873077 ) ) ;
#7356=CARTESIAN_POINT ( 'NONE',  ( 104.9999999999999716, 80.56250000000004263, -2.071067811865491937 ) ) ;
#7357=CARTESIAN_POINT ( 'NONE',  ( 5.444914386472302859, 37.62656250108393863, 13.14518615778179189 ) ) ;
#7362=CARTESIAN_POINT ( 'NONE',  ( 102.0710678118654187, 82.43750000273119838, 5.000000000000011546 ) ) ;
#7367=DIRECTION ( 'NONE',  ( 0.000000000000000000, 0.000000000000000000, 1.000000000000000000 ) ) ;
#7378=CARTESIAN_POINT ( 'NONE',  ( 78.14518615778179367, 33.80664062608393294, -1.609821015232357215E-15 ) ) ;
#7379=EDGE_CURVE ( 'NONE', #22018, #1696, #19073, .T. ) ;
#7382=( BOUNDED_CURVE ( )  B_SPLINE_CURVE ( 2, ( #7894, #16445, #5768, #1495, #27301, #12428, #1773, #14437, #14297 ),
 .UNSPECIFIED., .F., .T. ) 
 B_SPLINE_CURVE_WITH_KNOTS ( ( 3, 2, 2, 2, 3 ),
 ( 0.3541666666666666852, 0.3645833333333332593, 0.3749999999999998890, 0.3854166666666665741, 0.3958333333333331483 ),
 .UNSPECIFIED. ) 
 CURVE ( )  GEOMETRIC_REPRESENTATION_ITEM ( )  RATIONAL_B_SPLINE_CURVE ( ( 1.000000000000000000, 0.9238795325112867385, 1.000000000000000000, 0.9238795325112867385, 1.000000000000000000, 0.9238795325112867385, 1.000000000000000000, 0.9238795325112879597, 0.9999999999999987788 ) ) 
 REPRESENTATION_ITEM ( '' )  );
#7383=CARTESIAN_POINT ( 'NONE',  ( -5.622872871577873077, 32.91367187499999858, -13.57481594606304753 ) ) ;
#7384=CARTESIAN_POINT ( 'NONE',  ( 124.5550856135277087, 34.55078125108393294, 13.14518615778179722 ) ) ;
#7386=CARTESIAN_POINT ( 'NONE',  ( 97.92893218813451028, 82.18750000000000000, 4.999999999999989342 ) ) ;
#7387=CARTESIAN_POINT ( 'NONE',  ( 74.59884440882045453, 38.42031250216787441, -9.598844408820458085 ) ) ;
#7388=CARTESIAN_POINT ( 'NONE',  ( 96.84719886470459471, 82.31250000136559208, -3.152801135295383084 ) ) ;
#7390=CARTESIAN_POINT ( 'NONE',  ( 70.62287287157788285, 39.75976562716787299, 13.57481594606304576 ) ) ;
#7391=EDGE_CURVE ( 'NONE', #27982, #8588, #15071, .T. ) ;
#7393=CARTESIAN_POINT ( 'NONE',  ( 70.62287287157788285, 39.66054687500000142, 13.57481594606304576 ) ) ;
#7394=CARTESIAN_POINT ( 'NONE',  ( -8.312177448680279460E-16, 38.51953125216787299, -13.57481594606304576 ) ) ;
#7396=CYLINDRICAL_SURFACE ( 'NONE', #4900, 13.57481594606304398 ) ;
#7401=CARTESIAN_POINT ( 'NONE',  ( 185.7049497278729575, 39.85898437608393152, 9.295050272127047819 ) ) ;
#7403=PRODUCT ( 'Vacuum Distribution Tubing Harness', 'Vacuum Distribution Tubing Harness', '', ( #21095 ) ) ;
#7405=CARTESIAN_POINT ( 'NONE',  ( 139.2950502721270425, 40.25585937608393294, -9.295050272127046043 ) ) ;
#7406=CARTESIAN_POINT ( 'NONE',  ( 13.14518615778179900, 36.43593750108392726, -5.444914386472297529 ) ) ;
#7412=LINE ( 'NONE', #18401, #13632 ) ;
#7418=CARTESIAN_POINT ( 'NONE',  ( 130.0000000000000000, -7.395377635281828788, -1.503427012513233026E-14 ) ) ;
#7419=CARTESIAN_POINT ( 'NONE',  ( 9.295050272127046043, 34.89804687608393863, -9.295050272127046043 ) ) ;
#7422=CARTESIAN_POINT ( 'NONE',  ( 130.0000000000000000, 37.22968749999999716, 13.57481594606304576 ) ) ;
#7426=CARTESIAN_POINT ( 'NONE',  ( 185.7049497278729575, 36.68398437608392726, 9.295050272127047819 ) ) ;
#7428=CARTESIAN_POINT ( 'NONE',  ( 194.5539587432196527, 49.99999999978076204, -13.57776691409238268 ) ) ;
#7433=DIRECTION ( 'NONE',  ( 0.000000000000000000, -1.000000000000000000, 0.000000000000000000 ) ) ;
#7434=DIRECTION ( 'NONE',  ( 0.000000000000000000, 0.000000000000000000, 1.000000000000000000 ) ) ;
#7435=CARTESIAN_POINT ( 'NONE',  ( 135.4449143864723055, 38.71796875108393721, -13.14518615778179900 ) ) ;
#7436=CARTESIAN_POINT ( 'NONE',  ( -9.295050272127044266, 37.67617187608393436, 9.295050272127047819 ) ) ;
#7438=CARTESIAN_POINT ( 'NONE',  ( 5.444914386472297529, 33.95546875108393436, -13.14518615778179900 ) ) ;
#7440=CARTESIAN_POINT ( 'NONE',  ( 62.47041600482873491, 49.99999999938352602, -13.34625891065891778 ) ) ;
#7447=CARTESIAN_POINT ( 'NONE',  ( 78.14518615778180788, 36.93203125108394147, 5.444914386472293977 ) ) ;
#7448=MANIFOLD_SOLID_BREP ( 'Thread1', #21742 ) ;
#7450=CARTESIAN_POINT ( 'NONE',  ( 55.40115559117954547, 36.23750000216787726, -9.598844408820458085 ) ) ;
#7455=CARTESIAN_POINT ( 'NONE',  ( 208.1451861577818079, 38.02343750108395426, -5.444914386472297529 ) ) ;
#7457=ORIENTED_EDGE ( 'NONE', *, *, #16085, .T. ) ;
#7460=VERTEX_POINT ( 'NONE', #23724 ) ;
#7461=CARTESIAN_POINT ( 'NONE',  ( 124.5550856135277087, 31.87187500108393223, -13.14518615778179900 ) ) ;
#7462=CARTESIAN_POINT ( 'NONE',  ( 59.55508561352770158, 40.10703125108393152, 13.14518615778179722 ) ) ;
#7464=CARTESIAN_POINT ( 'NONE',  ( 189.5550856135277229, 35.34453125108393579, 13.14518615778179722 ) ) ;
#7468=( BOUNDED_CURVE ( )  B_SPLINE_CURVE ( 2, ( #6669, #22221, #272, #2700, #17647, #15355, #2420, #6955, #13208 ),
 .UNSPECIFIED., .F., .F. ) 
 B_SPLINE_CURVE_WITH_KNOTS ( ( 3, 2, 2, 2, 3 ),
 ( 0.4375000000000003331, 0.4479166666666669627, 0.4583333333333335369, 0.4687500000000001665, 0.4791666666666667962 ),
 .UNSPECIFIED. ) 
 CURVE ( )  GEOMETRIC_REPRESENTATION_ITEM ( )  RATIONAL_B_SPLINE_CURVE ( ( 0.9999999999999975575, 0.9238795325112891810, 1.000000000000000000, 0.9238795325112867385, 1.000000000000000000, 0.9238795325112867385, 1.000000000000000000, 0.9238795325112859613, 1.000000000000000888 ) ) 
 REPRESENTATION_ITEM ( '' )  );
#7469=CARTESIAN_POINT ( 'NONE',  ( 135.6228728715778971, 38.17226562716786731, 13.57481594606304576 ) ) ;
#7471=CARTESIAN_POINT ( 'NONE',  ( 51.42518405393695957, 40.25585937716787299, -5.622872871577872189 ) ) ;
#7473=CARTESIAN_POINT ( 'NONE',  ( 65.44604125677763307, 49.99999999978076914, 13.57776691409234715 ) ) ;
#7479=CARTESIAN_POINT ( 'NONE',  ( -2.086998648631069653, 36.00000000000000000, -13.31420566034952202 ) ) ;
#7481=CARTESIAN_POINT ( 'NONE',  ( 195.0000000000000000, 38.02343749999999289, 13.57481594606304576 ) ) ;
#7483=CARTESIAN_POINT ( 'NONE',  ( 51.85481384221820633, 32.02070312608393010, 0.000000000000000000 ) ) ;
#7489=CARTESIAN_POINT ( 'NONE',  ( 0.8765262653613452581, 51.45968077934942642, 14.99999999999965716 ) ) ;
#7490=CARTESIAN_POINT ( 'NONE',  ( 139.5988444088204687, 40.50390624999999289, 9.598844408820456309 ) ) ;
#7491=CARTESIAN_POINT ( 'NONE',  ( 124.3771271284221314, 35.59257812499999574, 13.57481594606304753 ) ) ;
#7498=CARTESIAN_POINT ( 'NONE',  ( 116.8548138422182063, 34.94765625108392726, -5.444914386472297529 ) ) ;
#7499=CARTESIAN_POINT ( 'NONE',  ( 59.55508561352770158, 39.61093750108393152, -13.14518615778179900 ) ) ;
#7500=EDGE_LOOP ( 'NONE', ( #6558, #12302, #4917, #15550 ) ) ;
#7503=CARTESIAN_POINT ( 'NONE',  ( 5.444914386472297529, 37.92421875108392726, -13.14518615778179900 ) ) ;
#7510=CARTESIAN_POINT ( 'NONE',  ( 143.4064236467344813, 36.00000000000000000, 1.227293221035692161 ) ) ;
#7513=CARTESIAN_POINT ( 'NONE',  ( 195.0000000000000000, 39.21406249999999716, -13.57481594606304576 ) ) ;
#7514=( BOUNDED_CURVE ( )  B_SPLINE_CURVE ( 2, ( #10853, #6587, #1776, #25698, #2333, #2049, #10991, #12712, #10440 ),
 .UNSPECIFIED., .F., .T. ) 
 B_SPLINE_CURVE_WITH_KNOTS ( ( 3, 2, 2, 2, 3 ),
 ( 0.5500000000000004885, 0.5750000000000003997, 0.6000000000000005329, 0.6250000000000005551, 0.6500000000000005773 ),
 .UNSPECIFIED. ) 
 CURVE ( )  GEOMETRIC_REPRESENTATION_ITEM ( )  RATIONAL_B_SPLINE_CURVE ( ( 0.9999999999999986677, 0.9238795325112880708, 1.000000000000000000, 0.9238795325112867385, 1.000000000000000000, 0.9238795325112867385, 1.000000000000000000, 0.9238795325112850731, 1.000000000000001776 ) ) 
 REPRESENTATION_ITEM ( '' )  );
#7515=CARTESIAN_POINT ( 'NONE',  ( 189.3771271284221029, 39.66054687716787441, 13.57481594606302444 ) ) ;
#7516=CARTESIAN_POINT ( 'NONE',  ( 195.0000000000000000, 38.91640625216786731, 13.57481594606304576 ) ) ;
#7524=CARTESIAN_POINT ( 'NONE',  ( 101.8468681455906903, 84.12500000136560629, -4.458734125000016313 ) ) ;
#7525=CARTESIAN_POINT ( 'NONE',  ( 51.85481384221820633, 33.40976562608393863, 0.000000000000000000 ) ) ;
#7527=DIRECTION ( 'NONE',  ( -0.000000000000000000, 1.000000000000000000, -0.000000000000000000 ) ) ;
#7529=CARTESIAN_POINT ( 'NONE',  ( 5.622872871577878406, 33.31054687499999289, 13.57481594606304576 ) ) ;
#7531=CARTESIAN_POINT ( 'NONE',  ( 124.5550856135277087, 32.96328125108393436, 13.14518615778179722 ) ) ;
#7533=CARTESIAN_POINT ( 'NONE',  ( 94.99999999999995737, 80.06250000000001421, 2.071067811865466624 ) ) ;
#7534=VECTOR ( 'NONE', #10569, 1000.000000000000000 ) ;
#7536=CARTESIAN_POINT ( 'NONE',  ( 104.4587341249999781, 82.87500000136560629, 1.846868145590721655 ) ) ;
#7538=CARTESIAN_POINT ( 'NONE',  ( 130.0000000000000000, 38.81718749999999574, 13.57481594606304576 ) ) ;
#7540=CARTESIAN_POINT ( 'NONE',  ( 208.1451861577817795, 32.16953125108393152, 5.444914386472293977 ) ) ;
#7542=CIRCLE ( 'NONE', #16183, 13.57481594606304398 ) ;
#7544=CARTESIAN_POINT ( 'NONE',  ( 51.42518405393695957, 36.18789062499999432, -5.622872871577872189 ) ) ;
#7549=CARTESIAN_POINT ( 'NONE',  ( 181.4251840539369596, 31.52460937716787370, -5.622872871577873077 ) ) ;
#7554=CARTESIAN_POINT ( 'NONE',  ( 135.4449143864723055, 32.36796875108393579, -13.14518615778179900 ) ) ;
#7564=CARTESIAN_POINT ( 'NONE',  ( 200.6228728715778118, 39.95820312499999716, -13.57481594606312036 ) ) ;
#7565=DIRECTION ( 'NONE',  ( -0.000000000000000000, 1.000000000000000000, -0.000000000000000000 ) ) ;
#7566=CARTESIAN_POINT ( 'NONE',  ( 2.414731522848535132E-15, 33.01289062608393721, 13.14518615778179544 ) ) ;
#7567=ORIENTED_EDGE ( 'NONE', *, *, #13115, .T. ) ;
#7570=CARTESIAN_POINT ( 'NONE',  ( -15.00000000000000000, 80.00000000000000000, 10.00000000000000000 ) ) ;
#7571=CARTESIAN_POINT ( 'NONE',  ( 181.8548138422181921, 33.36015625108393579, -5.444914386472297529 ) ) ;
#7574=ADVANCED_FACE ( 'NONE', ( #21030 ), #12440, .T. ) ;
#7575=CARTESIAN_POINT ( 'NONE',  ( 191.3635037532015986, 51.46815297079189122, -15.00000000000068745 ) ) ;
#7577=EDGE_CURVE ( 'NONE', #2045, #3877, #6139, .T. ) ;
#7578=ORIENTED_EDGE ( 'NONE', *, *, #4113, .T. ) ;
#7582=CARTESIAN_POINT ( 'NONE',  ( 181.4251840539369596, 39.56132812716787583, 5.622872871577880183 ) ) ;
#7583=CARTESIAN_POINT ( 'NONE',  ( 13.57481594606304931, 38.96601562499999005, 5.622872871577868636 ) ) ;
#7585=CARTESIAN_POINT ( 'NONE',  ( 120.7049497278729575, 38.27148437608393294, 9.295050272127047819 ) ) ;
#7586=CARTESIAN_POINT ( 'NONE',  ( -9.295050272127046043, 39.06523437608392868, -9.295050272127046043 ) ) ;
#7587=CARTESIAN_POINT ( 'NONE',  ( 9.295050272127046043, 40.45429687608393721, -9.295050272127046043 ) ) ;
#7593=ORIENTED_EDGE ( 'NONE', *, *, #11866, .T. ) ;
#7597=VECTOR ( 'NONE', #12584, 1000.000000000000000 ) ;
#7598=CARTESIAN_POINT ( 'NONE',  ( 70.44491438647229131, 37.13046875108393152, -13.14518615778179722 ) ) ;
#7602=ORIENTED_EDGE ( 'NONE', *, *, #17472, .T. ) ;
#7608=EDGE_CURVE ( 'NONE', #1369, #20160, #13141, .T. ) ;
#7613=CARTESIAN_POINT ( 'NONE',  ( 51.85481384221820633, 40.70234375108392300, -5.444914386472297529 ) ) ;
#7615=CARTESIAN_POINT ( 'NONE',  ( 189.5550856135277229, 33.45937500108394147, -13.14518615778179900 ) ) ;
#7617=CARTESIAN_POINT ( 'NONE',  ( 74.18017581364799184, 50.00000000000000000, -9.999999999999998224 ) ) ;
#7619=CARTESIAN_POINT ( 'NONE',  ( 6.450879342659026960, 50.00000000106836495, -11.97362904075607482 ) ) ;
#7620=CARTESIAN_POINT ( 'NONE',  ( 67.12981065842747341, 36.02027164734404607, -13.57481594606306352 ) ) ;
#7623=CARTESIAN_POINT ( 'NONE',  ( 135.6228728715778971, 37.37851562716787157, 13.57481594606304576 ) ) ;
#7626=CARTESIAN_POINT ( 'NONE',  ( 200.4449143864723055, 39.41250000108393436, 13.14518615778179189 ) ) ;
#7627=ORIENTED_EDGE ( 'NONE', *, *, #8158, .F. ) ;
#7629=CARTESIAN_POINT ( 'NONE',  ( 0.3745404134779373173, 36.00000000000003553, -13.51869779562201757 ) ) ;
#7631=CARTESIAN_POINT ( 'NONE',  ( -4.374022130818334020, 36.00000000000000711, 12.40367315690567018 ) ) ;
#7632=CARTESIAN_POINT ( 'NONE',  ( 59.55508561352770158, 31.87187500108393223, -13.14518615778179900 ) ) ;
#7635=CARTESIAN_POINT ( 'NONE',  ( 9.598844408820459861, 40.50390624999999289, 9.598844408820456309 ) ) ;
#7637=CARTESIAN_POINT ( 'NONE',  ( 2.024627725537271772, 50.00000000050963678, 13.43320860980897535 ) ) ;
#7639=CARTESIAN_POINT ( 'NONE',  ( 116.4251840539369454, 33.80664062500000000, -5.622872871577873077 ) ) ;
#7641=ORIENTED_EDGE ( 'NONE', *, *, #10, .T. ) ;
#7645=( BOUNDED_CURVE ( )  B_SPLINE_CURVE ( 2, ( #9947, #18661, #7387, #1006, #2844, #9675, #7823, #5126, #16516 ),
 .UNSPECIFIED., .F., .F. ) 
 B_SPLINE_CURVE_WITH_KNOTS ( ( 3, 2, 2, 2, 3 ),
 ( 0.1875000000000001388, 0.1979166666666667407, 0.2083333333333333703, 0.2187499999999999722, 0.2291666666666665741 ),
 .UNSPECIFIED. ) 
 CURVE ( )  GEOMETRIC_REPRESENTATION_ITEM ( )  RATIONAL_B_SPLINE_CURVE ( ( 0.9999999999999990008, 0.9238795325112877377, 1.000000000000000000, 0.9238795325112867385, 1.000000000000000000, 0.9238795325112867385, 1.000000000000000000, 0.9238795325112872936, 0.9999999999999994449 ) ) 
 REPRESENTATION_ITEM ( '' )  );
#7647=CARTESIAN_POINT ( 'NONE',  ( 116.8548138422182063, 31.77265625108393365, -5.444914386472297529 ) ) ;
#7648=CARTESIAN_POINT ( 'NONE',  ( 70.44491438647230552, 40.00781250108393294, 13.14518615778179189 ) ) ;
#7650=CARTESIAN_POINT ( 'NONE',  ( 2.493653234604083739E-15, 37.32890625216786873, 13.57481594606304576 ) ) ;
#7651=CARTESIAN_POINT ( 'NONE',  ( 2.414731522848535132E-15, 38.37070312608393152, 13.14518615778179544 ) ) ;
#7653=CARTESIAN_POINT ( 'NONE',  ( 65.00000000000000000, 37.62656249999999858, -13.57481594606304576 ) ) ;
#7655=CARTESIAN_POINT ( 'NONE',  ( 208.5748159460630688, 40.55351562499999574, 5.622872871577868636 ) ) ;
#7656=CARTESIAN_POINT ( 'NONE',  ( -13.14518615778179544, 40.55351562608393579, 0.000000000000000000 ) ) ;
#7657=CARTESIAN_POINT ( 'NONE',  ( 219.9999999999999716, 55.00000000000000000, -15.00000000000000000 ) ) ;
#7658=CARTESIAN_POINT ( 'NONE',  ( -15.00000000000000000, 75.00000000000000000, 10.00000000000000000 ) ) ;
#7662=CARTESIAN_POINT ( 'NONE',  ( 0.000000000000000000, 50.00000000000000000, 0.000000000000000000 ) ) ;
#7665=CARTESIAN_POINT ( 'NONE',  ( 130.0000000000000000, 50.00000000000000000, -13.57481594606305997 ) ) ;
#7668=CARTESIAN_POINT ( 'NONE',  ( 198.8783852973912474, 32.03609435653363136, -13.57481594606304576 ) ) ;
#7670=CARTESIAN_POINT ( 'NONE',  ( 103.1528011352953342, 84.06250000136560629, -3.152801135295383084 ) ) ;
#7671=CARTESIAN_POINT ( 'NONE',  ( 55.70494972787295751, 40.65273437608393436, -9.295050272127046043 ) ) ;
#7673=CYLINDRICAL_SURFACE ( 'NONE', #21409, 11.57481594606304398 ) ;
#7675=CARTESIAN_POINT ( 'NONE',  ( 9.598844408820459861, 32.56640625000000000, 9.598844408820456309 ) ) ;
#7677=CARTESIAN_POINT ( 'NONE',  ( 130.0000000000000000, 34.20351562608394147, -13.14518615778179544 ) ) ;
#7679=CARTESIAN_POINT ( 'NONE',  ( 135.6228728715777834, 37.67617187716787441, -13.57481594606313990 ) ) ;
#7680=DIRECTION ( 'NONE',  ( 0.000000000000000000, 0.000000000000000000, 1.000000000000000000 ) ) ;
#7681=CARTESIAN_POINT ( 'NONE',  ( 98.15313185440925281, 84.25000000136559208, -4.458734125000016313 ) ) ;
#7686=CARTESIAN_POINT ( 'NONE',  ( 181.8548138422181921, 31.77265625108393365, -5.444914386472297529 ) ) ;
#7688=CARTESIAN_POINT ( 'NONE',  ( -13.57481594606304576, 38.71796875216787726, 0.000000000000000000 ) ) ;
#7691=ORIENTED_EDGE ( 'NONE', *, *, #4785, .T. ) ;
#7694=CARTESIAN_POINT ( 'NONE',  ( 204.5988444088204403, 32.86406250216787583, -9.598844408820458085 ) ) ;
#7695=CYLINDRICAL_SURFACE ( 'NONE', #21708, 13.57481594606304398 ) ;
#7697=CARTESIAN_POINT ( 'NONE',  ( 143.1451861577818363, 40.10703125108393152, 5.444914386472293977 ) ) ;
#7698=CARTESIAN_POINT ( 'NONE',  ( -13.14518615778179900, 32.76484375108393010, -5.444914386472297529 ) ) ;
#7699=FACE_OUTER_BOUND ( 'NONE', #10574, .T. ) ;
#7700=CARTESIAN_POINT ( 'NONE',  ( 65.00000000000000000, 32.46718749999999432, 13.57481594606304576 ) ) ;
#7702=CARTESIAN_POINT ( 'NONE',  ( 181.4251840539369596, 39.41249999999999432, 0.000000000000000000 ) ) ;
#7703=CARTESIAN_POINT ( 'NONE',  ( 118.7351811978182781, 36.00000000000000000, 6.828991891054703167 ) ) ;
#7705=DIRECTION ( 'NONE',  ( 1.000000000000000000, 0.000000000000000000, 0.000000000000000000 ) ) ;
#7706=EDGE_CURVE ( 'NONE', #2793, #11153, #7712, .T. ) ;
#7712=CIRCLE ( 'NONE', #11321, 13.57481594606304398 ) ;
#7714=CARTESIAN_POINT ( 'NONE',  ( 13.14518615778179900, 33.26093750108393721, -5.444914386472297529 ) ) ;
#7715=VERTEX_POINT ( 'NONE', #21136 ) ;
#7716=CARTESIAN_POINT ( 'NONE',  ( 116.4251840539369738, 37.08085937499999574, 5.622872871577880183 ) ) ;
#7718=CARTESIAN_POINT ( 'NONE',  ( 204.2950502721270425, 33.70742187608393436, 9.295050272127046043 ) ) ;
#7720=CARTESIAN_POINT ( 'NONE',  ( 198.7165341137897485, 51.46663580899081580, -15.00000000000000178 ) ) ;
#7722=ORIENTED_EDGE ( 'NONE', *, *, #15580, .T. ) ;
#7725=CARTESIAN_POINT ( 'NONE',  ( 195.0000000000000000, 39.31328125216787583, -13.57481594606304576 ) ) ;
#7728=CARTESIAN_POINT ( 'NONE',  ( -8.049105076161786076E-16, 38.96601562608393721, -13.14518615778179544 ) ) ;
#7729=CARTESIAN_POINT ( 'NONE',  ( 13.14518615778179900, 32.26875000108393721, -5.444914386472297529 ) ) ;
#7731=CYLINDRICAL_SURFACE ( 'NONE', #19138, 11.57481594606304398 ) ;
#7732=AXIS2_PLACEMENT_3D ( 'NONE', #5294, #20547, #20250 ) ;
#7734=CARTESIAN_POINT ( 'NONE',  ( 0.000000000000000000, 50.00000000000000000, 0.000000000000000000 ) ) ;
#7737=ADVANCED_FACE ( 'NONE', ( #1902 ), #1483, .T. ) ;
#7738=CARTESIAN_POINT ( 'NONE',  ( 103.1528011352953342, 82.31250000136559208, -3.152801135295383084 ) ) ;
#7751=ORIENTED_EDGE ( 'NONE', *, *, #23185, .F. ) ;
#7753=CARTESIAN_POINT ( 'NONE',  ( 59.55508561352770158, 36.93203125108394147, 13.14518615778179722 ) ) ;
#7756=FACE_OUTER_BOUND ( 'NONE', #24433, .T. ) ;
#7760=CARTESIAN_POINT ( 'NONE',  ( 1.014130826074231884, 51.45790058219387930, -14.99999999999932321 ) ) ;
#7761=CARTESIAN_POINT ( 'NONE',  ( 201.0790800205188589, 54.65154858643461466, 14.99999999999994671 ) ) ;
#7762=CARTESIAN_POINT ( 'NONE',  ( 116.4251840539369454, 38.66835937716786731, -5.622872871577873077 ) ) ;
#7765=CARTESIAN_POINT ( 'NONE',  ( 208.1451861577817795, 38.81718750108393579, -5.444914386472297529 ) ) ;
#7768=AXIS2_PLACEMENT_3D ( 'NONE', #20115, #13384, #15534 ) ;
#7773=CARTESIAN_POINT ( 'NONE',  ( 55.70494972787295751, 32.11992187608393579, 9.295050272127047819 ) ) ;
#7778=CARTESIAN_POINT ( 'NONE',  ( 5.364947964714800399, 36.00000000000002842, 12.09311862596063492 ) ) ;
#7779=CARTESIAN_POINT ( 'NONE',  ( -15.00000000000000000, 55.00000000000000000, 10.00000000000000000 ) ) ;
#7780=CARTESIAN_POINT ( 'NONE',  ( 120.4011555911795455, 33.95546874999999432, 9.598844408820459861 ) ) ;
#7782=ORIENTED_EDGE ( 'NONE', *, *, #10011, .T. ) ;
#7783=DIRECTION ( 'NONE',  ( 1.000000000000000000, 0.000000000000000000, -2.385244779468110248E-16 ) ) ;
#7788=CARTESIAN_POINT ( 'NONE',  ( 116.8548138422182205, 40.75195312608393294, 0.000000000000000000 ) ) ;
#7789=CARTESIAN_POINT ( 'NONE',  ( 74.29505027212704249, 39.46210937608393010, -9.295050272127046043 ) ) ;
#7790=VECTOR ( 'NONE', #8028, 1000.000000000000000 ) ;
#7792=CARTESIAN_POINT ( 'NONE',  ( 60.21996080114833916, 35.99999999999998579, 12.25280873422828876 ) ) ;
#7793=CARTESIAN_POINT ( 'NONE',  ( -13.14518615778179900, 38.91640625108393436, -5.444914386472297529 ) ) ;
#7795=DIRECTION ( 'NONE',  ( 0.000000000000000000, 0.000000000000000000, -1.000000000000000000 ) ) ;
#7797=CARTESIAN_POINT ( 'NONE',  ( 195.0000000000000000, 40.40468749999999432, 13.57481594606304576 ) ) ;
#7799=CYLINDRICAL_SURFACE ( 'NONE', #17918, 13.57481594606304398 ) ;
#7802=CARTESIAN_POINT ( 'NONE',  ( 116.9040934463640156, 36.00000000000000000, 1.137167824541468031 ) ) ;
#7806=VERTEX_POINT ( 'NONE', #9007 ) ;
#7813=CARTESIAN_POINT ( 'NONE',  ( 99.99999999999995737, 80.68750000136559208, 4.458734124999988779 ) ) ;
#7814=CARTESIAN_POINT ( 'NONE',  ( 55.70494972787295751, 33.50898437608393010, 9.295050272127047819 ) ) ;
#7817=( BOUNDED_CURVE ( )  B_SPLINE_CURVE ( 2, ( #12422, #12006, #21140, #25133, #10286, #10016, #18994, #18724, #20731 ),
 .UNSPECIFIED., .F., .F. ) 
 B_SPLINE_CURVE_WITH_KNOTS ( ( 3, 2, 2, 2, 3 ),
 ( 0.06250000000000004163, 0.07291666666666665741, 0.08333333333333325932, 0.09374999999999987510, 0.1041666666666664909 ),
 .UNSPECIFIED. ) 
 CURVE ( )  GEOMETRIC_REPRESENTATION_ITEM ( )  RATIONAL_B_SPLINE_CURVE ( ( 0.9999999999999996669, 0.9238795325112870716, 1.000000000000000000, 0.9238795325112867385, 1.000000000000000000, 0.9238795325112867385, 1.000000000000000000, 0.9238795325112880708, 0.9999999999999986677 ) ) 
 REPRESENTATION_ITEM ( '' )  );
#7818=DIRECTION ( 'NONE',  ( 0.000000000000000000, 0.000000000000000000, -1.000000000000000000 ) ) ;
#7821=CARTESIAN_POINT ( 'NONE',  ( 124.5550856135277087, 35.34453125108393579, 13.14518615778179722 ) ) ;
#7823=CARTESIAN_POINT ( 'NONE',  ( 74.59884440882045453, 38.22187500216787015, 9.598844408820456309 ) ) ;
#7824=CARTESIAN_POINT ( 'NONE',  ( 95.54126587499996504, 82.43750000136559208, -1.387778780781445676E-14 ) ) ;
#7825=CARTESIAN_POINT ( 'NONE',  ( 116.8548138422182063, 40.50390625108394005, -5.444914386472297529 ) ) ;
#7826=CARTESIAN_POINT ( 'NONE',  ( 200.6228728715778686, 37.57695312499999574, -13.57481594606304753 ) ) ;
#7828=CARTESIAN_POINT ( 'NONE',  ( -9.598844408820458085, 39.41250000216787441, -9.598844408820458085 ) ) ;
#7829=ORIENTED_EDGE ( 'NONE', *, *, #19411, .T. ) ;
#7833=CARTESIAN_POINT ( 'NONE',  ( 208.1451861577818079, 39.36289062608393152, -1.609821015232357215E-15 ) ) ;
#7837=CARTESIAN_POINT ( 'NONE',  ( 143.1451861577818363, 37.03125000108393294, -5.444914386472297529 ) ) ;
#7838=CARTESIAN_POINT ( 'NONE',  ( 5.444914386472297529, 33.36015625108393579, -13.14518615778179900 ) ) ;
#7839=DIRECTION ( 'NONE',  ( -0.000000000000000000, 1.000000000000000000, -0.000000000000000000 ) ) ;
#7840=DIRECTION ( 'NONE',  ( 0.000000000000000000, 0.000000000000000000, -1.000000000000000000 ) ) ;
#7842=CARTESIAN_POINT ( 'NONE',  ( 185.4011555911795313, 40.10703124999999147, -9.598844408820458085 ) ) ;
#7852=CARTESIAN_POINT ( 'NONE',  ( -8.049105076161786076E-16, 34.20351562608394147, -13.14518615778179544 ) ) ;
#7854=CARTESIAN_POINT ( 'NONE',  ( 96.84719886470459471, 83.81250000136560629, 3.152801135295355994 ) ) ;
#7857=CARTESIAN_POINT ( 'NONE',  ( 185.7049497278729575, 33.50898437608393010, 9.295050272127047819 ) ) ;
#7858=EDGE_LOOP ( 'NONE', ( #5451, #25002, #23974, #2656 ) ) ;
#7861=EDGE_CURVE ( 'NONE', #13418, #11663, #20698, .T. ) ;
#7865=CARTESIAN_POINT ( 'NONE',  ( 219.9999999999999716, 80.00000000000000000, 9.999999999999946709 ) ) ;
#7867=CARTESIAN_POINT ( 'NONE',  ( 9.295050272127047819, 37.87460937608393863, 9.295050272127046043 ) ) ;
#7868=CARTESIAN_POINT ( 'NONE',  ( -9.295050272127044266, 33.50898437608393010, 9.295050272127047819 ) ) ;
#7870=CARTESIAN_POINT ( 'NONE',  ( 99.99999999999995737, 80.37500000273119838, 4.999999999999990230 ) ) ;
#7875=CARTESIAN_POINT ( 'NONE',  ( 98.15313185440923860, 82.87500000136560629, 4.458734124999987891 ) ) ;
#7877=CARTESIAN_POINT ( 'NONE',  ( 78.57481594606305464, 39.06523437716786873, 5.622872871577868636 ) ) ;
#7883=DIRECTION ( 'NONE',  ( -0.000000000000000000, 1.000000000000000000, -0.000000000000000000 ) ) ;
#7887=ORIENTED_EDGE ( 'NONE', *, *, #13135, .F. ) ;
#7888=CARTESIAN_POINT ( 'NONE',  ( 55.70494972787295751, 38.46992187608393721, 9.295050272127047819 ) ) ;
#7894=CARTESIAN_POINT ( 'NONE',  ( 65.00000000000000000, 37.62656249999999858, -13.57481594606304576 ) ) ;
#7896=CARTESIAN_POINT ( 'NONE',  ( 143.5748159460630688, 36.68398437716787441, 5.622872871577868636 ) ) ;
#7897=CARTESIAN_POINT ( 'NONE',  ( 143.5748159460630404, 35.98945312716787015, -5.622872871577873077 ) ) ;
#7898=ADVANCED_FACE ( 'NONE', ( #22268 ), #9282, .T. ) ;
#7900=LINE ( 'NONE', #21154, #4159 ) ;
#7901=CARTESIAN_POINT ( 'NONE',  ( 181.8548138422181921, 36.73359375108393010, -5.444914386472297529 ) ) ;
#7903=ORIENTED_EDGE ( 'NONE', *, *, #15621, .F. ) ;
#7906=CARTESIAN_POINT ( 'NONE',  ( -8.312177448680279460E-16, 38.42031249999999432, -13.57481594606304576 ) ) ;
#7907=DIRECTION ( 'NONE',  ( 0.000000000000000000, 0.000000000000000000, 1.000000000000000000 ) ) ;
#7908=LINE ( 'NONE', #1645, #14851 ) ;
#7910=DIRECTION ( 'NONE',  ( 0.000000000000000000, 0.000000000000000000, 1.000000000000000000 ) ) ;
#7912=CARTESIAN_POINT ( 'NONE',  ( 13.39333672780522733, 35.99999999999999289, -2.034633736483404398 ) ) ;
#7915=ORIENTED_EDGE ( 'NONE', *, *, #8104, .T. ) ;
#7916=ORIENTED_EDGE ( 'NONE', *, *, #22040, .F. ) ;
#7921=CARTESIAN_POINT ( 'NONE',  ( 120.7049497278729575, 40.65273437608393436, -9.295050272127046043 ) ) ;
#7922=CARTESIAN_POINT ( 'NONE',  ( 59.55508561352770158, 35.93984375108392726, 13.14518615778179722 ) ) ;
#7924=CARTESIAN_POINT ( 'NONE',  ( -5.444914386472297529, 35.64218750108392442, -13.14518615778179900 ) ) ;
#7928=DIRECTION ( 'NONE',  ( 0.000000000000000000, -1.000000000000000000, 0.000000000000000000 ) ) ;
#7929=CARTESIAN_POINT ( 'NONE',  ( 204.5988444088204687, 40.50390624999999289, 9.598844408820456309 ) ) ;
#7930=CARTESIAN_POINT ( 'NONE',  ( 5.444914386472302859, 37.62656250108393863, 13.14518615778179189 ) ) ;
#7931=CARTESIAN_POINT ( 'NONE',  ( 143.2454503467689619, 36.00000000000000000, 2.307131236160140375 ) ) ;
#7940=ORIENTED_EDGE ( 'NONE', *, *, #14668, .T. ) ;
#7943=LINE ( 'NONE', #21341, #5038 ) ;
#7944=EDGE_CURVE ( 'NONE', #16904, #10007, #11250, .T. ) ;
#7946=CARTESIAN_POINT ( 'NONE',  ( 101.8468681455906903, 81.75000000136560629, 4.458734124999987891 ) ) ;
#7947=CARTESIAN_POINT ( 'NONE',  ( 51.85481384221820633, 39.21406250108392300, 5.444914386472304635 ) ) ;
#7952=CARTESIAN_POINT ( 'NONE',  ( 143.1451861577818079, 34.05468750108394005, -5.444914386472297529 ) ) ;
#7954=CARTESIAN_POINT ( 'NONE',  ( -7.616525325480801634, 54.91574374957786375, -14.99999999999999822 ) ) ;
#7957=CARTESIAN_POINT ( 'NONE',  ( 120.7049497278729575, 38.27148437608393294, 9.295050272127047819 ) ) ;
#7958=CARTESIAN_POINT ( 'NONE',  ( 65.00000000000000000, 36.53515625216787299, 13.57481594606304576 ) ) ;
#7961=CARTESIAN_POINT ( 'NONE',  ( -5.622872871577873077, 38.07304687716787583, 13.57481594606304753 ) ) ;
#7964=ORIENTED_EDGE ( 'NONE', *, *, #13839, .T. ) ;
#7966=CARTESIAN_POINT ( 'NONE',  ( 189.3771271284221314, 31.72304687716787441, 13.57481594606304753 ) ) ;
#7967=CARTESIAN_POINT ( 'NONE',  ( 99.99999999999995737, 81.75000000000000000, -5.000000000000018652 ) ) ;
#7969=CARTESIAN_POINT ( 'NONE',  ( 116.8548138422182205, 37.37851562608393863, 0.000000000000000000 ) ) ;
#7970=CARTESIAN_POINT ( 'NONE',  ( 13.14518615778179900, 33.26093750108393721, -5.444914386472297529 ) ) ;
#7971=DIRECTION ( 'NONE',  ( 0.000000000000000000, -0.000000000000000000, 1.000000000000000000 ) ) ;
#7973=( BOUNDED_CURVE ( )  B_SPLINE_CURVE ( 2, ( #4731, #457, #9417, #13391, #26684, #3160, #11541, #9001, #22119 ),
 .UNSPECIFIED., .F., .F. ) 
 B_SPLINE_CURVE_WITH_KNOTS ( ( 3, 2, 2, 2, 3 ),
 ( 0.05000000000000004441, 0.07500000000000006661, 0.1000000000000000888, 0.1250000000000001110, 0.1500000000000001332 ),
 .UNSPECIFIED. ) 
 CURVE ( )  GEOMETRIC_REPRESENTATION_ITEM ( )  RATIONAL_B_SPLINE_CURVE ( ( 0.9999999999999998890, 0.9238795325112868495, 1.000000000000000000, 0.9238795325112867385, 1.000000000000000000, 0.9238795325112867385, 1.000000000000000000, 0.9238795325112862944, 1.000000000000000444 ) ) 
 REPRESENTATION_ITEM ( '' )  );
#7975=CARTESIAN_POINT ( 'NONE',  ( 200.6228728715778686, 37.27929687499999289, 13.57481594606304576 ) ) ;
#7976=CARTESIAN_POINT ( 'NONE',  ( 55.40115559117954547, 39.51171874999999289, 9.598844408820459861 ) ) ;
#7978=CARTESIAN_POINT ( 'NONE',  ( 70.44491438647230552, 39.21406250108392300, 13.14518615778179189 ) ) ;
#7984=CARTESIAN_POINT ( 'NONE',  ( 130.0000000000000000, 52.00000000000000711, 11.57481594606302799 ) ) ;
#7985=CARTESIAN_POINT ( 'NONE',  ( -9.598844408820454532, 40.30546874999999574, 9.598844408820459861 ) ) ;
#7987=CARTESIAN_POINT ( 'NONE',  ( 103.1528011352953342, 81.31250000136559208, -3.152801135295383084 ) ) ;
#7989=CIRCLE ( 'NONE', #23916, 13.57481594606304398 ) ;
#7991=VERTEX_POINT ( 'NONE', #26688 ) ;
#7993=CARTESIAN_POINT ( 'NONE',  ( 186.2306103279209140, 50.37710889402406877, -14.99999999999737454 ) ) ;
#7995=ORIENTED_EDGE ( 'NONE', *, *, #7861, .F. ) ;
#7998=CARTESIAN_POINT ( 'NONE',  ( 195.0000000000000000, 40.10703125216787157, -13.57481594606304576 ) ) ;
#8001=CARTESIAN_POINT ( 'NONE',  ( 130.0000000000000000, 40.15664062608393436, 13.14518615778179544 ) ) ;
#8002=CARTESIAN_POINT ( 'NONE',  ( -5.444914386472299306, 32.76484375108393010, 13.14518615778179722 ) ) ;
#8004=CARTESIAN_POINT ( 'NONE',  ( 55.40115559117954547, 38.71796874999999716, 9.598844408820459861 ) ) ;
#8005=CIRCLE ( 'NONE', #11630, 5.000000000000004441 ) ;
#8007=CARTESIAN_POINT ( 'NONE',  ( 1.662435489736055498E-15, 50.00000000000000000, -13.57481594606304398 ) ) ;
#8011=CARTESIAN_POINT ( 'NONE',  ( 95.54126587499996504, 83.68750000136560629, -1.387778780781445676E-14 ) ) ;
#8019=VECTOR ( 'NONE', #27074, 1000.000000000000000 ) ;
#8020=CARTESIAN_POINT ( 'NONE',  ( -20.00000000000000000, 55.00000000000000000, 10.00000000000000178 ) ) ;
#8021=FACE_OUTER_BOUND ( 'NONE', #18999, .T. ) ;
#8024=CARTESIAN_POINT ( 'NONE',  ( 1.662435489736055498E-15, -7.395377635281828788, -13.57481594606304398 ) ) ;
#8025=CIRCLE ( 'NONE', #18029, 13.57481594606304398 ) ;
#8026=EDGE_LOOP ( 'NONE', ( #8473, #9672, #28118, #18030, #22102, #4773, #20596, #7829, #5498, #14119, #26582, #5703, #15944, #10862, #26519, #2142, #15256 ) ) ;
#8027=CARTESIAN_POINT ( 'NONE',  ( 59.55508561352770158, 37.42812500108394147, -13.14518615778179722 ) ) ;
#8028=DIRECTION ( 'NONE',  ( -0.000000000000000000, 1.000000000000000000, -0.000000000000000000 ) ) ;
#8030=ORIENTED_EDGE ( 'NONE', *, *, #16988, .F. ) ;
#8032=CARTESIAN_POINT ( 'NONE',  ( -3.803054373244904696, 54.09082899096177499, -15.00000000000000000 ) ) ;
#8033=CARTESIAN_POINT ( 'NONE',  ( 196.5010191243050315, 53.60014735326985402, 14.99999999999994493 ) ) ;
#8034=CARTESIAN_POINT ( 'NONE',  ( 143.5748159460630688, 33.55859375216787299, -1.662435489736055892E-15 ) ) ;
#8037=DIRECTION ( 'NONE',  ( -1.000000000000000000, -6.938893903907235280E-16, 2.385244779468109755E-16 ) ) ;
#8038=CARTESIAN_POINT ( 'NONE',  ( 195.0000000000000000, 37.77539062608393294, 13.14518615778179544 ) ) ;
#8039=ORIENTED_EDGE ( 'NONE', *, *, #15218, .F. ) ;
#8045=CARTESIAN_POINT ( 'NONE',  ( 214.9999999999999716, 80.00000000000000000, 14.99999999999994493 ) ) ;
#8048=CARTESIAN_POINT ( 'NONE',  ( 139.1801758136479918, 50.00000000000000000, -10.00000000000000000 ) ) ;
#8050=DIRECTION ( 'NONE',  ( 0.000000000000000000, -1.000000000000000000, 0.000000000000000000 ) ) ;
#8056=VECTOR ( 'NONE', #4061, 1000.000000000000000 ) ;
#8058=CARTESIAN_POINT ( 'NONE',  ( 143.1451861577818079, 38.02343750108395426, -5.444914386472297529 ) ) ;
#8059=CARTESIAN_POINT ( 'NONE',  ( 74.29505027212704249, 35.49335937608393010, -9.295050272127046043 ) ) ;
#8061=CARTESIAN_POINT ( 'NONE',  ( -9.295050272127044266, 35.89023437608393152, 9.295050272127047819 ) ) ;
#8062=CARTESIAN_POINT ( 'NONE',  ( 190.0271122604904406, 36.00000000000000711, -12.48139679469847607 ) ) ;
#8065=DIRECTION ( 'NONE',  ( -1.000000000000000000, 0.000000000000000000, 0.000000000000000000 ) ) ;
#8066=DIRECTION ( 'NONE',  ( 0.000000000000000000, 0.000000000000000000, -1.000000000000000000 ) ) ;
#8067=CARTESIAN_POINT ( 'NONE',  ( -13.14518615778179544, 37.37851562608393863, 0.000000000000000000 ) ) ;
#8068=CARTESIAN_POINT ( 'NONE',  ( 133.3041185978226224, 35.99999999999998579, 12.77244747738241770 ) ) ;
#8082=CARTESIAN_POINT ( 'NONE',  ( 94.99999999999995737, 80.06250000000001421, 2.071067811865466624 ) ) ;
#8083=CARTESIAN_POINT ( 'NONE',  ( 96.84719886470459471, 80.56250000136559208, 3.152801135295355994 ) ) ;
#8084=CARTESIAN_POINT ( 'NONE',  ( 65.00000000000000000, 36.98164062608393721, 13.14518615778179544 ) ) ;
#8087=EDGE_CURVE ( 'NONE', #6724, #5473, #9993, .T. ) ;
#8091=CARTESIAN_POINT ( 'NONE',  ( 135.4449143864723055, 32.26875000108393721, 13.14518615778179189 ) ) ;
#8092=VERTEX_POINT ( 'NONE', #25239 ) ;
#8094=ADVANCED_FACE ( 'NONE', ( #5729 ), #25831, .T. ) ;
#8097=CARTESIAN_POINT ( 'NONE',  ( 130.0000000000000000, 38.37070312608393152, 13.14518615778179544 ) ) ;
#8098=CARTESIAN_POINT ( 'NONE',  ( 65.00000000000000000, 36.93203125216787441, -13.57481594606304576 ) ) ;
#8101=CARTESIAN_POINT ( 'NONE',  ( -13.57481594606304576, 35.54296875216788010, 0.000000000000000000 ) ) ;
#8104=EDGE_CURVE ( 'NONE', #23060, #19811, #15659, .T. ) ;
#8107=CARTESIAN_POINT ( 'NONE',  ( 185.7049497278729575, 38.86679687608393863, -9.295050272127046043 ) ) ;
#8109=CARTESIAN_POINT ( 'NONE',  ( 135.4449143864723339, 38.42031250108393436, 13.14518615778179189 ) ) ;
#8110=CARTESIAN_POINT ( 'NONE',  ( 13.14518615778179900, 33.16171875108393863, 5.444914386472293977 ) ) ;
#8111=CARTESIAN_POINT ( 'NONE',  ( 130.0000000000000000, 37.22968749999999716, 13.57481594606304576 ) ) ;
#8115=CARTESIAN_POINT ( 'NONE',  ( 185.4011555911795313, 38.51953124999999289, -9.598844408820458085 ) ) ;
#8116=EDGE_CURVE ( 'NONE', #2928, #12585, #20230, .T. ) ;
#8120=CARTESIAN_POINT ( 'NONE',  ( 74.29505027212704249, 40.25585937608393294, -9.295050272127046043 ) ) ;
#8125=CARTESIAN_POINT ( 'NONE',  ( 9.598844408820459861, 38.12265624999999858, 9.598844408820456309 ) ) ;
#8126=CARTESIAN_POINT ( 'NONE',  ( 143.1451861577818079, 40.40468750108393436, -5.444914386472297529 ) ) ;
#8128=CARTESIAN_POINT ( 'NONE',  ( 101.8468681455906903, 83.00000000136559208, 4.458734124999987891 ) ) ;
#8131=CYLINDRICAL_SURFACE ( 'NONE', #15664, 13.57481594606304398 ) ;
#8132=ORIENTED_EDGE ( 'NONE', *, *, #17385, .F. ) ;
#8135=VERTEX_POINT ( 'NONE', #12075 ) ;
#8136=CARTESIAN_POINT ( 'NONE',  ( 129.6752756888039926, 53.49346745874646558, -15.00000000000000355 ) ) ;
#8141=CARTESIAN_POINT ( 'NONE',  ( 189.3771271284221314, 37.77539062716788010, -13.57481594606304753 ) ) ;
#8144=CARTESIAN_POINT ( 'NONE',  ( 195.4460412567803189, 49.99999999978059151, 13.57776691409217484 ) ) ;
#8145=CARTESIAN_POINT ( 'NONE',  ( 135.4449143864723339, 38.61875000108392442, 13.14518615778179189 ) ) ;
#8146=CARTESIAN_POINT ( 'NONE',  ( 13.14518615778179900, 32.96328125108393436, 5.444914386472293977 ) ) ;
#8149=CARTESIAN_POINT ( 'NONE',  ( 51.42518405393695957, 37.77539062499999289, -5.622872871577873077 ) ) ;
#8151=CARTESIAN_POINT ( 'NONE',  ( 201.8311344573052111, 36.00000000000002842, 11.35217666745979770 ) ) ;
#8155=DIRECTION ( 'NONE',  ( 0.000000000000000000, -1.000000000000000000, 0.000000000000000000 ) ) ;
#8157=CARTESIAN_POINT ( 'NONE',  ( 5.444914386472297529, 40.50390625108394005, -13.14518615778179900 ) ) ;
#8158=EDGE_CURVE ( 'NONE', #3022, #861, #22822, .T. ) ;
#8169=CARTESIAN_POINT ( 'NONE',  ( 51.85481384221820633, 37.57695312608393579, 0.000000000000000000 ) ) ;
#8170=CARTESIAN_POINT ( 'NONE',  ( 94.99999999999995737, 83.06250000273119838, -2.071067811865491493 ) ) ;
#8171=CARTESIAN_POINT ( 'NONE',  ( 189.5550856135277229, 31.87187500108393223, -13.14518615778179900 ) ) ;
#8174=CARTESIAN_POINT ( 'NONE',  ( -9.180175813648009608, 49.99999999999997868, -14.99999999999999822 ) ) ;
#8177=CARTESIAN_POINT ( 'NONE',  ( 120.4011555911795455, 34.65000000216787868, -9.598844408820458085 ) ) ;
#8178=CARTESIAN_POINT ( 'NONE',  ( 51.85481384221820633, 39.16445312608393436, 0.000000000000000000 ) ) ;
#8180=CARTESIAN_POINT ( 'NONE',  ( 195.0000000000000000, 38.56914062608393579, 13.14518615778179544 ) ) ;
#8181=ORIENTED_EDGE ( 'NONE', *, *, #430, .F. ) ;
#8184=CARTESIAN_POINT ( 'NONE',  ( 94.99999999999995737, 84.06250000000002842, 2.071067811865466624 ) ) ;
#8185=CARTESIAN_POINT ( 'NONE',  ( 13.57481594606304753, 39.85898437499999858, -5.622872871577873966 ) ) ;
#8190=CARTESIAN_POINT ( 'NONE',  ( 3.304118597821753767, 35.99999999999998579, 12.77244747738262554 ) ) ;
#8192=CARTESIAN_POINT ( 'NONE',  ( 124.3771271284221314, 32.41757812499999858, 13.57481594606304753 ) ) ;
#8197=CARTESIAN_POINT ( 'NONE',  ( 116.8548138422182205, 39.95820312608393010, 0.000000000000000000 ) ) ;
#8198=CARTESIAN_POINT ( 'NONE',  ( 70.44491438647230552, 37.62656250108393863, 13.14518615778179189 ) ) ;
#8199=CARTESIAN_POINT ( 'NONE',  ( 189.5550856135277229, 31.97109375108393436, 13.14518615778179722 ) ) ;
#8200=FACE_OUTER_BOUND ( 'NONE', #11171, .T. ) ;
#8201=CARTESIAN_POINT ( 'NONE',  ( 2.414731522848535132E-15, 35.19570312608392726, 13.14518615778179544 ) ) ;
#8202=CARTESIAN_POINT ( 'NONE',  ( 199.1572863549628210, 35.99999999999999289, -12.92256159328821141 ) ) ;
#8203=DIRECTION ( 'NONE',  ( -0.000000000000000000, 1.000000000000000000, -0.000000000000000000 ) ) ;
#8204=CARTESIAN_POINT ( 'NONE',  ( 195.0000000000000000, -7.395377635281828788, 11.57481594606302266 ) ) ;
#8205=ADVANCED_FACE ( 'NONE', ( #16653 ), #5560, .T. ) ;
#8206=VERTEX_POINT ( 'NONE', #18660 ) ;
#8207=CARTESIAN_POINT ( 'NONE',  ( -13.14518615778179544, 38.17226562608393436, 0.000000000000000000 ) ) ;
#8208=CARTESIAN_POINT ( 'NONE',  ( 0.7197605961091595450, 53.51499872091925170, 14.99999999999999645 ) ) ;
#8214=EDGE_LOOP ( 'NONE', ( #13599, #2978, #2528, #13989 ) ) ;
#8220=CARTESIAN_POINT ( 'NONE',  ( 104.4587341249999781, 81.00000000136560629, -1.846868145590750299 ) ) ;
#8221=CARTESIAN_POINT ( 'NONE',  ( 51.85481384221819923, 39.11484375108394573, -5.444914386472297529 ) ) ;
#8225=CARTESIAN_POINT ( 'NONE',  ( 143.5748159460630688, 39.06523437499999574, -5.622872871577873966 ) ) ;
#8227=CARTESIAN_POINT ( 'NONE',  ( 116.4251840539369596, 39.46210937499999005, 5.622872871577880183 ) ) ;
#8229=CARTESIAN_POINT ( 'NONE',  ( 7.623941961925452482, 55.00000000000001421, -15.00000000000000000 ) ) ;
#8231=CARTESIAN_POINT ( 'NONE',  ( 98.15313185440925281, 79.62500000136560629, 4.458734124999987891 ) ) ;
#8233=CARTESIAN_POINT ( 'NONE',  ( 70.62287287157786864, 38.46992187716787015, -13.57481594606304753 ) ) ;
#8236=CARTESIAN_POINT ( 'NONE',  ( 13.57481594606304753, 35.19570312716788152, -5.622872871577873077 ) ) ;
#8237=EDGE_LOOP ( 'NONE', ( #13369, #40, #1747, #26526 ) ) ;
#8240=CARTESIAN_POINT ( 'NONE',  ( 208.1451861577817795, 36.13828125108393863, 5.444914386472293977 ) ) ;
#8243=CARTESIAN_POINT ( 'NONE',  ( 143.1451861577818363, 39.41250000108393436, -5.444914386472297529 ) ) ;
#8250=CARTESIAN_POINT ( 'NONE',  ( 181.4251840539369596, 37.87460937499999147, 5.622872871577880183 ) ) ;
#8254=CARTESIAN_POINT ( 'NONE',  ( 78.14518615778179367, 39.36289062608393152, -1.609821015232357215E-15 ) ) ;
#8256=CARTESIAN_POINT ( 'NONE',  ( 0.000000000000000000, 78.00000000000000000, 0.000000000000000000 ) ) ;
#8259=CARTESIAN_POINT ( 'NONE',  ( -13.57481594606304576, 39.46210937499999005, 5.622872871577880183 ) ) ;
#8260=CARTESIAN_POINT ( 'NONE',  ( 116.8548138422182063, 39.90859375108394147, -5.444914386472297529 ) ) ;
#8261=EDGE_CURVE ( 'NONE', #11873, #8652, #18008, .T. ) ;
#8262=VERTEX_POINT ( 'NONE', #25487 ) ;
#8263=CARTESIAN_POINT ( 'NONE',  ( 98.15313185440925281, 82.87500000136560629, 4.458734124999987891 ) ) ;
#8266=CARTESIAN_POINT ( 'NONE',  ( -20.00000000000000355, 55.00000000000000000, -9.999999999999998224 ) ) ;
#8267=CARTESIAN_POINT ( 'NONE',  ( 51.85481384221820633, 33.65781250108393152, 5.444914386472304635 ) ) ;
#8273=CARTESIAN_POINT ( 'NONE',  ( 208.5748159460630120, 36.68398437716788152, 5.622872871577869525 ) ) ;
#8274=EDGE_CURVE ( 'NONE', #19327, #20134, #21386, .T. ) ;
#8277=CARTESIAN_POINT ( 'NONE',  ( 203.3959387412915873, 54.99999999495823744, 14.99999999999994671 ) ) ;
#8278=CARTESIAN_POINT ( 'NONE',  ( 143.1451861577818363, 39.61093750108393863, -5.444914386472297529 ) ) ;
#8279=CARTESIAN_POINT ( 'NONE',  ( -5.444914386472297529, 39.80937500108392868, -13.14518615778179900 ) ) ;
#8281=CARTESIAN_POINT ( 'NONE',  ( 55.40115559117954547, 36.93203124999999432, -9.598844408820458085 ) ) ;
#8284=CARTESIAN_POINT ( 'NONE',  ( 97.92893218813449607, 83.93750000273119838, -5.000000000000020428 ) ) ;
#8288=CARTESIAN_POINT ( 'NONE',  ( 104.4587341249999781, 80.25000000136559208, -1.846868145590750521 ) ) ;
#8290=CARTESIAN_POINT ( 'NONE',  ( -13.14518615778179900, 38.32109375108394289, -5.444914386472297529 ) ) ;
#8295=( BOUNDED_CURVE ( )  B_SPLINE_CURVE ( 2, ( #26708, #22142, #2622, #16707, #25257, #5748, #22716, #20717, #14415 ),
 .UNSPECIFIED., .F., .T. ) 
 B_SPLINE_CURVE_WITH_KNOTS ( ( 3, 2, 2, 2, 3 ),
 ( 0.2708333333333330928, 0.2812499999999998890, 0.2916666666666666852, 0.3020833333333334259, 0.3125000000000002220 ),
 .UNSPECIFIED. ) 
 CURVE ( )  GEOMETRIC_REPRESENTATION_ITEM ( )  RATIONAL_B_SPLINE_CURVE ( ( 1.000000000000001554, 0.9238795325112850731, 1.000000000000000000, 0.9238795325112867385, 1.000000000000000000, 0.9238795325112867385, 1.000000000000000000, 0.9238795325112850731, 1.000000000000001554 ) ) 
 REPRESENTATION_ITEM ( '' )  );
#8298=CARTESIAN_POINT ( 'NONE',  ( 99.99999999999995737, 80.37500000273119838, 4.999999999999990230 ) ) ;
#8302=CARTESIAN_POINT ( 'NONE',  ( 59.55508561352770158, 38.51953125108393294, 13.14518615778179722 ) ) ;
#8303=CARTESIAN_POINT ( 'NONE',  ( 99.99999999999995737, 82.87500000273119838, -5.000000000000018652 ) ) ;
#8304=CARTESIAN_POINT ( 'NONE',  ( 185.7049497278729575, 32.11992187608393579, 9.295050272127047819 ) ) ;
#8305=ORIENTED_EDGE ( 'NONE', *, *, #4038, .T. ) ;
#8307=CARTESIAN_POINT ( 'NONE',  ( -4.504887086316538891, 51.44650206076907040, -14.99999999999999645 ) ) ;
#8310=CARTESIAN_POINT ( 'NONE',  ( 130.0000000000000000, 34.94765625216787441, 13.57481594606304576 ) ) ;
#8311=CARTESIAN_POINT ( 'NONE',  ( 104.9999999999999716, 81.62500000273119838, -1.449011120738813565E-14 ) ) ;
#8314=CARTESIAN_POINT ( 'NONE',  ( 208.1451861577817795, 34.74921875108395142, 5.444914386472293977 ) ) ;
#8315=ORIENTED_EDGE ( 'NONE', *, *, #5147, .T. ) ;
#8316=ORIENTED_EDGE ( 'NONE', *, *, #769, .F. ) ;
#8323=CARTESIAN_POINT ( 'NONE',  ( 96.84719886470459471, 83.56250000136560629, 3.152801135295355994 ) ) ;
#8327=DIRECTION ( 'NONE',  ( 0.000000000000000000, 0.000000000000000000, -1.000000000000000000 ) ) ;
#8328=FACE_OUTER_BOUND ( 'NONE', #13622, .T. ) ;
#8336=CARTESIAN_POINT ( 'NONE',  ( 139.2950502721270425, 35.69179687608394147, -9.295050272127046043 ) ) ;
#8337=CARTESIAN_POINT ( 'NONE',  ( 51.85481384221820633, 37.42812500108393436, 5.444914386472304635 ) ) ;
#8338=CARTESIAN_POINT ( 'NONE',  ( 200.4449143864723055, 38.91640625108393436, -13.14518615778179900 ) ) ;
#8339=CARTESIAN_POINT ( 'NONE',  ( 54.21315323181566015, 35.99999999999999289, 7.561388982944276194 ) ) ;
#8340=CARTESIAN_POINT ( 'NONE',  ( 13.14518615778179544, 35.39414062608393152, -1.609821015232357215E-15 ) ) ;
#8341=CARTESIAN_POINT ( 'NONE',  ( 137.1154903918550758, 49.99999999945652718, -11.58166858714055003 ) ) ;
#8342=CARTESIAN_POINT ( 'NONE',  ( 196.1371678245420753, 35.99999999999999289, 13.09590655363592582 ) ) ;
#8345=CARTESIAN_POINT ( 'NONE',  ( -8.049105076161786076E-16, 37.97382812608393721, -13.14518615778179544 ) ) ;
#8346=CARTESIAN_POINT ( 'NONE',  ( -3.116592080465746761, 53.90895096933311237, 14.99999999999999645 ) ) ;
#8349=CARTESIAN_POINT ( 'NONE',  ( 195.0000000000000000, 37.32890625216786873, 13.57481594606304576 ) ) ;
#8359=CARTESIAN_POINT ( 'NONE',  ( 104.4587341249999639, 79.93750000136559208, -1.442382525525748735E-14 ) ) ;
#8360=CARTESIAN_POINT ( 'NONE',  ( 78.14518615778179367, 38.02343750108395426, -5.444914386472297529 ) ) ;
#8365=PLANE ( 'NONE',  #27271 ) ;
#8367=CARTESIAN_POINT ( 'NONE',  ( 136.9444236247691151, 31.75150628229955529, -11.16113343896966370 ) ) ;
#8372=CARTESIAN_POINT ( 'NONE',  ( 104.4587341249999781, 80.87500000136560629, 1.846868145590721655 ) ) ;
#8374=CARTESIAN_POINT ( 'NONE',  ( 51.42518405393695957, 35.59257812716788294, 5.622872871577880183 ) ) ;
#8376=CARTESIAN_POINT ( 'NONE',  ( 13.57481594606304753, 34.40195312716787157, -5.622872871577873077 ) ) ;
#8377=EDGE_LOOP ( 'NONE', ( #3418, #26870, #2883, #14718 ) ) ;
#8380=CARTESIAN_POINT ( 'NONE',  ( 195.0000000000000000, 37.57695312608392868, 13.14518615778179544 ) ) ;
#8383=CARTESIAN_POINT ( 'NONE',  ( 143.1451861577818363, 37.82500000108392868, -5.444914386472297529 ) ) ;
#8385=DIRECTION ( 'NONE',  ( -1.000000000000000000, 0.000000000000000000, 2.385244779468110248E-16 ) ) ;
#8388=CARTESIAN_POINT ( 'NONE',  ( 208.5748159460630120, 38.96601562499999005, 5.622872871577869525 ) ) ;
#8389=CARTESIAN_POINT ( 'NONE',  ( 55.40115559117954547, 39.31328124999999574, -9.598844408820458085 ) ) ;
#8391=CARTESIAN_POINT ( 'NONE',  ( 70.44491438647230552, 38.71796875108393721, -13.14518615778179900 ) ) ;
#8393=FACE_OUTER_BOUND ( 'NONE', #10714, .T. ) ;
#8396=CARTESIAN_POINT ( 'NONE',  ( 2.493653234604083739E-15, 38.81718749999999574, 13.57481594606304576 ) ) ;
#8397=CARTESIAN_POINT ( 'NONE',  ( 120.7049497278729575, 39.85898437608393152, -9.295050272127046043 ) ) ;
#8399=CARTESIAN_POINT ( 'NONE',  ( 95.54126587499995082, 81.75000000136560629, 1.846868145590724986 ) ) ;
#8404=CARTESIAN_POINT ( 'NONE',  ( 65.00000000000000000, 35.79101562608394005, -13.14518615778179544 ) ) ;
#8411=CARTESIAN_POINT ( 'NONE',  ( 204.5988444088204403, 38.42031250216787441, -9.598844408820458085 ) ) ;
#8413=CARTESIAN_POINT ( 'NONE',  ( 199.5048870863314505, 51.44650206076381238, 14.99999999999995381 ) ) ;
#8414=CARTESIAN_POINT ( 'NONE',  ( 143.1451861577818363, 39.51171875108393294, 5.444914386472293977 ) ) ;
#8415=CARTESIAN_POINT ( 'NONE',  ( 9.295050272127046043, 38.86679687608393863, -9.295050272127046043 ) ) ;
#8417=VERTEX_POINT ( 'NONE', #15473 ) ;
#8418=CARTESIAN_POINT ( 'NONE',  ( 120.7049497278729575, 34.10429687608393579, -9.295050272127046043 ) ) ;
#8419=CARTESIAN_POINT ( 'NONE',  ( 51.42518405393695957, 38.66835937499999432, 5.622872871577880183 ) ) ;
#8427=VECTOR ( 'NONE', #14609, 1000.000000000000000 ) ;
#8430=CARTESIAN_POINT ( 'NONE',  ( -13.14518615778179544, 38.37070312608393152, 0.000000000000000000 ) ) ;
#8432=EDGE_LOOP ( 'NONE', ( #22714, #14124, #25207, #4537, #6695 ) ) ;
#8434=DIRECTION ( 'NONE',  ( -1.000000000000000000, 0.000000000000000000, 2.385244779468110248E-16 ) ) ;
#8435=EDGE_CURVE ( 'NONE', #1369, #15719, #24188, .T. ) ;
#8439=ADVANCED_FACE ( 'NONE', ( #19206 ), #27908, .T. ) ;
#8441=CARTESIAN_POINT ( 'NONE',  ( 189.5550856135277229, 39.11484375108394573, 13.14518615778179722 ) ) ;
#8444=EDGE_CURVE ( 'NONE', #13216, #8588, #10915, .T. ) ;
#8445=CARTESIAN_POINT ( 'NONE',  ( 96.46446609406721961, 83.00000000273119838, -3.535533905932755072 ) ) ;
#8446=CARTESIAN_POINT ( 'NONE',  ( 55.81982418635200816, 55.00000000000000000, -14.99999999999999822 ) ) ;
#8447=ORIENTED_EDGE ( 'NONE', *, *, #10719, .T. ) ;
#8450=CIRCLE ( 'NONE', #12083, 13.57481594606304398 ) ;
#8453=CARTESIAN_POINT ( 'NONE',  ( 135.6228728715778971, 35.79101562716787299, 13.57481594606304576 ) ) ;
#8456=CARTESIAN_POINT ( 'NONE',  ( 195.0000000000000000, 35.79101562608394005, -13.14518615778179544 ) ) ;
#8457=ORIENTED_EDGE ( 'NONE', *, *, #84, .T. ) ;
#8461=DIRECTION ( 'NONE',  ( -0.000000000000000000, 1.000000000000000000, -0.000000000000000000 ) ) ;
#8462=( BOUNDED_CURVE ( )  B_SPLINE_CURVE ( 2, ( #24541, #9423, #5025, #11690, #13691, #18122, #9713, #26836, #1040 ),
 .UNSPECIFIED., .F., .T. ) 
 B_SPLINE_CURVE_WITH_KNOTS ( ( 3, 2, 2, 2, 3 ),
 ( 0.4791666666666667962, 0.4895833333333333703, 0.5000000000000000000, 0.5104166666666665186, 0.5208333333333332593 ),
 .UNSPECIFIED. ) 
 CURVE ( )  GEOMETRIC_REPRESENTATION_ITEM ( )  RATIONAL_B_SPLINE_CURVE ( ( 0.9999999999999992228, 0.9238795325112875156, 1.000000000000000000, 0.9238795325112867385, 1.000000000000000000, 0.9238795325112867385, 1.000000000000000000, 0.9238795325112875156, 0.9999999999999992228 ) ) 
 REPRESENTATION_ITEM ( '' )  );
#8464=EDGE_CURVE ( 'NONE', #3050, #2793, #10637, .T. ) ;
#8465=CARTESIAN_POINT ( 'NONE',  ( 98.15313185440923860, 80.62500000136559208, 4.458734124999987891 ) ) ;
#8466=CARTESIAN_POINT ( 'NONE',  ( 181.8548138422182205, 38.96601562608393721, 0.000000000000000000 ) ) ;
#8470=DIRECTION ( 'NONE',  ( 0.000000000000000000, 0.000000000000000000, -1.000000000000000000 ) ) ;
#8471=CARTESIAN_POINT ( 'NONE',  ( 200.4449143864723055, 39.71015625108393010, -13.14518615778179722 ) ) ;
#8473=ORIENTED_EDGE ( 'NONE', *, *, #16314, .T. ) ;
#8478=CARTESIAN_POINT ( 'NONE',  ( 139.2950502721270425, 37.87460937608393863, 9.295050272127046043 ) ) ;
#8479=CARTESIAN_POINT ( 'NONE',  ( 51.85481384221820633, 38.17226562608393436, 0.000000000000000000 ) ) ;
#8480=B_SPLINE_CURVE_WITH_KNOTS ( 'NONE', 3,
 ( #6005, #23805, #6417, #25798, #1598, #27671, #12940, #8136, #4283, #12808, #16830, #10675, #25526, #10400, #27814, #10812, #8693, #14951 ),
 .UNSPECIFIED., .F., .F.,
 ( 4, 2, 2, 2, 2, 2, 2, 2, 4 ),
 ( 0.000000000000000000, 0.004618502246277096830, 0.006927753369415644812, 0.009237004492554193660, 0.01039163005412350842, 0.01154625561569282317, 0.01385550673883145616, 0.01616475786197005271, 0.01847400898510864406 ),
 .UNSPECIFIED. ) ;
#8482=CARTESIAN_POINT ( 'NONE',  ( 208.1451861577817795, 39.61093750108393863, -5.444914386472297529 ) ) ;
#8484=CARTESIAN_POINT ( 'NONE',  ( -5.444914386472299306, 35.14609375108393152, 13.14518615778179722 ) ) ;
#8485=CARTESIAN_POINT ( 'NONE',  ( 138.2113140151611788, 50.68678854790365307, -15.00000000000138201 ) ) ;
#8486=CIRCLE ( 'NONE', #20342, 5.000000000000000000 ) ;
#8489=CARTESIAN_POINT ( 'NONE',  ( 13.14518615778179544, 39.36289062608393152, -1.609821015232357215E-15 ) ) ;
#8491=CIRCLE ( 'NONE', #23083, 13.57481594606304398 ) ;
#8492=CARTESIAN_POINT ( 'NONE',  ( 63.39746686938465814, 53.60343507248209249, 14.99999999999997868 ) ) ;
#8496=CARTESIAN_POINT ( 'NONE',  ( 78.49550141231718214, 36.00000000000000711, -0.9550757908087965653 ) ) ;
#8497=ORIENTED_EDGE ( 'NONE', *, *, #26923, .T. ) ;
#8498=DIRECTION ( 'NONE',  ( 0.000000000000000000, 0.000000000000000000, 1.000000000000000000 ) ) ;
#8500=CARTESIAN_POINT ( 'NONE',  ( 65.00000000000000000, 38.12265625216787157, 13.57481594606304576 ) ) ;
#8502=DIRECTION ( 'NONE',  ( 0.000000000000000000, 0.000000000000000000, 1.000000000000000000 ) ) ;
#8503=CARTESIAN_POINT ( 'NONE',  ( 104.4587341249999781, 80.12500000136560629, 1.846868145590721655 ) ) ;
#8504=CARTESIAN_POINT ( 'NONE',  ( 78.14518615778179367, 37.97382812608393721, -1.609821015232357215E-15 ) ) ;
#8506=CARTESIAN_POINT ( 'NONE',  ( -13.14518615778179544, 39.75976562608393294, 0.000000000000000000 ) ) ;
#8507=CIRCLE ( 'NONE', #28087, 5.000000000000000000 ) ;
#8508=EDGE_LOOP ( 'NONE', ( #26743, #1737, #26131, #19562 ) ) ;
#8509=DIRECTION ( 'NONE',  ( -1.000000000000000000, 0.000000000000000000, 0.000000000000000000 ) ) ;
#8512=CARTESIAN_POINT ( 'NONE',  ( 120.7049497278729575, 32.11992187608393579, 9.295050272127047819 ) ) ;
#8516=CARTESIAN_POINT ( 'NONE',  ( 95.54126587499995082, 79.50000000136560629, 1.846868145590724986 ) ) ;
#8517=CARTESIAN_POINT ( 'NONE',  ( 116.8548138422182205, 37.37851562608393863, 0.000000000000000000 ) ) ;
#8518=CARTESIAN_POINT ( 'NONE',  ( 55.40115559117954547, 38.61875000216787157, -9.598844408820458085 ) ) ;
#8520=CARTESIAN_POINT ( 'NONE',  ( 2.493653234604083739E-15, 36.53515625216787299, 13.57481594606304576 ) ) ;
#8523=CARTESIAN_POINT ( 'NONE',  ( 200.4449143864723055, 37.13046875108393152, -13.14518615778179900 ) ) ;
#8524=AXIS2_PLACEMENT_3D ( 'NONE', #19179, #5806, #18896 ) ;
#8526=FACE_OUTER_BOUND ( 'NONE', #22463, .T. ) ;
#8533=CARTESIAN_POINT ( 'NONE',  ( 181.4251840539369596, 38.61874999999999147, 0.000000000000000000 ) ) ;
#8534=CARTESIAN_POINT ( 'NONE',  ( 59.37712712842205320, 40.05742187499998863, -13.57481594606297293 ) ) ;
#8536=CARTESIAN_POINT ( 'NONE',  ( 59.55508561352770158, 38.32109375108394289, 13.14518615778179722 ) ) ;
#8540=CARTESIAN_POINT ( 'NONE',  ( 55.81982418635200105, 50.00000000000000000, 9.999999999999982236 ) ) ;
#8541=CARTESIAN_POINT ( 'NONE',  ( -9.598844408820458085, 39.31328124999999574, -9.598844408820458085 ) ) ;
#8542=CARTESIAN_POINT ( 'NONE',  ( 130.0000000000000000, 39.36289062608393152, 13.14518615778179544 ) ) ;
#8544=CARTESIAN_POINT ( 'NONE',  ( 103.5355339059327093, 82.62500000000000000, -3.535533905932755072 ) ) ;
#8548=CARTESIAN_POINT ( 'NONE',  ( 70.44491438647230552, 33.36015625108393579, -13.14518615778179900 ) ) ;
#8549=ORIENTED_EDGE ( 'NONE', *, *, #11558, .T. ) ;
#8556=CARTESIAN_POINT ( 'NONE',  ( 195.0000000000000000, 36.13828125216787157, -13.57481594606304576 ) ) ;
#8559=CARTESIAN_POINT ( 'NONE',  ( 195.7238719380222562, 53.51529642094860861, 14.99999999999994671 ) ) ;
#8560=CARTESIAN_POINT ( 'NONE',  ( 120.7049497278729575, 38.46992187608393721, 9.295050272127047819 ) ) ;
#8562=CARTESIAN_POINT ( 'NONE',  ( -5.444914386472297529, 38.22187500108393010, -13.14518615778179900 ) ) ;
#8564=CARTESIAN_POINT ( 'NONE',  ( 116.8548138422182063, 35.84062500108394289, 5.444914386472304635 ) ) ;
#8565=CARTESIAN_POINT ( 'NONE',  ( 59.37712712842213136, 38.46992187499999716, -13.57481594606304753 ) ) ;
#8566=VECTOR ( 'NONE', #19751, 1000.000000000000000 ) ;
#8572=CARTESIAN_POINT ( 'NONE',  ( 13.57481594606304931, 39.06523437716786873, 5.622872871577868636 ) ) ;
#8573=CARTESIAN_POINT ( 'NONE',  ( 98.15313185440923860, 80.87500000136560629, 4.458734124999987891 ) ) ;
#8575=CARTESIAN_POINT ( 'NONE',  ( -5.444914386472297529, 39.80937500108392868, -13.14518615778179900 ) ) ;
#8577=ORIENTED_EDGE ( 'NONE', *, *, #18586, .F. ) ;
#8580=DIRECTION ( 'NONE',  ( 1.000000000000000000, -0.000000000000000000, -7.228014483236696740E-18 ) ) ;
#8582=CARTESIAN_POINT ( 'NONE',  ( 185.7049497278729575, 38.07304687608393579, -9.295050272127046043 ) ) ;
#8583=ORIENTED_EDGE ( 'NONE', *, *, #27226, .T. ) ;
#8586=AXIS2_PLACEMENT_3D ( 'NONE', #7779, #1241, #10458 ) ;
#8587=CARTESIAN_POINT ( 'NONE',  ( 143.5748159460630688, 39.80937499999999574, -1.662435489736055892E-15 ) ) ;
#8588=VERTEX_POINT ( 'NONE', #5376 ) ;
#8590=CARTESIAN_POINT ( 'NONE',  ( 124.3771271284221314, 37.67617187499999432, -13.57481594606304753 ) ) ;
#8592=CARTESIAN_POINT ( 'NONE',  ( 116.4251840539369596, 31.57421875216786944, 0.000000000000000000 ) ) ;
#8594=( BOUNDED_CURVE ( )  B_SPLINE_CURVE ( 2, ( #6803, #19925, #17636, #24631, #4682, #26195, #13198, #408, #2959 ),
 .UNSPECIFIED., .F., .T. ) 
 B_SPLINE_CURVE_WITH_KNOTS ( ( 3, 2, 2, 2, 3 ),
 ( 0.06250000000000004163, 0.07291666666666665741, 0.08333333333333325932, 0.09374999999999987510, 0.1041666666666664909 ),
 .UNSPECIFIED. ) 
 CURVE ( )  GEOMETRIC_REPRESENTATION_ITEM ( )  RATIONAL_B_SPLINE_CURVE ( ( 0.9999999999999996669, 0.9238795325112870716, 1.000000000000000000, 0.9238795325112867385, 1.000000000000000000, 0.9238795325112867385, 1.000000000000000000, 0.9238795325112880708, 0.9999999999999986677 ) ) 
 REPRESENTATION_ITEM ( '' )  );
#8595=CARTESIAN_POINT ( 'NONE',  ( 51.85481384221819923, 40.70234375108393721, -5.444914386472297529 ) ) ;
#8598=CARTESIAN_POINT ( 'NONE',  ( 204.2950502721270425, 34.89804687608393863, -9.295050272127046043 ) ) ;
#8599=EDGE_LOOP ( 'NONE', ( #13688, #13326 ) ) ;
#8601=EDGE_LOOP ( 'NONE', ( #4018, #12572, #17379, #9608 ) ) ;
#8604=CARTESIAN_POINT ( 'NONE',  ( 59.55508561352770158, 40.40468750108393436, -13.14518615778179722 ) ) ;
#8605=CARTESIAN_POINT ( 'NONE',  ( 51.42518405393695957, 36.33671875216787583, 0.000000000000000000 ) ) ;
#8606=CARTESIAN_POINT ( 'NONE',  ( 204.2950502721270425, 39.26367187608393294, 9.295050272127046043 ) ) ;
#8611=FACE_OUTER_BOUND ( 'NONE', #10738, .T. ) ;
#8618=CARTESIAN_POINT ( 'NONE',  ( 130.0000000000000000, 36.98164062608393721, 13.14518615778179544 ) ) ;
#8619=CARTESIAN_POINT ( 'NONE',  ( 55.70494972787295751, 32.51679687608393721, -9.295050272127046043 ) ) ;
#8620=CARTESIAN_POINT ( 'NONE',  ( 195.0000000000000000, 38.56914062608393579, 13.14518615778179544 ) ) ;
#8621=CARTESIAN_POINT ( 'NONE',  ( 63.97819628124013036, 36.00000000000001421, 13.11239906893439233 ) ) ;
#8622=CARTESIAN_POINT ( 'NONE',  ( 13.14518615778179544, 33.01289062608393010, -1.609821015232357215E-15 ) ) ;
#8624=CARTESIAN_POINT ( 'NONE',  ( 190.6259778691825204, 36.00000000000002132, 12.40367315690597749 ) ) ;
#8625=ADVANCED_FACE ( 'NONE', ( #3094, #5092, #6929, #7350, #13754 ), #22193, .F. ) ;
#8628=CARTESIAN_POINT ( 'NONE',  ( -9.295050272127046043, 34.10429687608393579, -9.295050272127046043 ) ) ;
#8630=DIRECTION ( 'NONE',  ( 0.000000000000000000, -1.000000000000000000, 0.000000000000000000 ) ) ;
#8631=CARTESIAN_POINT ( 'NONE',  ( 103.5355339059327093, 79.75000000273119838, -3.535533905932755072 ) ) ;
#8633=ADVANCED_FACE ( 'NONE', ( #11614 ), #11334, .F. ) ;
#8635=CARTESIAN_POINT ( 'NONE',  ( 0.000000000000000000, 0.000000000000000000, 0.000000000000000000 ) ) ;
#8640=CARTESIAN_POINT ( 'NONE',  ( 59.37712712842203189, 37.77539062716787299, -13.57481594606295339 ) ) ;
#8641=EDGE_CURVE ( 'NONE', #6724, #19008, #16189, .T. ) ;
#8642=VECTOR ( 'NONE', #13282, 1000.000000000000000 ) ;
#8644=CARTESIAN_POINT ( 'NONE',  ( -8.312177448680279460E-16, 36.93203125216787441, -13.57481594606304576 ) ) ;
#8645=CARTESIAN_POINT ( 'NONE',  ( 104.4587341249999781, 83.25000000136560629, -1.846868145590750299 ) ) ;
#8646=CARTESIAN_POINT ( 'NONE',  ( 65.00000000000000000, 36.58476562608393579, -13.14518615778179544 ) ) ;
#8648=CARTESIAN_POINT ( 'NONE',  ( -13.14518615778179544, 40.55351562608393579, 0.000000000000000000 ) ) ;
#8650=CARTESIAN_POINT ( 'NONE',  ( 103.5355339059327093, 80.75000000273119838, -3.535533905932755072 ) ) ;
#8651=CARTESIAN_POINT ( 'NONE',  ( 139.2950502721270425, 32.31835937608393294, 9.295050272127046043 ) ) ;
#8652=VERTEX_POINT ( 'NONE', #26620 ) ;
#8655=CARTESIAN_POINT ( 'NONE',  ( 116.8548138422182063, 38.12265625108393152, -5.444914386472297529 ) ) ;
#8656=CARTESIAN_POINT ( 'NONE',  ( 51.42518405393695957, 32.41757812716787157, 5.622872871577880183 ) ) ;
#8659=CARTESIAN_POINT ( 'NONE',  ( -13.57481594606304753, 34.69960937716787441, -5.622872871577873077 ) ) ;
#8663=CARTESIAN_POINT ( 'NONE',  ( 185.7049497278729575, 39.06523437608392868, 9.295050272127047819 ) ) ;
#8664=CARTESIAN_POINT ( 'NONE',  ( 74.59884440882045453, 38.91640624999999432, 9.598844408820456309 ) ) ;
#8665=CARTESIAN_POINT ( 'NONE',  ( 139.2950502721270425, 36.28710937608393294, -9.295050272127046043 ) ) ;
#8666=CARTESIAN_POINT ( 'NONE',  ( 65.00000000000000000, -7.395377635281828788, -13.57481594606305109 ) ) ;
#8668=CARTESIAN_POINT ( 'NONE',  ( 129.1578924045353460, 53.50112910130382460, 14.99999999999996803 ) ) ;
#8673=CARTESIAN_POINT ( 'NONE',  ( 200.6228728715778686, 33.31054687499999289, 13.57481594606304576 ) ) ;
#8674=EDGE_CURVE ( 'NONE', #18802, #27424, #18193, .T. ) ;
#8676=CARTESIAN_POINT ( 'NONE',  ( 99.99999999999995737, 85.00000000000000000, 4.999999999999990230 ) ) ;
#8677=CARTESIAN_POINT ( 'NONE',  ( 59.55508561352770158, 36.73359375108393010, 13.14518615778179722 ) ) ;
#8682=LINE ( 'NONE', #21946, #3460 ) ;
#8683=CARTESIAN_POINT ( 'NONE',  ( 9.598844408820459861, 36.53515624999999289, 9.598844408820456309 ) ) ;
#8686=CARTESIAN_POINT ( 'NONE',  ( 102.0710678118654329, 83.68750000000001421, -5.000000000000018652 ) ) ;
#8691=CARTESIAN_POINT ( 'NONE',  ( 65.00000000000000000, 33.40976562608393863, -13.14518615778179544 ) ) ;
#8693=CARTESIAN_POINT ( 'NONE',  ( 121.6077847083616206, 54.99999999999998579, -15.00000000000000178 ) ) ;
#8695=ORIENTED_EDGE ( 'NONE', *, *, #23457, .F. ) ;
#8698=CARTESIAN_POINT ( 'NONE',  ( 208.5748159460630120, 38.37070312716786447, -5.622872871577873077 ) ) ;
#8701=CARTESIAN_POINT ( 'NONE',  ( 196.8143553545835402, 51.46618445021835697, 15.00000000000029843 ) ) ;
#8703=CARTESIAN_POINT ( 'NONE',  ( -9.295050272127046043, 37.47773437608393010, -9.295050272127046043 ) ) ;
#8704=CARTESIAN_POINT ( 'NONE',  ( 130.0000000000000000, 35.19570312608392726, 13.14518615778179544 ) ) ;
#8705=CARTESIAN_POINT ( 'NONE',  ( 65.00000000000000000, 34.45156249999999432, -13.57481594606304576 ) ) ;
#8708=CARTESIAN_POINT ( 'NONE',  ( 94.99999999999995737, 84.06250000273119838, -2.071067811865491493 ) ) ;
#8714=CARTESIAN_POINT ( 'NONE',  ( 5.444914386472302859, 37.03125000108393294, 13.14518615778179189 ) ) ;
#8715=CARTESIAN_POINT ( 'NONE',  ( 130.0000000000000000, 50.00000000000000000, 13.57481594606302799 ) ) ;
#8719=CARTESIAN_POINT ( 'NONE',  ( 120.4011555911795455, 37.03125000216787299, -9.598844408820458085 ) ) ;
#8721=ADVANCED_FACE ( 'NONE', ( #11761 ), #26903, .T. ) ;
#8722=CARTESIAN_POINT ( 'NONE',  ( 189.5550856135277229, 38.02343750108394005, -13.14518615778179900 ) ) ;
#8724=CARTESIAN_POINT ( 'NONE',  ( 78.14518615778179367, 36.38632812608393863, -1.609821015232357215E-15 ) ) ;
#8731=CARTESIAN_POINT ( 'NONE',  ( 139.2950502721270425, 39.26367187608393294, 9.295050272127046043 ) ) ;
#8734=CARTESIAN_POINT ( 'NONE',  ( 74.29505027212704249, 39.46210937608393721, 9.295050272127046043 ) ) ;
#8735=LINE ( 'NONE', #15275, #4600 ) ;
#8736=CARTESIAN_POINT ( 'NONE',  ( 185.7049497278729575, 35.29492187608393294, 9.295050272127047819 ) ) ;
#8738=EDGE_LOOP ( 'NONE', ( #25846, #26458, #7064, #17039 ) ) ;
#8745=CARTESIAN_POINT ( 'NONE',  ( 98.15313185440923860, 82.62500000136560629, 4.458734124999987891 ) ) ;
#8746=CARTESIAN_POINT ( 'NONE',  ( 185.7049497278729575, 39.06523437608392868, 9.295050272127047819 ) ) ;
#8748=CARTESIAN_POINT ( 'NONE',  ( 188.8822400544688378, 54.65941425414899157, 14.99999999999995026 ) ) ;
#8749=FACE_OUTER_BOUND ( 'NONE', #18558, .T. ) ;
#8750=CARTESIAN_POINT ( 'NONE',  ( 181.8548138422182205, 40.75195312608393294, 0.000000000000000000 ) ) ;
#8752=VERTEX_POINT ( 'NONE', #27325 ) ;
#8756=CARTESIAN_POINT ( 'NONE',  ( 139.2950502721270425, 35.49335937608393721, 9.295050272127046043 ) ) ;
#8757=CARTESIAN_POINT ( 'NONE',  ( 70.44491438647230552, 33.16171875108393152, -13.14518615778179900 ) ) ;
#8759=CARTESIAN_POINT ( 'NONE',  ( 208.1451861577817795, 38.02343750108395426, -5.444914386472297529 ) ) ;
#8763=CARTESIAN_POINT ( 'NONE',  ( -13.14518615778179189, 31.87187500108393223, 5.444914386472304635 ) ) ;
#8767=CARTESIAN_POINT ( 'NONE',  ( -5.444914386472299306, 35.93984375108392726, 13.14518615778179722 ) ) ;
#8771=CARTESIAN_POINT ( 'NONE',  ( 65.00000000000000000, -7.395377635281828788, 13.57481594606303688 ) ) ;
#8773=ORIENTED_EDGE ( 'NONE', *, *, #4109, .T. ) ;
#8776=CARTESIAN_POINT ( 'NONE',  ( 55.40115559117954547, 38.02343750216788010, 9.598844408820459861 ) ) ;
#8779=DIRECTION ( 'NONE',  ( 0.000000000000000000, 1.000000000000000000, 0.000000000000000000 ) ) ;
#8780=CARTESIAN_POINT ( 'NONE',  ( 99.99999999999995737, 82.43750000136559208, -4.458734125000016313 ) ) ;
#8781=CARTESIAN_POINT ( 'NONE',  ( 55.70494972787295751, 35.89023437608393152, -9.295050272127046043 ) ) ;
#8784=CARTESIAN_POINT ( 'NONE',  ( -9.295050272127046043, 36.48554687608393721, -9.295050272127046043 ) ) ;
#8785=DIRECTION ( 'NONE',  ( 0.000000000000000000, 0.000000000000000000, -1.000000000000000000 ) ) ;
#8786=CARTESIAN_POINT ( 'NONE',  ( 124.3771271284221029, 36.38632812499999858, 13.57481594606300135 ) ) ;
#8788=CARTESIAN_POINT ( 'NONE',  ( 143.5748159460630404, 36.58476562499999574, 5.622872871577869525 ) ) ;
#8792=CARTESIAN_POINT ( 'NONE',  ( 139.2950502721270425, 37.67617187608393436, 9.295050272127046043 ) ) ;
#8793=EDGE_CURVE ( 'NONE', #26308, #19984, #17079, .T. ) ;
#8794=CARTESIAN_POINT ( 'NONE',  ( 65.00000000000000000, 32.96328125216787441, -13.57481594606304576 ) ) ;
#8795=CARTESIAN_POINT ( 'NONE',  ( 102.0710678118654329, 83.68750000000002842, -5.000000000000004441 ) ) ;
#8796=CARTESIAN_POINT ( 'NONE',  ( -5.622872871577873077, 32.51679687716787726, 13.57481594606304753 ) ) ;
#8798=EDGE_CURVE ( 'NONE', #10978, #12157, #369, .T. ) ;
#8801=CARTESIAN_POINT ( 'NONE',  ( 208.1451861577818079, 33.80664062608393294, -1.609821015232357215E-15 ) ) ;
#8804=CARTESIAN_POINT ( 'NONE',  ( 135.4449143864723339, 36.33671875108393579, -13.14518615778179722 ) ) ;
#8807=CARTESIAN_POINT ( 'NONE',  ( 99.99999999999995737, 85.00000000000000000, 4.999999999999990230 ) ) ;
#8810=DIRECTION ( 'NONE',  ( -1.000000000000000000, -1.040834085586055858E-15, 7.228014483236695200E-18 ) ) ;
#8813=CARTESIAN_POINT ( 'NONE',  ( 200.6228728715778686, 34.40195312499999858, -13.57481594606304753 ) ) ;
#8815=CARTESIAN_POINT ( 'NONE',  ( 55.40115559117954547, 40.30546874999999574, 9.598844408820459861 ) ) ;
#8817=CARTESIAN_POINT ( 'NONE',  ( 74.29505027212704249, 34.69960937608393436, -9.295050272127046043 ) ) ;
#8822=CARTESIAN_POINT ( 'NONE',  ( 5.622872871577878406, 37.27929687499999289, 13.57481594606304576 ) ) ;
#8823=CARTESIAN_POINT ( 'NONE',  ( 120.7049497278729575, 37.47773437608393010, -9.295050272127046043 ) ) ;
#8826=CARTESIAN_POINT ( 'NONE',  ( 95.54126587499995082, 80.75000000136560629, 1.846868145590724986 ) ) ;
#8827=CARTESIAN_POINT ( 'NONE',  ( 99.99999999999995737, 82.87500000273119838, -5.000000000000018652 ) ) ;
#8829=CARTESIAN_POINT ( 'NONE',  ( 55.16061839111207377, 36.00000000000002132, -9.004033604613061570 ) ) ;
#8830=ORIENTED_EDGE ( 'NONE', *, *, #12437, .T. ) ;
#8832=CARTESIAN_POINT ( 'NONE',  ( 78.14518615778179367, 33.95546875108393436, 5.444914386472293977 ) ) ;
#8835=ADVANCED_FACE ( 'NONE', ( #20622, #1108 ), #9775, .T. ) ;
#8837=EDGE_LOOP ( 'NONE', ( #10448, #25551, #7286, #8577 ) ) ;
#8840=CARTESIAN_POINT ( 'NONE',  ( 195.0000000000000000, 34.94765625216787441, 13.57481594606304576 ) ) ;
#8845=CARTESIAN_POINT ( 'NONE',  ( 5.444914386472297529, 37.32890625108393579, -13.14518615778179900 ) ) ;
#8846=CARTESIAN_POINT ( 'NONE',  ( 143.1451861577818079, 35.34453125108392868, 5.444914386472293977 ) ) ;
#8847=CARTESIAN_POINT ( 'NONE',  ( 78.57481594606304043, 33.50898437499999716, -5.622872871577873077 ) ) ;
#8848=CARTESIAN_POINT ( 'NONE',  ( 59.37712712842205320, 39.36289062716787157, -13.57481594606297293 ) ) ;
#8850=CARTESIAN_POINT ( 'NONE',  ( 185.8198241863519797, 50.00000000000000000, 9.999999999999952038 ) ) ;
#8857=CARTESIAN_POINT ( 'NONE',  ( -5.444914386472299306, 37.72578125108395142, 13.14518615778179722 ) ) ;
#8861=CARTESIAN_POINT ( 'NONE',  ( 130.0000000000000000, 37.32890625216786873, 13.57481594606304576 ) ) ;
#8862=CARTESIAN_POINT ( 'NONE',  ( 95.27063293749995410, 84.84375000068281736, -1.387778780781445676E-14 ) ) ;
#8863=CARTESIAN_POINT ( 'NONE',  ( 208.1451861577818079, 38.56914062608393579, -1.609821015232357215E-15 ) ) ;
#8865=CARTESIAN_POINT ( 'NONE',  ( 70.44491438647229131, 36.23750000108393721, 13.14518615778179189 ) ) ;
#8867=CARTESIAN_POINT ( 'NONE',  ( 143.5748159460630688, 39.75976562499999289, 5.622872871577868636 ) ) ;
#8872=CARTESIAN_POINT ( 'NONE',  ( 116.4251840539369454, 32.31835937716786589, -5.622872871577873077 ) ) ;
#8873=CARTESIAN_POINT ( 'NONE',  ( 9.295050272127046043, 39.66054687608393436, -9.295050272127046043 ) ) ;
#8875=CARTESIAN_POINT ( 'NONE',  ( 74.29505027212704249, 37.08085937608393579, 9.295050272127046043 ) ) ;
#8876=FACE_OUTER_BOUND ( 'NONE', #9600, .T. ) ;
#8877=CARTESIAN_POINT ( 'NONE',  ( 185.7049497278729575, 34.30273437608393294, -9.295050272127046043 ) ) ;
#8879=EDGE_CURVE ( 'NONE', #19109, #24259, #22902, .T. ) ;
#8880=VERTEX_POINT ( 'NONE', #1244 ) ;
#8881=EDGE_LOOP ( 'NONE', ( #23763, #16304, #23292, #14264, #12803, #2305, #795, #18162, #21533, #16455, #20466, #7903, #2636, #15405, #18987 ) ) ;
#8886=CARTESIAN_POINT ( 'NONE',  ( 55.70494972787295751, 40.45429687608393721, -9.295050272127046043 ) ) ;
#8887=CARTESIAN_POINT ( 'NONE',  ( 98.15313185440923860, 82.25000000136559208, -4.458734125000016313 ) ) ;
#8888=CARTESIAN_POINT ( 'NONE',  ( 200.4449143864723055, 38.42031250108393436, 13.14518615778179189 ) ) ;
#8890=CARTESIAN_POINT ( 'NONE',  ( 186.7314026716027229, 50.00000000054362914, 10.78867689283715414 ) ) ;
#8893=CARTESIAN_POINT ( 'NONE',  ( 74.59884440882045453, 39.90859374999999432, -9.598844408820458085 ) ) ;
#8901=CARTESIAN_POINT ( 'NONE',  ( 116.8548138422182063, 37.62656250108393863, 5.444914386472304635 ) ) ;
#8902=CARTESIAN_POINT ( 'NONE',  ( 70.44491438647230552, 33.65781250108393152, 13.14518615778179189 ) ) ;
#8903=CARTESIAN_POINT ( 'NONE',  ( 195.0000000000000000, 35.79101562608394005, -13.14518615778179544 ) ) ;
#8906=CARTESIAN_POINT ( 'NONE',  ( 128.4945078184423153, 53.60078691996341149, -15.00000000000000000 ) ) ;
#8907=CARTESIAN_POINT ( 'NONE',  ( 70.62287287157796811, 40.75195312499999289, -13.57481594606294095 ) ) ;
#8914=VERTEX_POINT ( 'NONE', #26354 ) ;
#8919=CARTESIAN_POINT ( 'NONE',  ( 125.4284083674797046, 51.44262710532316873, 15.00000000000193978 ) ) ;
#8922=CARTESIAN_POINT ( 'NONE',  ( 98.15313185440925281, 80.50000000136560629, -4.458734125000016313 ) ) ;
#8923=CARTESIAN_POINT ( 'NONE',  ( 78.14518615778179367, 35.64218750108393152, -5.444914386472297529 ) ) ;
#8925=CARTESIAN_POINT ( 'NONE',  ( -5.444914386472299306, 36.73359375108393010, 13.14518615778179722 ) ) ;
#8927=FACE_OUTER_BOUND ( 'NONE', #23393, .T. ) ;
#8928=CARTESIAN_POINT ( 'NONE',  ( 104.9999999999999716, 82.56250000000002842, -2.071067811865491937 ) ) ;
#8929=CARTESIAN_POINT ( 'NONE',  ( 120.4011555911795455, 37.72578124999999005, -9.598844408820458085 ) ) ;
#8935=CARTESIAN_POINT ( 'NONE',  ( 116.8548138422182063, 37.32890625108393579, -5.444914386472297529 ) ) ;
#8936=CARTESIAN_POINT ( 'NONE',  ( 78.57481594606304043, 34.30273437716787299, 5.622872871577869525 ) ) ;
#8938=CARTESIAN_POINT ( 'NONE',  ( 13.57481594606304931, 31.92148437716787512, 5.622872871577869525 ) ) ;
#8939=AXIS2_PLACEMENT_3D ( 'NONE', #23426, #23152, #1493 ) ;
#8943=CARTESIAN_POINT ( 'NONE',  ( 200.4449143864723055, 33.16171875108393152, -13.14518615778179900 ) ) ;
#8946=FACE_OUTER_BOUND ( 'NONE', #10353, .T. ) ;
#8948=CARTESIAN_POINT ( 'NONE',  ( 195.0000000000000000, 36.83281249999999574, -13.57481594606304576 ) ) ;
#8949=CARTESIAN_POINT ( 'NONE',  ( 123.8834397602831672, 54.66944451632671331, 14.99999999999996625 ) ) ;
#8952=AXIS2_PLACEMENT_3D ( 'NONE', #2594, #310, #6989 ) ;
#8955=EDGE_CURVE ( 'NONE', #26695, #17655, #10161, .T. ) ;
#8956=CARTESIAN_POINT ( 'NONE',  ( 181.4251840539369596, 34.69960937499999432, 5.622872871577880183 ) ) ;
#8957=DIRECTION ( 'NONE',  ( 1.000000000000000000, -3.469446951953519526E-16, -2.385244779468110248E-16 ) ) ;
#8959=CARTESIAN_POINT ( 'NONE',  ( 59.55508561352770158, 35.93984375108392726, 13.14518615778179722 ) ) ;
#8960=EDGE_CURVE ( 'NONE', #8135, #9261, #25925, .T. ) ;
#8963=VERTEX_POINT ( 'NONE', #26497 ) ;
#8965=CARTESIAN_POINT ( 'NONE',  ( -5.622872871577873077, 35.59257812499999574, 13.57481594606304753 ) ) ;
#8966=CARTESIAN_POINT ( 'NONE',  ( 139.2950502721270425, 36.28710937608393294, 9.295050272127046043 ) ) ;
#8968=ORIENTED_EDGE ( 'NONE', *, *, #20977, .T. ) ;
#8969=CARTESIAN_POINT ( 'NONE',  ( 99.99999999999995737, 79.93750000136559208, 4.458734124999988779 ) ) ;
#8970=CARTESIAN_POINT ( 'NONE',  ( 97.92893218813451028, 83.31250000273122680, 4.999999999999989342 ) ) ;
#8972=CARTESIAN_POINT ( 'NONE',  ( 64.00443877494754474, 35.99999999999999289, -13.45766439703026407 ) ) ;
#8973=EDGE_CURVE ( 'NONE', #4933, #2793, #9019, .T. ) ;
#8975=CARTESIAN_POINT ( 'NONE',  ( 78.14518615778179367, 33.16171875108393863, 5.444914386472293977 ) ) ;
#8976=ORIENTED_EDGE ( 'NONE', *, *, #22015, .F. ) ;
#8980=CARTESIAN_POINT ( 'NONE',  ( 9.180175813647991845, 55.00000000000000000, -9.999999999999998224 ) ) ;
#8983=CARTESIAN_POINT ( 'NONE',  ( 181.4251840539369596, 33.95546875216787441, 0.000000000000000000 ) ) ;
#8988=CARTESIAN_POINT ( 'NONE',  ( 116.8548138422182205, 36.83281250108393579, 5.444914386472304635 ) ) ;
#8990=CARTESIAN_POINT ( 'NONE',  ( 2.414731522848535132E-15, 34.60039062608393579, 13.14518615778179544 ) ) ;
#8991=CARTESIAN_POINT ( 'NONE',  ( 124.5550856135277087, 35.64218750108392442, -13.14518615778179900 ) ) ;
#8992=CARTESIAN_POINT ( 'NONE',  ( 51.42518405393695957, 34.64999999999999147, 0.000000000000000000 ) ) ;
#9000=CIRCLE ( 'NONE', #2171, 3.000000000000004441 ) ;
#9001=CARTESIAN_POINT ( 'NONE',  ( 102.0710678118654329, 83.43750000273121259, 4.999999999999999112 ) ) ;
#9003=CARTESIAN_POINT ( 'NONE',  ( -13.14518615778179544, 37.57695312608393579, 0.000000000000000000 ) ) ;
#9007=CARTESIAN_POINT ( 'NONE',  ( 195.0000000000000000, 52.00000000000000711, 11.57481594606302266 ) ) ;
#9010=CARTESIAN_POINT ( 'NONE',  ( 189.5550856135277229, 38.81718750108393579, -13.14518615778179900 ) ) ;
#9013=CARTESIAN_POINT ( 'NONE',  ( 9.598844408820459861, 39.80937500216786873, 9.598844408820456309 ) ) ;
#9019=CIRCLE ( 'NONE', #4487, 4.999999999999997335 ) ;
#9020=CARTESIAN_POINT ( 'NONE',  ( 135.6228728715778971, 31.82226562716787654, 13.57481594606304576 ) ) ;
#9024=CARTESIAN_POINT ( 'NONE',  ( 70.44491438647230552, 38.91640625108393436, -13.14518615778179900 ) ) ;
#9025=CARTESIAN_POINT ( 'NONE',  ( 62.72385315545274409, 51.46995505939283078, -14.99999999999999822 ) ) ;
#9026=CARTESIAN_POINT ( 'NONE',  ( 189.5550856135277229, 32.66562500108393863, -13.14518615778179900 ) ) ;
#9029=ORIENTED_EDGE ( 'NONE', *, *, #22243, .T. ) ;
#9030=EDGE_LOOP ( 'NONE', ( #11869, #22814, #11579, #9289 ) ) ;
#9033=CARTESIAN_POINT ( 'NONE',  ( 78.14518615778180788, 39.41250000108393436, -5.444914386472297529 ) ) ;
#9034=CARTESIAN_POINT ( 'NONE',  ( 59.37712712842218821, 36.48554687716787726, 13.57481594606311504 ) ) ;
#9035=CARTESIAN_POINT ( 'NONE',  ( 195.0000000000000000, 38.37070312608393152, 13.14518615778179544 ) ) ;
#9037=CARTESIAN_POINT ( 'NONE',  ( 195.0000000000000000, 38.51953125216787299, -13.57481594606304576 ) ) ;
#9040=CIRCLE ( 'NONE', #15809, 3.000000000000004441 ) ;
#9045=VERTEX_POINT ( 'NONE', #5259 ) ;
#9047=CARTESIAN_POINT ( 'NONE',  ( 59.55508561352770158, 34.05468750108393294, -13.14518615778179900 ) ) ;
#9048=CARTESIAN_POINT ( 'NONE',  ( 189.5550856135277229, 38.51953125108393294, 13.14518615778179722 ) ) ;
#9050=LINE ( 'NONE', #13295, #5700 ) ;
#9051=CARTESIAN_POINT ( 'NONE',  ( -13.14518615778179900, 31.77265625108393365, -5.444914386472297529 ) ) ;
#9054=CARTESIAN_POINT ( 'NONE',  ( 74.59884440882045453, 40.70234374999999716, -9.598844408820458085 ) ) ;
#9055=CARTESIAN_POINT ( 'NONE',  ( 0.000000000000000000, -7.395377635281828788, 11.57481594606304398 ) ) ;
#9057=CARTESIAN_POINT ( 'NONE',  ( 60.07497321633574217, 49.99999999893042713, 12.67776588291749462 ) ) ;
#9058=EDGE_LOOP ( 'NONE', ( #5031, #14291, #5282, #20124 ) ) ;
#9066=CARTESIAN_POINT ( 'NONE',  ( 103.1528011352953342, 81.31250000136559208, -3.152801135295383084 ) ) ;
#9067=CARTESIAN_POINT ( 'NONE',  ( 74.29505027212704249, 35.69179687608394147, -9.295050272127046043 ) ) ;
#9069=CARTESIAN_POINT ( 'NONE',  ( 9.295050272127046043, 36.28710937608393294, -9.295050272127046043 ) ) ;
#9072=CARTESIAN_POINT ( 'NONE',  ( 124.3771271284221314, 37.67617187499999432, -13.57481594606304753 ) ) ;
#9073=EDGE_LOOP ( 'NONE', ( #19668, #18083, #16582, #24136 ) ) ;
#9074=VERTEX_POINT ( 'NONE', #11929 ) ;
#9079=CARTESIAN_POINT ( 'NONE',  ( 116.8548138422182063, 36.53515625108392584, -5.444914386472297529 ) ) ;
#9080=CARTESIAN_POINT ( 'NONE',  ( 51.42518405393695957, 34.79882812716787299, 5.622872871577880183 ) ) ;
#9081=EDGE_CURVE ( 'NONE', #20134, #152, #15843, .T. ) ;
#9082=CARTESIAN_POINT ( 'NONE',  ( 99.99999999999995737, 83.75000000000000000, -5.000000000000018652 ) ) ;
#9083=CARTESIAN_POINT ( 'NONE',  ( -5.622872871577873077, 33.31054687716787299, 13.57481594606304753 ) ) ;
#9087=CARTESIAN_POINT ( 'NONE',  ( 204.2950502721270425, 34.50117187608393010, 9.295050272127046043 ) ) ;
#9088=CYLINDRICAL_SURFACE ( 'NONE', #21107, 13.57481594606304398 ) ;
#9089=AXIS2_PLACEMENT_3D ( 'NONE', #3758, #7883, #5759 ) ;
#9090=CARTESIAN_POINT ( 'NONE',  ( 103.5355339059327093, 81.62500000000000000, -3.535533905932755072 ) ) ;
#9094=CARTESIAN_POINT ( 'NONE',  ( 130.7197605961091824, 53.51499872091923038, 14.99999999999996447 ) ) ;
#9099=CARTESIAN_POINT ( 'NONE',  ( 200.6228728715778686, 35.98945312499999716, -13.57481594606304753 ) ) ;
#9102=CARTESIAN_POINT ( 'NONE',  ( 51.85481384221820633, 35.79101562608393294, 0.000000000000000000 ) ) ;
#9107=CARTESIAN_POINT ( 'NONE',  ( -13.57481594606304753, 37.77539062499999289, -5.622872871577873077 ) ) ;
#9108=CARTESIAN_POINT ( 'NONE',  ( 139.2950502721270425, 38.66835937608393436, 9.295050272127046043 ) ) ;
#9110=CARTESIAN_POINT ( 'NONE',  ( 96.84719886470459471, 80.56250000136559208, -3.152801135295383084 ) ) ;
#9111=FACE_OUTER_BOUND ( 'NONE', #20130, .T. ) ;
#9112=CARTESIAN_POINT ( 'NONE',  ( 99.99999999999995737, 81.37500000273119838, 4.999999999999990230 ) ) ;
#9116=CARTESIAN_POINT ( 'NONE',  ( 51.42518405393695957, 39.46210937499999005, 5.622872871577880183 ) ) ;
#9118=EDGE_CURVE ( 'NONE', #27809, #1909, #12001, .T. ) ;
#9119=CARTESIAN_POINT ( 'NONE',  ( 214.9999999999999716, 75.00000000000000000, 0.000000000000000000 ) ) ;
#9121=EDGE_CURVE ( 'NONE', #25739, #18276, #20425, .T. ) ;
#9124=CARTESIAN_POINT ( 'NONE',  ( 200.6228728715778686, 35.79101562716787299, 13.57481594606304576 ) ) ;
#9127=CARTESIAN_POINT ( 'NONE',  ( 130.0000000000000000, 36.98164062608393721, 13.14518615778179544 ) ) ;
#9128=ORIENTED_EDGE ( 'NONE', *, *, #5622, .F. ) ;
#9129=CARTESIAN_POINT ( 'NONE',  ( 9.295050272127046043, 36.48554687608393721, -9.295050272127046043 ) ) ;
#9131=CARTESIAN_POINT ( 'NONE',  ( 55.40115559117954547, 35.34453124999998863, -9.598844408820458085 ) ) ;
#9134=CARTESIAN_POINT ( 'NONE',  ( 99.99999999999995737, 85.00000000000000000, -1.387778780781445676E-14 ) ) ;
#9135=AXIS2_PLACEMENT_3D ( 'NONE', #9404, #26672, #20395 ) ;
#9139=DIRECTION ( 'NONE',  ( -0.000000000000000000, 1.000000000000000000, -0.000000000000000000 ) ) ;
#9141=CARTESIAN_POINT ( 'NONE',  ( -13.14518615778179189, 35.24531250108393721, 5.444914386472304635 ) ) ;
#9149=CARTESIAN_POINT ( 'NONE',  ( 208.1451861577818079, 36.18789062608393436, -1.609821015232357215E-15 ) ) ;
#9156=CIRCLE ( 'NONE', #7059, 5.000000000000004441 ) ;
#9159=EDGE_CURVE ( 'NONE', #10007, #26290, #14073, .T. ) ;
#9160=CARTESIAN_POINT ( 'NONE',  ( 139.5988444088204687, 31.87187500216787228, 9.598844408820456309 ) ) ;
#9161=CARTESIAN_POINT ( 'NONE',  ( -9.295050272127046043, 40.65273437608393436, -9.295050272127046043 ) ) ;
#9163=CARTESIAN_POINT ( 'NONE',  ( 78.14518615778179367, 37.22968750108393721, -5.444914386472297529 ) ) ;
#9164=CARTESIAN_POINT ( 'NONE',  ( 61.02018555418613488, 50.00000000123296218, -13.01613927312751429 ) ) ;
#9166=CARTESIAN_POINT ( 'NONE',  ( 204.2950502721270425, 33.11210937608393579, 9.295050272127046043 ) ) ;
#9172=CARTESIAN_POINT ( 'NONE',  ( 51.85481384221820633, 38.17226562608393436, 0.000000000000000000 ) ) ;
#9175=ORIENTED_EDGE ( 'NONE', *, *, #28145, .T. ) ;
#9178=CARTESIAN_POINT ( 'NONE',  ( 181.8548138422182205, 38.42031250108393436, 5.444914386472304635 ) ) ;
#9180=ORIENTED_EDGE ( 'NONE', *, *, #16115, .T. ) ;
#9183=ORIENTED_EDGE ( 'NONE', *, *, #608, .T. ) ;
#9184=CARTESIAN_POINT ( 'NONE',  ( 124.5550856135277087, 33.75703125108393721, 13.14518615778179722 ) ) ;
#9185=CARTESIAN_POINT ( 'NONE',  ( 65.00000000000000000, 35.19570312608392726, 13.14518615778179544 ) ) ;
#9186=CARTESIAN_POINT ( 'NONE',  ( 204.2950502721270425, 36.28710937608393294, 9.295050272127046043 ) ) ;
#9189=CARTESIAN_POINT ( 'NONE',  ( -13.14518615778179900, 33.36015625108393579, -5.444914386472297529 ) ) ;
#9192=CARTESIAN_POINT ( 'NONE',  ( 120.4011555911795455, 40.20625000216787726, -9.598844408820458085 ) ) ;
#9194=DIRECTION ( 'NONE',  ( -0.000000000000000000, 1.000000000000000000, -0.000000000000000000 ) ) ;
#9196=CARTESIAN_POINT ( 'NONE',  ( 67.52958399517125088, 49.99999999938368944, 13.34625891065909897 ) ) ;
#9206=CARTESIAN_POINT ( 'NONE',  ( 55.70494972787295751, 35.29492187608393294, 9.295050272127047819 ) ) ;
#9207=CARTESIAN_POINT ( 'NONE',  ( 189.3771271284220745, 37.67617187499999432, -13.57481594606304753 ) ) ;
#9208=CARTESIAN_POINT ( 'NONE',  ( -13.14518615778179722, 37.32890625108393579, -5.444914386472297529 ) ) ;
#9210=CARTESIAN_POINT ( 'NONE',  ( 8.259611528887869980, 50.00000000056319038, 10.79618466885915851 ) ) ;
#9212=CARTESIAN_POINT ( 'NONE',  ( 130.0000000000000000, 36.83281249999999574, -13.57481594606304576 ) ) ;
#9213=ORIENTED_EDGE ( 'NONE', *, *, #3429, .T. ) ;
#9214=VECTOR ( 'NONE', #1366, 1000.000000000000000 ) ;
#9215=ORIENTED_EDGE ( 'NONE', *, *, #5672, .F. ) ;
#9219=( BOUNDED_CURVE ( )  B_SPLINE_CURVE ( 2, ( #20478, #1100, #4801, #2801, #13460, #20047, #24459, #9207, #17901 ),
 .UNSPECIFIED., .F., .F. ) 
 B_SPLINE_CURVE_WITH_KNOTS ( ( 3, 2, 2, 2, 3 ),
 ( 0.3125000000000002220, 0.3229166666666668517, 0.3333333333333334259, 0.3437500000000000555, 0.3541666666666666852 ),
 .UNSPECIFIED. ) 
 CURVE ( )  GEOMETRIC_REPRESENTATION_ITEM ( )  RATIONAL_B_SPLINE_CURVE ( ( 0.9999999999999983347, 0.9238795325112884038, 1.000000000000000000, 0.9238795325112867385, 1.000000000000000000, 0.9238795325112867385, 1.000000000000000000, 0.9238795325112867385, 1.000000000000000000 ) ) 
 REPRESENTATION_ITEM ( '' )  );
#9221=CARTESIAN_POINT ( 'NONE',  ( 120.7049497278729575, 33.50898437608393010, 9.295050272127047819 ) ) ;
#9222=CARTESIAN_POINT ( 'NONE',  ( 59.37712712842213136, 34.60039062716786873, -13.57481594606304753 ) ) ;
#9223=DIRECTION ( 'NONE',  ( 1.000000000000000000, 0.000000000000000000, -2.385244779468110248E-16 ) ) ;
#9224=CARTESIAN_POINT ( 'NONE',  ( 13.57481594606304931, 33.50898437716787015, 5.622872871577869525 ) ) ;
#9228=CARTESIAN_POINT ( 'NONE',  ( 185.7049497278729575, 35.89023437608393152, 9.295050272127047819 ) ) ;
#9237=CARTESIAN_POINT ( 'NONE',  ( -9.180175813648000727, 55.00000000000014211, -9.999999999999998224 ) ) ;
#9240=CARTESIAN_POINT ( 'NONE',  ( 195.0000000000000000, 33.65781249999999147, -13.57481594606304576 ) ) ;
#9243=CARTESIAN_POINT ( 'NONE',  ( 55.70494972787295751, 35.09648437608392868, 9.295050272127047819 ) ) ;
#9245=CARTESIAN_POINT ( 'NONE',  ( 195.0000000000000000, -7.395377635281828788, 13.57481594606302266 ) ) ;
#9249=CARTESIAN_POINT ( 'NONE',  ( -5.622872871577873077, 37.67617187499999432, -13.57481594606304753 ) ) ;
#9250=CARTESIAN_POINT ( 'NONE',  ( 116.8548138422182063, 37.62656250108393863, 5.444914386472304635 ) ) ;
#9252=CARTESIAN_POINT ( 'NONE',  ( 94.99999999999995737, 80.00000000000000000, -1.387778780781445676E-14 ) ) ;
#9254=CARTESIAN_POINT ( 'NONE',  ( 104.9999999999999574, 82.56250000273119838, 2.071067811865462627 ) ) ;
#9258=CARTESIAN_POINT ( 'NONE',  ( 78.57481594606304043, 40.55351562499998863, 5.622872871577869525 ) ) ;
#9259=VERTEX_POINT ( 'NONE', #1822 ) ;
#9261=VERTEX_POINT ( 'NONE', #12064 ) ;
#9263=CARTESIAN_POINT ( 'NONE',  ( 195.0000000000000000, 34.15390625216787157, 13.57481594606304576 ) ) ;
#9265=DIRECTION ( 'NONE',  ( 0.000000000000000000, 0.000000000000000000, 1.000000000000000000 ) ) ;
#9266=CARTESIAN_POINT ( 'NONE',  ( 116.8548138422182205, 37.57695312608393579, 0.000000000000000000 ) ) ;
#9267=CARTESIAN_POINT ( 'NONE',  ( 9.295050272127047819, 33.90585937608393863, 9.295050272127046043 ) ) ;
#9270=CARTESIAN_POINT ( 'NONE',  ( 70.62287287157786864, 33.60820312499998863, -13.57481594606304753 ) ) ;
#9274=AXIS2_PLACEMENT_3D ( 'NONE', #19218, #6250, #23501 ) ;
#9280=CARTESIAN_POINT ( 'NONE',  ( 2.414731522848535132E-15, 36.98164062608393721, 13.14518615778179544 ) ) ;
#9282=CYLINDRICAL_SURFACE ( 'NONE', #23658, 13.57481594606304398 ) ;
#9285=CARTESIAN_POINT ( 'NONE',  ( 181.8548138422181921, 35.04687500108393294, 5.444914386472304635 ) ) ;
#9286=EDGE_LOOP ( 'NONE', ( #27974, #19573, #20621, #27720 ) ) ;
#9287=CARTESIAN_POINT ( 'NONE',  ( 203.2685973283972771, 50.00000000054347993, -10.78867689283658216 ) ) ;
#9289=ORIENTED_EDGE ( 'NONE', *, *, #17160, .T. ) ;
#9293=CARTESIAN_POINT ( 'NONE',  ( 124.5550856135277087, 37.22968750108393721, -13.14518615778179900 ) ) ;
#9294=CARTESIAN_POINT ( 'NONE',  ( 99.99999999999995737, 82.87500000273119838, -5.000000000000018652 ) ) ;
#9295=CARTESIAN_POINT ( 'NONE',  ( -13.14518615778179544, 34.99726562608393721, 0.000000000000000000 ) ) ;
#9298=( BOUNDED_SURFACE ( )  B_SPLINE_SURFACE ( 1, 2, ( 
 ( #25211, #5699, #14366, #11945, #3557, #24791, #15940, #20943, #5419, #12214, #9392, #7390, #14089, #27085, #16376, #16083, #26800, #7250, #5564, #24656, #14227, #13939, #3409, #5129, #13796, #22519, #20381, #866, #9539, #22665, #3135, #11805, #20528, #25624, #8518, #3973, #12360, #8233, #14913, #23221, #19067, #21217, #21492, #23633, #10219, #27912, #25353, #1840, #12905, #18930, #1973, #5969, #19348, #10641, #5836, #12490, #4245, #1425, #6106, #18796, #6244, #10084, #14638, #3697, #4110, #23356, #1701, #17058, #8098, #27503, #3829, #14504, #16924, #25762, #27775, #16792, #7958, #10359, #14773, #25491, #28051, #17203, #25908, #6378, #23493, #12776, #12633, #16658, #21078, #21360, #15052, #23769, #27638, #10503, #19210, #8374, #1567, #24475, #2111, #19767, #11339, #4672, #10920, #22060, #24330, #2400, #13334, #6935, #15478, #11057, #22199, #9080, #6649, #539, #17626, #9222, #24193, #4387, #250, #15629, #15190, #8936, #26332, #15335, #23907, #6514, #20060, #13045, #2535, #15767, #21779, #10778, #6793, #17914, #11198, #26625, #17484, #2678, #7072, #13186, #2258, #19630, #13475, #19915, #111, #398, #17775, #21924, #8794, #26479, #4814, #4959, #26183, #21635, #24051, #17347, #4526, #19490, #28188, #8656, #26044, #7355, #25040, #18346, #11905, #14189, #972, #18488, #27197, #16048, #13621, #9780, #3100, #22908, #26765, #16340, #5097, #24619, #5381, #11766, #5238, #9498, #2949 ),
 ( #16194, #3370, #12041, #11620, #24756, #7209, #20765, #13760, #5522, #20490, #9641, #7648, #14050, #1250, #2813, #22343, #9912, #18627, #13903, #7499, #27330, #22630, #7789, #27050, #16476, #25171, #11482, #20199, #24901, #20345, #18199, #22771, #3237, #20629, #22484, #684, #1113, #15902, #9359, #18052, #832, #26909, #19026, #21178, #6070, #27738, #12452, #21318, #8479, #12593, #3660, #17169, #25587, #5661, #10465, #14877, #14324, #12177, #18888, #8198, #10319, #21460, #23184, #8337, #27875, #10179, #25454, #23045, #3793, #16888, #18761, #6207, #23456, #20907, #1659, #1800, #17021, #12736, #25724, #14736, #1938, #1389, #3934, #19173, #23592, #23320, #4074, #10607, #19314, #28015, #3518, #10050, #27465, #7922, #16753, #16619, #25311, #5800, #14466, #5934, #12321, #27598, #8059, #21042, #1527, #14602, #4633, #24015, #9185, #2497, #6899, #504, #4209, #10884, #11017, #2362, #13436, #15153, #360, #19874, #2220, #17449, #25871, #4493, #19730, #10743, #26440, #15441, #12868, #13150, #13291, #9047, #4775, #17738, #21888, #22163, #21598, #215, #11159, #8902, #15299, #15586, #17590, #26297, #24294, #6758, #2075, #24156, #6340, #8757, #15014, #2641, #11303, #22020, #26148, #20024, #19593, #76, #4351, #23736, #19454, #28152, #8619, #6615, #17307, #26007, #6478, #23872, #13005, #21745, #9320, #647, #9606, #7321, #9461, #13726, #7173, #22874, #18308, #20165, #3339, #25004, #5062 ) ),
 .UNSPECIFIED., .F., .F., .F. ) 
 B_SPLINE_SURFACE_WITH_KNOTS ( ( 2, 2 ),
 ( 3, 2, 2, 2, 2, 2, 2, 2, 2, 2, 2, 2, 2, 2, 2, 2, 2, 2, 2, 2, 2, 2, 2, 2, 2, 2, 2, 2, 2, 2, 2, 2, 2, 2, 2, 2, 2, 2, 2, 2, 2, 2, 2, 2, 2, 2, 2, 2, 2, 2, 2, 2, 2, 2, 2, 2, 2, 2, 2, 2, 2, 2, 2, 2, 2, 2, 2, 2, 2, 2, 2, 2, 2, 2, 2, 2, 2, 2, 2, 2, 2, 2, 2, 2, 2, 2, 2, 2, 2, 2, 2, 3 ),
 ( 0.000000000000000000, 1.000000000000000000 ),
 ( 0.000000000000000000, 0.01041666666666666609, 0.02083333333333333218, 0.03125000000000000000, 0.04166666666666666435, 0.05208333333333333565, 0.06250000000000000000, 0.07291666666666667129, 0.08333333333333332871, 0.09375000000000000000, 0.1041666666666666713, 0.1145833333333333287, 0.1250000000000000000, 0.1354166666666666574, 0.1458333333333333426, 0.1562500000000000000, 0.1666666666666666574, 0.1770833333333333426, 0.1875000000000000000, 0.1979166666666666574, 0.2083333333333333426, 0.2187500000000000000, 0.2291666666666666574, 0.2395833333333333426, 0.2500000000000000000, 0.2604166666666666852, 0.2708333333333333148, 0.2812500000000000000, 0.2916666666666666852, 0.3020833333333333148, 0.3125000000000000000, 0.3229166666666666852, 0.3333333333333333148, 0.3437500000000000000, 0.3541666666666666852, 0.3645833333333333148, 0.3750000000000000000, 0.3854166666666666852, 0.3958333333333333148, 0.4062500000000000000, 0.4166666666666666852, 0.4270833333333333148, 0.4375000000000000000, 0.4479166666666666852, 0.4583333333333333148, 0.4687500000000000000, 0.4791666666666666852, 0.4895833333333333148, 0.5000000000000000000, 0.5104166666666666297, 0.5208333333333333703, 0.5312500000000000000, 0.5416666666666666297, 0.5520833333333333703, 0.5625000000000000000, 0.5729166666666666297, 0.5833333333333333703, 0.5937500000000000000, 0.6041666666666666297, 0.6145833333333333703, 0.6250000000000000000, 0.6354166666666666297, 0.6458333333333333703, 0.6562500000000000000, 0.6666666666666666297, 0.6770833333333333703, 0.6875000000000000000, 0.6979166666666666297, 0.7083333333333333703, 0.7187500000000000000, 0.7291666666666666297, 0.7395833333333333703, 0.7500000000000000000, 0.7604166666666666297, 0.7708333333333333703, 0.7812500000000000000, 0.7916666666666666297, 0.8020833333333333703, 0.8125000000000000000, 0.8229166666666666297, 0.8333333333333333703, 0.8437500000000000000, 0.8541666666666666297, 0.8645833333333333703, 0.8750000000000000000, 0.8854166666666666297, 0.8958333333333333703, 0.9062500000000000000, 0.9166666666666666297, 0.9270833333333333703, 0.9375000000000000000, 0.9448586970929392370 ),
 .UNSPECIFIED. ) 
 GEOMETRIC_REPRESENTATION_ITEM ( )  RATIONAL_B_SPLINE_SURFACE ( (
 ( 1.000000000000000000, 0.9238795325112867385, 1.000000000000000000, 0.9238795325112867385, 1.000000000000000000, 0.9238795325112867385, 1.000000000000000000, 0.9238795325112867385, 1.000000000000000000, 0.9238795325112867385, 1.000000000000000000, 0.9238795325112867385, 1.000000000000000000, 0.9238795325112867385, 1.000000000000000000, 0.9238795325112867385, 1.000000000000000000, 0.9238795325112867385, 1.000000000000000000, 0.9238795325112867385, 1.000000000000000000, 0.9238795325112867385, 1.000000000000000000, 0.9238795325112867385, 1.000000000000000000, 0.9238795325112867385, 1.000000000000000000, 0.9238795325112867385, 1.000000000000000000, 0.9238795325112867385, 1.000000000000000000, 0.9238795325112867385, 1.000000000000000000, 0.9238795325112867385, 1.000000000000000000, 0.9238795325112867385, 1.000000000000000000, 0.9238795325112867385, 1.000000000000000000, 0.9238795325112867385, 1.000000000000000000, 0.9238795325112867385, 1.000000000000000000, 0.9238795325112867385, 1.000000000000000000, 0.9238795325112867385, 1.000000000000000000, 0.9238795325112867385, 1.000000000000000000, 0.9238795325112867385, 1.000000000000000000, 0.9238795325112867385, 1.000000000000000000, 0.9238795325112867385, 1.000000000000000000, 0.9238795325112867385, 1.000000000000000000, 0.9238795325112867385, 1.000000000000000000, 0.9238795325112867385, 1.000000000000000000, 0.9238795325112867385, 1.000000000000000000, 0.9238795325112867385, 1.000000000000000000, 0.9238795325112867385, 1.000000000000000000, 0.9238795325112867385, 1.000000000000000000, 0.9238795325112867385, 1.000000000000000000, 0.9238795325112867385, 1.000000000000000000, 0.9238795325112867385, 1.000000000000000000, 0.9238795325112867385, 1.000000000000000000, 0.9238795325112867385, 1.000000000000000000, 0.9238795325112867385, 1.000000000000000000, 0.9238795325112867385, 1.000000000000000000, 0.9238795325112867385, 1.000000000000000000, 0.9238795325112867385, 1.000000000000000000, 0.9238795325112867385, 1.000000000000000000, 0.9238795325112867385, 1.000000000000000000, 0.9238795325112867385, 1.000000000000000000, 0.9238795325112867385, 1.000000000000000000, 0.9238795325112867385, 1.000000000000000000, 0.9238795325112867385, 1.000000000000000000, 0.9238795325112867385, 1.000000000000000000, 0.9238795325112867385, 1.000000000000000000, 0.9238795325112867385, 1.000000000000000000, 0.9238795325112867385, 1.000000000000000000, 0.9238795325112867385, 1.000000000000000000, 0.9238795325112867385, 1.000000000000000000, 0.9238795325112867385, 1.000000000000000000, 0.9238795325112867385, 1.000000000000000000, 0.9238795325112867385, 1.000000000000000000, 0.9238795325112867385, 1.000000000000000000, 0.9238795325112867385, 1.000000000000000000, 0.9238795325112867385, 1.000000000000000000, 0.9238795325112867385, 1.000000000000000000, 0.9238795325112867385, 1.000000000000000000, 0.9238795325112867385, 1.000000000000000000, 0.9238795325112867385, 1.000000000000000000, 0.9238795325112867385, 1.000000000000000000, 0.9238795325112867385, 1.000000000000000000, 0.9238795325112867385, 1.000000000000000000, 0.9238795325112867385, 1.000000000000000000, 0.9238795325112867385, 1.000000000000000000, 0.9238795325112867385, 1.000000000000000000, 0.9238795325112867385, 1.000000000000000000, 0.9238795325112867385, 1.000000000000000000, 0.9238795325112867385, 1.000000000000000000, 0.9238795325112867385, 1.000000000000000000, 0.9238795325112867385, 1.000000000000000000, 0.9238795325112867385, 1.000000000000000000, 0.9238795325112867385, 1.000000000000000000, 0.9238795325112867385, 1.000000000000000000, 0.9238795325112867385, 1.000000000000000000, 0.9238795325112867385, 1.000000000000000000, 0.9238795325112867385, 1.000000000000000000, 0.9238795325112867385, 1.000000000000000000, 0.9238795325112867385, 1.000000000000000000, 0.9238795325112867385, 1.000000000000000000, 0.9238795325112867385, 1.000000000000000000, 0.9238795325112867385, 1.000000000000000000, 0.9238795325112867385, 1.000000000000000000, 0.9238795325112867385, 1.000000000000000000, 0.9238795325112867385, 1.000000000000000000, 0.9462258435690522607, 0.9684275710300105366),
 ( 1.000000000000000000, 0.9238795325112867385, 1.000000000000000000, 0.9238795325112867385, 1.000000000000000000, 0.9238795325112867385, 1.000000000000000000, 0.9238795325112867385, 1.000000000000000000, 0.9238795325112867385, 1.000000000000000000, 0.9238795325112867385, 1.000000000000000000, 0.9238795325112867385, 1.000000000000000000, 0.9238795325112867385, 1.000000000000000000, 0.9238795325112867385, 1.000000000000000000, 0.9238795325112867385, 1.000000000000000000, 0.9238795325112867385, 1.000000000000000000, 0.9238795325112867385, 1.000000000000000000, 0.9238795325112867385, 1.000000000000000000, 0.9238795325112867385, 1.000000000000000000, 0.9238795325112867385, 1.000000000000000000, 0.9238795325112867385, 1.000000000000000000, 0.9238795325112867385, 1.000000000000000000, 0.9238795325112867385, 1.000000000000000000, 0.9238795325112867385, 1.000000000000000000, 0.9238795325112867385, 1.000000000000000000, 0.9238795325112867385, 1.000000000000000000, 0.9238795325112867385, 1.000000000000000000, 0.9238795325112867385, 1.000000000000000000, 0.9238795325112867385, 1.000000000000000000, 0.9238795325112867385, 1.000000000000000000, 0.9238795325112867385, 1.000000000000000000, 0.9238795325112867385, 1.000000000000000000, 0.9238795325112867385, 1.000000000000000000, 0.9238795325112867385, 1.000000000000000000, 0.9238795325112867385, 1.000000000000000000, 0.9238795325112867385, 1.000000000000000000, 0.9238795325112867385, 1.000000000000000000, 0.9238795325112867385, 1.000000000000000000, 0.9238795325112867385, 1.000000000000000000, 0.9238795325112867385, 1.000000000000000000, 0.9238795325112867385, 1.000000000000000000, 0.9238795325112867385, 1.000000000000000000, 0.9238795325112867385, 1.000000000000000000, 0.9238795325112867385, 1.000000000000000000, 0.9238795325112867385, 1.000000000000000000, 0.9238795325112867385, 1.000000000000000000, 0.9238795325112867385, 1.000000000000000000, 0.9238795325112867385, 1.000000000000000000, 0.9238795325112867385, 1.000000000000000000, 0.9238795325112867385, 1.000000000000000000, 0.9238795325112867385, 1.000000000000000000, 0.9238795325112867385, 1.000000000000000000, 0.9238795325112867385, 1.000000000000000000, 0.9238795325112867385, 1.000000000000000000, 0.9238795325112867385, 1.000000000000000000, 0.9238795325112867385, 1.000000000000000000, 0.9238795325112867385, 1.000000000000000000, 0.9238795325112867385, 1.000000000000000000, 0.9238795325112867385, 1.000000000000000000, 0.9238795325112867385, 1.000000000000000000, 0.9238795325112867385, 1.000000000000000000, 0.9238795325112867385, 1.000000000000000000, 0.9238795325112867385, 1.000000000000000000, 0.9238795325112867385, 1.000000000000000000, 0.9238795325112867385, 1.000000000000000000, 0.9238795325112867385, 1.000000000000000000, 0.9238795325112867385, 1.000000000000000000, 0.9238795325112867385, 1.000000000000000000, 0.9238795325112867385, 1.000000000000000000, 0.9238795325112867385, 1.000000000000000000, 0.9238795325112867385, 1.000000000000000000, 0.9238795325112867385, 1.000000000000000000, 0.9238795325112867385, 1.000000000000000000, 0.9238795325112867385, 1.000000000000000000, 0.9238795325112867385, 1.000000000000000000, 0.9238795325112867385, 1.000000000000000000, 0.9238795325112867385, 1.000000000000000000, 0.9238795325112867385, 1.000000000000000000, 0.9238795325112867385, 1.000000000000000000, 0.9238795325112867385, 1.000000000000000000, 0.9238795325112867385, 1.000000000000000000, 0.9238795325112867385, 1.000000000000000000, 0.9238795325112867385, 1.000000000000000000, 0.9238795325112867385, 1.000000000000000000, 0.9238795325112867385, 1.000000000000000000, 0.9238795325112867385, 1.000000000000000000, 0.9238795325112867385, 1.000000000000000000, 0.9238795325112867385, 1.000000000000000000, 0.9238795325112867385, 1.000000000000000000, 0.9238795325112867385, 1.000000000000000000, 0.9238795325112867385, 1.000000000000000000, 0.9238795325112867385, 1.000000000000000000, 0.9238795325112867385, 1.000000000000000000, 0.9238795325112867385, 1.000000000000000000, 0.9238795325112867385, 1.000000000000000000, 0.9462258435690522607, 0.9684275710300105366) ) ) 
 REPRESENTATION_ITEM ( '' )  SURFACE ( )  );
#9299=CARTESIAN_POINT ( 'NONE',  ( 78.14518615778179367, 37.97382812608393721, -1.609821015232357215E-15 ) ) ;
#9300=CARTESIAN_POINT ( 'NONE',  ( 64.60300058535341350, 51.45716825712325715, -15.00000000000000178 ) ) ;
#9302=CARTESIAN_POINT ( 'NONE',  ( 198.7556381558599696, 31.78804748261757140, -13.14518615778179367 ) ) ;
#9303=FACE_OUTER_BOUND ( 'NONE', #27849, .T. ) ;
#9307=CARTESIAN_POINT ( 'NONE',  ( 74.29505027212704249, 37.67617187608393436, 9.295050272127046043 ) ) ;
#9309=EDGE_CURVE ( 'NONE', #4613, #18339, #541, .T. ) ;
#9312=CARTESIAN_POINT ( 'NONE',  ( 181.8548138422182205, 39.16445312608393436, 0.000000000000000000 ) ) ;
#9315=CIRCLE ( 'NONE', #18878, 5.000000000000004441 ) ;
#9318=ORIENTED_EDGE ( 'NONE', *, *, #6735, .T. ) ;
#9319=CARTESIAN_POINT ( 'NONE',  ( 116.8548138422182063, 33.55859375108393294, -5.444914386472297529 ) ) ;
#9320=CARTESIAN_POINT ( 'NONE',  ( 74.29505027212704249, 32.11992187608393579, 9.295050272127046043 ) ) ;
#9322=CARTESIAN_POINT ( 'NONE',  ( 204.2950502721270425, 33.31054687608394005, -9.295050272127046043 ) ) ;
#9325=CARTESIAN_POINT ( 'NONE',  ( -0.3286002765684034599, 53.49358765998907472, -14.99999999999999822 ) ) ;
#9326=CARTESIAN_POINT ( 'NONE',  ( 130.0000000000000000, -7.395377635281828788, -13.57481594606305997 ) ) ;
#9327=DIRECTION ( 'NONE',  ( 0.000000000000000000, 1.000000000000000000, 0.000000000000000000 ) ) ;
#9329=CARTESIAN_POINT ( 'NONE',  ( 65.00000000000000000, -7.395377635281828788, -7.517135062566165128E-15 ) ) ;
#9331=CARTESIAN_POINT ( 'NONE',  ( 181.8548138422182205, 40.75195312608393294, 0.000000000000000000 ) ) ;
#9333=AXIS2_PLACEMENT_3D ( 'NONE', #24635, #11783, #27485 ) ;
#9336=ORIENTED_EDGE ( 'NONE', *, *, #25348, .F. ) ;
#9337=CARTESIAN_POINT ( 'NONE',  ( -12.85950995607747949, 36.00000000000000711, -3.245221471867173246 ) ) ;
#9341=CARTESIAN_POINT ( 'NONE',  ( -10.78684676818434518, 35.99999999999998579, 7.561388982944274417 ) ) ;
#9346=CARTESIAN_POINT ( 'NONE',  ( -9.295050272127044266, 37.47773437608393010, 9.295050272127047819 ) ) ;
#9351=CARTESIAN_POINT ( 'NONE',  ( 143.5748159460630688, 40.60312499999999858, -1.662435489736055892E-15 ) ) ;
#9352=CARTESIAN_POINT ( 'NONE',  ( 116.4251840539369596, 34.64999999999999147, 0.000000000000000000 ) ) ;
#9353=EDGE_CURVE ( 'NONE', #21949, #26975, #14001, .T. ) ;
#9358=CARTESIAN_POINT ( 'NONE',  ( 139.2950502721270425, 34.69960937608393436, -9.295050272127046043 ) ) ;
#9359=CARTESIAN_POINT ( 'NONE',  ( 74.29505027212704249, 38.66835937608393436, -9.295050272127046043 ) ) ;
#9360=CARTESIAN_POINT ( 'NONE',  ( 9.598844408820456309, 37.62656250216787157, -9.598844408820458085 ) ) ;
#9361=CARTESIAN_POINT ( 'NONE',  ( -9.598844408820458085, 33.85625000216787583, -9.598844408820458085 ) ) ;
#9365=CARTESIAN_POINT ( 'NONE',  ( 204.2950502721270425, 35.29492187608393294, 9.295050272127046043 ) ) ;
#9366=CARTESIAN_POINT ( 'NONE',  ( 185.8198241863519797, 55.00000000000000000, -10.00000000000000000 ) ) ;
#9378=CARTESIAN_POINT ( 'NONE',  ( 103.1528011352953342, 83.81250000136560629, 3.152801135295355106 ) ) ;
#9379=CARTESIAN_POINT ( 'NONE',  ( 51.85481384221820633, 32.61601562608393579, 0.000000000000000000 ) ) ;
#9384=CARTESIAN_POINT ( 'NONE',  ( 13.57481594606304576, 32.66562499999999858, -1.662435489736055892E-15 ) ) ;
#9385=CARTESIAN_POINT ( 'NONE',  ( 124.5550856135277087, 38.22187500108393010, -13.14518615778179900 ) ) ;
#9386=EDGE_CURVE ( 'NONE', #4933, #3340, #17333, .T. ) ;
#9388=CARTESIAN_POINT ( 'NONE',  ( 94.99999999999995737, 80.93750000000000000, -2.071067811865491048 ) ) ;
#9390=CARTESIAN_POINT ( 'NONE',  ( 103.5355339059327093, 79.75000000273119838, -3.535533905932755072 ) ) ;
#9392=CARTESIAN_POINT ( 'NONE',  ( 74.59884440882045453, 39.80937500216786873, 9.598844408820456309 ) ) ;
#9394=CARTESIAN_POINT ( 'NONE',  ( 71.94442362476911512, 31.75150628229955529, -11.16113343896966370 ) ) ;
#9398=ORIENTED_EDGE ( 'NONE', *, *, #16018, .T. ) ;
#9400=CARTESIAN_POINT ( 'NONE',  ( 200.6228728715778686, 34.99726562716787726, 13.57481594606304576 ) ) ;
#9404=CARTESIAN_POINT ( 'NONE',  ( 130.0000000000000000, 52.00000000000000711, -1.503427012513233026E-14 ) ) ;
#9405=CARTESIAN_POINT ( 'NONE',  ( -13.14518615778179189, 36.03906250108394005, 5.444914386472304635 ) ) ;
#9413=DIRECTION ( 'NONE',  ( -0.000000000000000000, -1.000000000000000000, -0.000000000000000000 ) ) ;
#9417=CARTESIAN_POINT ( 'NONE',  ( 103.5355339059327093, 83.75000000273119838, -3.535533905932755072 ) ) ;
#9419=CARTESIAN_POINT ( 'NONE',  ( -5.444914386472299306, 33.75703125108393721, 13.14518615778179722 ) ) ;
#9420=ORIENTED_EDGE ( 'NONE', *, *, #27379, .T. ) ;
#9423=CARTESIAN_POINT ( 'NONE',  ( -5.622872871577920151, 36.38632812499999858, 13.57481594606300135 ) ) ;
#9424=CARTESIAN_POINT ( 'NONE',  ( 204.2950502721270425, 35.29492187608393294, 9.295050272127046043 ) ) ;
#9425=VERTEX_POINT ( 'NONE', #23618 ) ;
#9429=EDGE_CURVE ( 'NONE', #16918, #23612, #24961, .T. ) ;
#9435=CARTESIAN_POINT ( 'NONE',  ( 120.7049497278729575, 36.68398437608392726, 9.295050272127047819 ) ) ;
#9436=CARTESIAN_POINT ( 'NONE',  ( 2.414731522848535132E-15, 39.36289062608393152, 13.14518615778179544 ) ) ;
#9437=CARTESIAN_POINT ( 'NONE',  ( 13.14518615778179900, 35.34453125108392868, 5.444914386472293977 ) ) ;
#9439=AXIS2_PLACEMENT_3D ( 'NONE', #21406, #6283, #22208 ) ;
#9440=CARTESIAN_POINT ( 'NONE',  ( 55.81982418635199394, 50.00000000000000000, -9.999999999999985789 ) ) ;
#9442=CARTESIAN_POINT ( 'NONE',  ( 185.7049497278729575, 31.92148437608393508, -9.295050272127046043 ) ) ;
#9443=ORIENTED_EDGE ( 'NONE', *, *, #21801, .F. ) ;
#9444=CARTESIAN_POINT ( 'NONE',  ( 71.35193222877107644, 36.00000000000000711, 11.61660627739524365 ) ) ;
#9447=CARTESIAN_POINT ( 'NONE',  ( 74.29505027212704249, 37.87460937608393152, -9.295050272127046043 ) ) ;
#9449=LINE ( 'NONE', #3188, #3787 ) ;
#9450=CARTESIAN_POINT ( 'NONE',  ( 195.0000000000000000, 36.78320312608393294, 13.14518615778179544 ) ) ;
#9454=CARTESIAN_POINT ( 'NONE',  ( 204.2950502721270425, 37.87460937608393863, 9.295050272127046043 ) ) ;
#9460=CARTESIAN_POINT ( 'NONE',  ( 130.0000000000000000, 32.21914062608393436, 13.14518615778179544 ) ) ;
#9461=CARTESIAN_POINT ( 'NONE',  ( 55.70494972787295751, 31.92148437608393508, 9.295050272127047819 ) ) ;
#9462=CARTESIAN_POINT ( 'NONE',  ( 208.1451861577817795, 35.64218750108393152, -5.444914386472297529 ) ) ;
#9465=CARTESIAN_POINT ( 'NONE',  ( 5.365496568045275971, 54.48174559707876341, -15.00000000000000000 ) ) ;
#9466=( BOUNDED_SURFACE ( )  B_SPLINE_SURFACE ( 3, 2, ( 
 ( #20598, #1224, #26880 ),
 ( #16446, #14016, #5066 ),
 ( #3346, #18460, #2919 ),
 ( #22740, #27166, #22452 ),
 ( #7619, #5490, #9465 ),
 ( #7325, #15874, #5207 ),
 ( #11449, #12016, #18598 ),
 ( #14159, #20170, #20739 ),
 ( #27302, #7760, #25142 ),
 ( #5633, #652, #9325 ),
 ( #18021, #13871, #21149 ),
 ( #27572, #12711, #4048 ),
 ( #5912, #25839, #23015 ),
 ( #3903, #21017, #6179 ),
 ( #16589, #8307, #8032 ),
 ( #10439, #1496, #12151 ),
 ( #27431, #1633, #19146 ),
 ( #10152, #6314, #16730 ),
 ( #18863, #14847, #1915 ),
 ( #10580, #8174, #25697 ) ),
 .UNSPECIFIED., .F., .F., .F. ) 
 B_SPLINE_SURFACE_WITH_KNOTS ( ( 4, 2, 2, 2, 2, 2, 2, 2, 2, 4 ),
 ( 3, 3 ),
 ( 0.009073803551359463371, 0.01139250602759181788, 0.01371120850382417065, 0.01602991098005652343, 0.01834861345628887794, 0.01950796469440505693, 0.02066731593252123245, 0.02298601840875358349, 0.02530472088498593800, 0.02762342336121829250 ),
 ( 0.000000000000000000, 1.000000000000000000 ),
 .UNSPECIFIED. ) 
 GEOMETRIC_REPRESENTATION_ITEM ( )  RATIONAL_B_SPLINE_SURFACE ( (
 ( 1.000000000000000000, 0.7071067811865473507, 1.000000000000000000),
 ( 1.000000000000000000, 0.7344871497829210671, 1.000000000000000000),
 ( 1.000000000000000000, 0.7612510203318444413, 1.000000000000000000),
 ( 1.000000000000000000, 0.8116663633844437564, 1.000000000000000000),
 ( 1.000000000000000000, 0.8353358059750773945, 1.000000000000000000),
 ( 1.000000000000000000, 0.8764699612587100175, 1.000000000000000000),
 ( 1.000000000000000000, 0.8939017358719162365, 1.000000000000000000),
 ( 1.000000000000000000, 0.9185314935647118650, 1.000000000000000000),
 ( 1.000000000000000000, 0.9256439951239471275, 1.000000000000000000),
 ( 1.000000000000000000, 0.9261623622476505835, 1.000000000000000000),
 ( 1.000000000000000000, 0.9246301385978624721, 1.000000000000000000),
 ( 1.000000000000000000, 0.9183304321348235710, 1.000000000000000000),
 ( 1.000000000000000000, 0.9135987334168408358, 1.000000000000000000),
 ( 1.000000000000000000, 0.8954110486039673633, 1.000000000000000000),
 ( 1.000000000000000000, 0.8779877431163967128, 1.000000000000000000),
 ( 1.000000000000000000, 0.8366182664709538308, 1.000000000000000000),
 ( 1.000000000000000000, 0.8126941604019177756, 1.000000000000000000),
 ( 1.000000000000000000, 0.7617527316302064033, 1.000000000000000000),
 ( 1.000000000000000000, 0.7347103785794923958, 1.000000000000000000),
 ( 1.000000000000000000, 0.7071067811865462405, 1.000000000000000000) ) ) 
 REPRESENTATION_ITEM ( '' )  SURFACE ( )  );
#9467=ADVANCED_FACE ( 'NONE', ( #23893 ), #26027, .F. ) ;
#9468=CARTESIAN_POINT ( 'NONE',  ( 143.5748159460630404, 37.47773437716787726, 5.622872871577869525 ) ) ;
#9470=ADVANCED_FACE ( 'NONE', ( #17467 ), #10904, .T. ) ;
#9473=CARTESIAN_POINT ( 'NONE',  ( 208.1451861577817795, 40.40468750108393436, -5.444914386472297529 ) ) ;
#9474=VERTEX_POINT ( 'NONE', #8644 ) ;
#9477=CARTESIAN_POINT ( 'NONE',  ( -4.972887739508807137, 36.00000000000002842, -12.48139679469879582 ) ) ;
#9479=CARTESIAN_POINT ( 'NONE',  ( 208.5748159460630688, 38.22187499999999716, -1.662435489736055892E-15 ) ) ;
#9480=ADVANCED_FACE ( 'NONE', ( #6778 ), #234, .F. ) ;
#9482=CARTESIAN_POINT ( 'NONE',  ( -11.26481880218186227, 36.00000000000000000, 6.828991891054477570 ) ) ;
#9485=CARTESIAN_POINT ( 'NONE',  ( -9.598844408820458085, 39.41250000216787441, -9.598844408820458085 ) ) ;
#9487=CARTESIAN_POINT ( 'NONE',  ( 204.1801758136479918, 55.00000000000000000, -15.00000000000000000 ) ) ;
#9488=CARTESIAN_POINT ( 'NONE',  ( -2.169956583105884018, 49.99999999883904422, 13.43548448457833366 ) ) ;
#9490=CARTESIAN_POINT ( 'NONE',  ( 139.5988444088204687, 34.94765624999999432, 9.598844408820456309 ) ) ;
#9492=ORIENTED_EDGE ( 'NONE', *, *, #14367, .T. ) ;
#9493=CARTESIAN_POINT ( 'NONE',  ( -20.00000000000000355, 55.00000000000000000, -14.99999999999999822 ) ) ;
#9497=CARTESIAN_POINT ( 'NONE',  ( 120.7049497278729575, 34.10429687608393579, -9.295050272127046043 ) ) ;
#9498=CARTESIAN_POINT ( 'NONE',  ( 68.87838541077974241, 31.34156310770110565, -13.57481594606304931 ) ) ;
#9501=CARTESIAN_POINT ( 'NONE',  ( -8.049105076161786076E-16, 39.56132812608393579, -13.14518615778179544 ) ) ;
#9507=VECTOR ( 'NONE', #6805, 1000.000000000000000 ) ;
#9513=CYLINDRICAL_SURFACE ( 'NONE', #20999, 5.000000000000000888 ) ;
#9514=ORIENTED_EDGE ( 'NONE', *, *, #22631, .T. ) ;
#9515=( BOUNDED_CURVE ( )  B_SPLINE_CURVE ( 2, ( #24514, #2296, #292, #15229, #23947, #15373, #15521, #13081, #26374 ),
 .UNSPECIFIED., .F., .T. ) 
 B_SPLINE_CURVE_WITH_KNOTS ( ( 3, 2, 2, 2, 3 ),
 ( 0.1041666666666664909, 0.1145833333333332732, 0.1250000000000000833, 0.1354166666666668517, 0.1458333333333336757 ),
 .UNSPECIFIED. ) 
 CURVE ( )  GEOMETRIC_REPRESENTATION_ITEM ( )  RATIONAL_B_SPLINE_CURVE ( ( 1.000000000000001332, 0.9238795325112854062, 1.000000000000000000, 0.9238795325112867385, 1.000000000000000000, 0.9238795325112867385, 1.000000000000000000, 0.9238795325112842960, 1.000000000000002442 ) ) 
 REPRESENTATION_ITEM ( '' )  );
#9517=CARTESIAN_POINT ( 'NONE',  ( 204.5988444088204687, 39.01562500216787299, 9.598844408820456309 ) ) ;
#9524=DIRECTION ( 'NONE',  ( 0.000000000000000000, -1.000000000000000000, 0.000000000000000000 ) ) ;
#9526=CARTESIAN_POINT ( 'NONE',  ( 70.44491438647230552, 32.07031250108393294, 13.14518615778179189 ) ) ;
#9531=CARTESIAN_POINT ( 'NONE',  ( -13.57481594606304576, 33.85624999999999574, 0.000000000000000000 ) ) ;
#9532=CARTESIAN_POINT ( 'NONE',  ( 130.0000000000000000, 34.99726562608393721, -13.14518615778179544 ) ) ;
#9534=CARTESIAN_POINT ( 'NONE',  ( 94.99999999999995737, 82.06250000000001421, 2.071067811865466624 ) ) ;
#9537=CARTESIAN_POINT ( 'NONE',  ( 96.84719886470459471, 82.56250000136559208, 3.152801135295355994 ) ) ;
#9539=CARTESIAN_POINT ( 'NONE',  ( 65.00000000000000000, 38.91640625216786731, 13.57481594606304576 ) ) ;
#9541=CARTESIAN_POINT ( 'NONE',  ( 78.57481594606304043, 40.65273437499998721, -5.622872871577873077 ) ) ;
#9542=CARTESIAN_POINT ( 'NONE',  ( 9.598844408820456309, 37.62656250216787157, -9.598844408820458085 ) ) ;
#9546=ORIENTED_EDGE ( 'NONE', *, *, #6239, .T. ) ;
#9548=CARTESIAN_POINT ( 'NONE',  ( 181.4251840539369596, 31.62382812716787228, 5.622872871577880183 ) ) ;
#9552=CARTESIAN_POINT ( 'NONE',  ( 204.5988444088204687, 38.22187500216787015, 9.598844408820456309 ) ) ;
#9553=CARTESIAN_POINT ( 'NONE',  ( -13.14518615778179900, 34.35234375108393579, -5.444914386472297529 ) ) ;
#9554=CARTESIAN_POINT ( 'NONE',  ( 130.0000000000000000, 32.02070312608393010, 13.14518615778179544 ) ) ;
#9555=CARTESIAN_POINT ( 'NONE',  ( 51.42518405393695957, 33.01289062500000426, -5.622872871577873077 ) ) ;
#9556=FACE_OUTER_BOUND ( 'NONE', #23488, .T. ) ;
#9565=CARTESIAN_POINT ( 'NONE',  ( 13.14518615778179544, 34.00507812608393721, -1.609821015232357215E-15 ) ) ;
#9567=CARTESIAN_POINT ( 'NONE',  ( 0.000000000000000000, -7.395377635281828788, 0.000000000000000000 ) ) ;
#9570=CARTESIAN_POINT ( 'NONE',  ( 185.7049497278729575, 35.69179687608393436, -9.295050272127046043 ) ) ;
#9572=CARTESIAN_POINT ( 'NONE',  ( 2.493653234604083739E-15, 37.22968749999999716, 13.57481594606304576 ) ) ;
#9574=VECTOR ( 'NONE', #16646, 1000.000000000000227 ) ;
#9575=EDGE_LOOP ( 'NONE', ( #4212, #7319, #13144, #15480 ) ) ;
#9579=LINE ( 'NONE', #5319, #11202 ) ;
#9580=CARTESIAN_POINT ( 'NONE',  ( 143.1451861577818079, 37.72578125108393721, 5.444914386472293977 ) ) ;
#9581=CARTESIAN_POINT ( 'NONE',  ( -5.444914386472297529, 39.01562500108394005, -13.14518615778179722 ) ) ;
#9582=CARTESIAN_POINT ( 'NONE',  ( 9.295050272127047819, 34.50117187608393010, 9.295050272127046043 ) ) ;
#9584=CARTESIAN_POINT ( 'NONE',  ( 68.71653411378430576, 51.46663580899353008, -14.99999999999931966 ) ) ;
#9590=CARTESIAN_POINT ( 'NONE',  ( 51.85481384221820633, 37.37851562608393863, 0.000000000000000000 ) ) ;
#9598=CARTESIAN_POINT ( 'NONE',  ( 208.1451861577818079, 38.71796875108393721, 5.444914386472293977 ) ) ;
#9600=EDGE_LOOP ( 'NONE', ( #27164, #22842, #16874, #3912, #14373 ) ) ;
#9604=ORIENTED_EDGE ( 'NONE', *, *, #5841, .F. ) ;
#9605=CARTESIAN_POINT ( 'NONE',  ( 116.8548138422182205, 32.81445312608393294, 0.000000000000000000 ) ) ;
#9606=CARTESIAN_POINT ( 'NONE',  ( 65.00000000000000000, 32.02070312608393010, 13.14518615778179544 ) ) ;
#9607=CARTESIAN_POINT ( 'NONE',  ( 195.0000000000000000, 34.60039062608393579, 13.14518615778179544 ) ) ;
#9608=ORIENTED_EDGE ( 'NONE', *, *, #13839, .F. ) ;
#9612=CARTESIAN_POINT ( 'NONE',  ( 143.5748159460630688, 37.52734375216787299, -1.662435489736055892E-15 ) ) ;
#9614=CARTESIAN_POINT ( 'NONE',  ( 65.00000000000000000, 50.00000000000000000, 13.57481594606303688 ) ) ;
#9616=CARTESIAN_POINT ( 'NONE',  ( 69.85849929045953388, 49.99999999891532099, 12.70434618649044189 ) ) ;
#9621=CARTESIAN_POINT ( 'NONE',  ( -6.470563696665745823, 36.00000000000002132, -11.78199955157067080 ) ) ;
#9625=CARTESIAN_POINT ( 'NONE',  ( 71.94442639331153089, 31.75150625057403175, -11.16113171639042356 ) ) ;
#9628=CARTESIAN_POINT ( 'NONE',  ( 195.0000000000000000, 38.02343749999999289, 13.57481594606304576 ) ) ;
#9630=CARTESIAN_POINT ( 'NONE',  ( 4.858499290463564435, 49.99999999891551994, 12.70434618648897818 ) ) ;
#9632=CARTESIAN_POINT ( 'NONE',  ( 130.0000000000000000, 33.26093749999999716, 13.57481594606304576 ) ) ;
#9640=CARTESIAN_POINT ( 'NONE',  ( 116.8548138422182205, 33.40976562608393863, 0.000000000000000000 ) ) ;
#9641=CARTESIAN_POINT ( 'NONE',  ( 74.29505027212704249, 40.05742187608392868, 9.295050272127046043 ) ) ;
#9643=CARTESIAN_POINT ( 'NONE',  ( -8.049105076161786076E-16, 38.76757812608393294, -13.14518615778179544 ) ) ;
#9645=CARTESIAN_POINT ( 'NONE',  ( 181.9416181435491637, 36.00000000000000711, 1.569311539113946274 ) ) ;
#9648=CARTESIAN_POINT ( 'NONE',  ( 185.7049497278729575, 32.51679687608393721, -9.295050272127046043 ) ) ;
#9649=LINE ( 'NONE', #4826, #24289 ) ;
#9653=EDGE_CURVE ( 'NONE', #3976, #1420, #25612, .T. ) ;
#9655=DIRECTION ( 'NONE',  ( -0.000000000000000000, 1.000000000000000000, -0.000000000000000000 ) ) ;
#9663=CARTESIAN_POINT ( 'NONE',  ( 96.84719886470459471, 83.31250000136560629, -3.152801135295383084 ) ) ;
#9664=CARTESIAN_POINT ( 'NONE',  ( 74.29505027212704249, 33.90585937608393152, -9.295050272127046043 ) ) ;
#9666=DIRECTION ( 'NONE',  ( -1.000000000000000000, 0.000000000000000000, 7.228014483236696740E-18 ) ) ;
#9668=CARTESIAN_POINT ( 'NONE',  ( 124.3771271284220319, 37.77539062716787299, -13.57481594606295339 ) ) ;
#9669=CARTESIAN_POINT ( 'NONE',  ( 13.57481594606304753, 34.30273437500000000, -5.622872871577873077 ) ) ;
#9671=CARTESIAN_POINT ( 'NONE',  ( 135.4449143864723055, 33.06250000108393294, 13.14518615778179189 ) ) ;
#9672=ORIENTED_EDGE ( 'NONE', *, *, #17170, .F. ) ;
#9673=CARTESIAN_POINT ( 'NONE',  ( 104.9999999999999574, 81.56250000000002842, -2.071067811865491937 ) ) ;
#9674=EDGE_CURVE ( 'NONE', #8206, #3171, #3453, .T. ) ;
#9675=CARTESIAN_POINT ( 'NONE',  ( 78.57481594606305464, 38.27148437716787299, 5.622872871577868636 ) ) ;
#9676=CARTESIAN_POINT ( 'NONE',  ( 104.4587341249999781, 83.00000000136559208, -1.846868145590750299 ) ) ;
#9678=CARTESIAN_POINT ( 'NONE',  ( 208.5748159460630688, 37.37851562499999858, 5.622872871577868636 ) ) ;
#9681=CARTESIAN_POINT ( 'NONE',  ( 208.1451861577818079, 39.56132812608393579, -1.609821015232357215E-15 ) ) ;
#9682=CARTESIAN_POINT ( 'NONE',  ( -8.312177448680279460E-16, 37.72578125216787726, -13.57481594606304576 ) ) ;
#9684=CARTESIAN_POINT ( 'NONE',  ( 183.0647576233092195, 35.99999999999999289, -5.809862729997679054 ) ) ;
#9685=AXIS2_PLACEMENT_3D ( 'NONE', #23647, #4122, #7840 ) ;
#9687=EDGE_CURVE ( 'NONE', #2214, #144, #14422, .T. ) ;
#9689=( BOUNDED_CURVE ( )  B_SPLINE_CURVE ( 2, ( #3873, #21120, #23540, #21263, #19392, #19117, #18974, #2017, #3739, #1886, #25808, #20987, #8001, #12818, #1745, #21541, #23266, #1468, #25952, #27824, #14960, #25400, #6284, #8278, #16969, #8414, #14816, #23680, #3603, #21407, #19258, #10124, #28097, #27682, #4016, #14550, #12682, #25668, #18837, #17104, #10550, #16702, #6150, #8145, #4157, #10685, #8560, #17251, #14412, #5881, #12262, #27544, #12399, #16839, #25536, #6016, #14679, #23400, #13234, #11105, #15382, #19966, #6839, #4437, #9266, #26384, #17962, #11247, #15676, #6426, #12951, #19675, #19819, #302, #22250, #23957, #9127, #443, #10964, #8988, #15095, #4865, #19536, #6980, #24237, #21685, #4720, #18, #13089, #2160, #17820, #26525, #24097, #4573, #21829, #23815, #17394 ),
 .UNSPECIFIED., .F., .F. ) 
 B_SPLINE_CURVE_WITH_KNOTS ( ( 3, 2, 2, 2, 2, 2, 2, 2, 2, 2, 2, 2, 2, 2, 2, 2, 2, 2, 2, 2, 2, 2, 2, 2, 2, 2, 2, 2, 2, 2, 2, 2, 2, 2, 2, 2, 2, 2, 2, 2, 2, 2, 2, 2, 2, 2, 2, 2, 3 ),
 ( 0.000000000000000000, 0.01041666666666666609, 0.02083333333333333218, 0.03125000000000000000, 0.04166666666666666435, 0.05208333333333333565, 0.06250000000000000000, 0.07291666666666667129, 0.08333333333333332871, 0.09374999999999998612, 0.1041666666666666713, 0.1145833333333333287, 0.1250000000000000000, 0.1354166666666666574, 0.1458333333333333426, 0.1562500000000000000, 0.1666666666666666574, 0.1770833333333333426, 0.1874999999999999722, 0.1979166666666666574, 0.2083333333333333426, 0.2187500000000000000, 0.2291666666666666574, 0.2395833333333333426, 0.2500000000000000000, 0.2604166666666666852, 0.2708333333333333148, 0.2812500000000000000, 0.2916666666666666852, 0.3020833333333333148, 0.3125000000000000000, 0.3229166666666666852, 0.3333333333333333148, 0.3437500000000000000, 0.3541666666666666852, 0.3645833333333333148, 0.3749999999999999445, 0.3854166666666666852, 0.3958333333333333148, 0.4062500000000000000, 0.4166666666666666852, 0.4270833333333333148, 0.4375000000000000000, 0.4479166666666666852, 0.4583333333333333148, 0.4687500000000000000, 0.4791666666666666852, 0.4895833333333333148, 0.4988304892921909817 ),
 .UNSPECIFIED. ) 
 CURVE ( )  GEOMETRIC_REPRESENTATION_ITEM ( )  RATIONAL_B_SPLINE_CURVE ( ( 1.000000000000000000, 0.9238795325112867385, 1.000000000000000000, 0.9238795325112867385, 1.000000000000000000, 0.9238795325112867385, 1.000000000000000000, 0.9238795325112867385, 1.000000000000000000, 0.9238795325112867385, 1.000000000000000000, 0.9238795325112867385, 1.000000000000000000, 0.9238795325112867385, 1.000000000000000000, 0.9238795325112867385, 1.000000000000000000, 0.9238795325112867385, 1.000000000000000000, 0.9238795325112867385, 1.000000000000000000, 0.9238795325112867385, 1.000000000000000000, 0.9238795325112867385, 1.000000000000000000, 0.9238795325112867385, 1.000000000000000000, 0.9238795325112867385, 1.000000000000000000, 0.9238795325112867385, 1.000000000000000000, 0.9238795325112867385, 1.000000000000000000, 0.9238795325112867385, 1.000000000000000000, 0.9238795325112867385, 1.000000000000000000, 0.9238795325112867385, 1.000000000000000000, 0.9238795325112867385, 1.000000000000000000, 0.9238795325112867385, 1.000000000000000000, 0.9238795325112867385, 1.000000000000000000, 0.9238795325112867385, 1.000000000000000000, 0.9238795325112867385, 1.000000000000000000, 0.9238795325112867385, 1.000000000000000000, 0.9238795325112867385, 1.000000000000000000, 0.9238795325112867385, 1.000000000000000000, 0.9238795325112867385, 1.000000000000000000, 0.9238795325112867385, 1.000000000000000000, 0.9238795325112867385, 1.000000000000000000, 0.9238795325112867385, 1.000000000000000000, 0.9238795325112867385, 1.000000000000000000, 0.9238795325112867385, 1.000000000000000000, 0.9238795325112867385, 1.000000000000000000, 0.9238795325112867385, 1.000000000000000000, 0.9238795325112867385, 1.000000000000000000, 0.9238795325112867385, 1.000000000000000000, 0.9238795325112867385, 1.000000000000000000, 0.9238795325112867385, 1.000000000000000000, 0.9238795325112867385, 1.000000000000000000, 0.9238795325112867385, 1.000000000000000000, 0.9238795325112867385, 1.000000000000000000, 0.9238795325112867385, 1.000000000000000000, 0.9238795325112867385, 1.000000000000000000, 0.9238795325112867385, 1.000000000000000000, 0.9238795325112867385, 1.000000000000000000, 0.9238795325112867385, 1.000000000000000000, 0.9324258078851886955, 0.9848264816800353927 ) ) 
 REPRESENTATION_ITEM ( '' )  );
#9691=CARTESIAN_POINT ( 'NONE',  ( 208.5748159460630688, 31.97109375216787441, -1.662435489736055892E-15 ) ) ;
#9695=CARTESIAN_POINT ( 'NONE',  ( -9.295050272127044266, 32.11992187608393579, 9.295050272127047819 ) ) ;
#9696=CARTESIAN_POINT ( 'NONE',  ( 124.5550856135277087, 31.67343750108393863, -13.14518615778179900 ) ) ;
#9702=CARTESIAN_POINT ( 'NONE',  ( 70.44491438647230552, 40.30546875108393579, -13.14518615778179900 ) ) ;
#9708=CARTESIAN_POINT ( 'NONE',  ( 5.444914386472302859, 33.06250000108393294, 13.14518615778179189 ) ) ;
#9713=CARTESIAN_POINT ( 'NONE',  ( -9.598844408820458085, 36.13828124999999147, -9.598844408820458085 ) ) ;
#9714=EDGE_CURVE ( 'NONE', #9261, #7715, #6187, .T. ) ;
#9715=CARTESIAN_POINT ( 'NONE',  ( 204.2950502721270425, 34.69960937608393436, -9.295050272127046043 ) ) ;
#9721=CARTESIAN_POINT ( 'NONE',  ( 195.0000000000000000, 39.71015625216787015, 13.57481594606304576 ) ) ;
#9723=CARTESIAN_POINT ( 'NONE',  ( 143.1451861577818079, 38.56914062608393579, -1.609821015232357215E-15 ) ) ;
#9724=CARTESIAN_POINT ( 'NONE',  ( 9.295050272127047819, 38.66835937608393436, 9.295050272127046043 ) ) ;
#9725=CARTESIAN_POINT ( 'NONE',  ( -9.295050272127046043, 40.65273437608393436, -9.295050272127046043 ) ) ;
#9727=CARTESIAN_POINT ( 'NONE',  ( -8.312177448680279460E-16, 36.13828125216787157, -13.57481594606304576 ) ) ;
#9729=DIRECTION ( 'NONE',  ( 0.000000000000000000, -1.000000000000000000, 0.000000000000000000 ) ) ;
#9732=CARTESIAN_POINT ( 'NONE',  ( 78.14518615778180788, 36.13828125108393152, 5.444914386472293977 ) ) ;
#9735=CARTESIAN_POINT ( 'NONE',  ( 195.0000000000000000, -7.395377635281828788, 13.57481594606302266 ) ) ;
#9739=CARTESIAN_POINT ( 'NONE',  ( 195.0000000000000000, 38.96601562608393721, -13.14518615778179544 ) ) ;
#9747=CARTESIAN_POINT ( 'NONE',  ( 200.4449143864723055, 34.65000000108393863, 13.14518615778179189 ) ) ;
#9751=CARTESIAN_POINT ( 'NONE',  ( 187.3760580380745466, 55.00000000000000711, 14.99999999999995559 ) ) ;
#9752=CARTESIAN_POINT ( 'NONE',  ( 143.5748159460630404, 38.37070312716786447, -5.622872871577873077 ) ) ;
#9755=CARTESIAN_POINT ( 'NONE',  ( 71.11984362770094492, 51.28708186914658995, 14.99999999999719513 ) ) ;
#9762=CARTESIAN_POINT ( 'NONE',  ( 136.4128666762518662, 50.00000000108477849, 11.99502265407748780 ) ) ;
#9763=CARTESIAN_POINT ( 'NONE',  ( -5.569058551903145471, 35.99999999999999289, 11.91493531101255599 ) ) ;
#9764=CARTESIAN_POINT ( 'NONE',  ( 55.70494972787295751, 32.91367187608393152, 9.295050272127047819 ) ) ;
#9767=CARTESIAN_POINT ( 'NONE',  ( 13.14518615778179722, 36.13828125108393152, 5.444914386472293977 ) ) ;
#9768=VECTOR ( 'NONE', #9223, 1000.000000000000000 ) ;
#9770=CARTESIAN_POINT ( 'NONE',  ( -0.8389268692817103412, 53.50081894914648473, 14.99999999999999645 ) ) ;
#9772=CARTESIAN_POINT ( 'NONE',  ( 124.3771271284221314, 34.79882812499998579, 13.57481594606304753 ) ) ;
#9773=ORIENTED_EDGE ( 'NONE', *, *, #19217, .T. ) ;
#9775=PLANE ( 'NONE',  #19019 ) ;
#9779=CARTESIAN_POINT ( 'NONE',  ( 135.4449143864723055, 40.20625000108394431, 13.14518615778179189 ) ) ;
#9780=CARTESIAN_POINT ( 'NONE',  ( 70.62287287157788285, 31.82226562716787654, 13.57481594606304576 ) ) ;
#9782=CARTESIAN_POINT ( 'NONE',  ( 5.622872871577786924, 37.37851562716787157, 13.57481594606313813 ) ) ;
#9783=CARTESIAN_POINT ( 'NONE',  ( 2.414731522848535132E-15, 37.57695312608392868, 13.14518615778179544 ) ) ;
#9785=CARTESIAN_POINT ( 'NONE',  ( 51.42518405393695957, 37.77539062499998579, -5.622872871577872189 ) ) ;
#9789=CARTESIAN_POINT ( 'NONE',  ( 208.5748159460630688, 40.60312499999999858, -1.662435489736055892E-15 ) ) ;
#9790=CARTESIAN_POINT ( 'NONE',  ( 214.9999999999999716, 50.00000000000000000, -10.00000000000000000 ) ) ;
#9794=DIRECTION ( 'NONE',  ( 1.000000000000000000, 0.000000000000000000, -7.228014483236696740E-18 ) ) ;
#9796=CARTESIAN_POINT ( 'NONE',  ( 130.0000000000000000, 38.42031249999999432, -13.57481594606304576 ) ) ;
#9801=CARTESIAN_POINT ( 'NONE',  ( 181.4251840539369596, 32.31835937499999289, 5.622872871577880183 ) ) ;
#9803=DIRECTION ( 'NONE',  ( -0.000000000000000000, 1.000000000000000000, -0.000000000000000000 ) ) ;
#9804=CARTESIAN_POINT ( 'NONE',  ( 99.99999999999995737, 84.18750000136560629, -4.458734125000016313 ) ) ;
#9805=CARTESIAN_POINT ( 'NONE',  ( 59.55508561352770158, 32.46718750108393436, -13.14518615778179900 ) ) ;
#9809=CARTESIAN_POINT ( 'NONE',  ( 120.4011555911795455, 37.82500000216787583, -9.598844408820458085 ) ) ;
#9810=CARTESIAN_POINT ( 'NONE',  ( -9.598844408820458085, 32.96328124999999432, -9.598844408820458085 ) ) ;
#9812=CARTESIAN_POINT ( 'NONE',  ( 116.8548138422182063, 34.45156250108394147, 5.444914386472304635 ) ) ;
#9814=CARTESIAN_POINT ( 'NONE',  ( 104.9999999999999574, 81.43750000000001421, 2.071067811865462627 ) ) ;
#9816=CARTESIAN_POINT ( 'NONE',  ( 101.8468681455906903, 82.12500000136560629, -4.458734125000016313 ) ) ;
#9820=CARTESIAN_POINT ( 'NONE',  ( 200.4449143864723055, 39.71015625108393010, -13.14518615778179900 ) ) ;
#9821=CARTESIAN_POINT ( 'NONE',  ( -13.57481594606304576, 40.30546875216787583, 0.000000000000000000 ) ) ;
#9826=CARTESIAN_POINT ( 'NONE',  ( 204.5988444088204403, 32.07031250216787299, -9.598844408820458085 ) ) ;
#9827=ADVANCED_FACE ( 'NONE', ( #26463, #22859 ), #16428, .F. ) ;
#9828=CARTESIAN_POINT ( 'NONE',  ( 5.622872871577870413, 36.88242187716787157, -13.57481594606304753 ) ) ;
#9833=CARTESIAN_POINT ( 'NONE',  ( 55.40115559117954547, 32.96328124999999432, -9.598844408820458085 ) ) ;
#9836=CARTESIAN_POINT ( 'NONE',  ( 65.00000000000000000, 36.53515625216787299, 13.57481594606304576 ) ) ;
#9843=CARTESIAN_POINT ( 'NONE',  ( 195.0000000000000000, 39.61093749999999147, 13.57481594606304576 ) ) ;
#9845=CARTESIAN_POINT ( 'NONE',  ( -9.295050272127044266, 32.11992187608393579, 9.295050272127047819 ) ) ;
#9846=EDGE_CURVE ( 'NONE', #9895, #439, #4043, .T. ) ;
#9847=ORIENTED_EDGE ( 'NONE', *, *, #6036, .T. ) ;
#9849=CARTESIAN_POINT ( 'NONE',  ( -9.598844408820454532, 37.92421874999999432, 9.598844408820459861 ) ) ;
#9850=( BOUNDED_SURFACE ( )  B_SPLINE_SURFACE ( 3, 2, ( 
 ( #4596, #24546, #13256 ),
 ( #11412, #2465, #611 ),
 ( #9287, #26692, #20416 ),
 ( #27264, #9987, #22843 ),
 ( #25245, #20979, #18418 ),
 ( #1459, #20564, #27124 ),
 ( #5735, #7720, #25108 ),
 ( #18561, #18828, #23119 ),
 ( #16412, #5872, #902 ),
 ( #7428, #3593, #12115 ),
 ( #20841, #16122, #11840 ),
 ( #16270, #24828, #16554 ),
 ( #14120, #12251, #5312 ),
 ( #18696, #7575, #22701 ),
 ( #25391, #20705, #1044 ),
 ( #14262, #22557, #10116 ),
 ( #24968, #3024, #14402 ),
 ( #5596, #3310, #22982 ),
 ( #27536, #7993, #3449 ),
 ( #5452, #16691, #18277 ) ),
 .UNSPECIFIED., .F., .F., .T. ) 
 B_SPLINE_SURFACE_WITH_KNOTS ( ( 4, 2, 2, 2, 2, 2, 2, 2, 2, 4 ),
 ( 3, 3 ),
 ( 0.009073803551359449493, 0.01139250602759181094, 0.01371120850382417239, 0.01602991098005653384, 0.01834861345628889528, 0.01950796469440507774, 0.02066731593252125673, 0.02298601840875361818, 0.02530472088498597616, 0.02762342336121833761 ),
 ( 0.000000000000000000, 1.000000000000000000 ),
 .UNSPECIFIED. ) 
 GEOMETRIC_REPRESENTATION_ITEM ( )  RATIONAL_B_SPLINE_SURFACE ( (
 ( 1.000000000000000000, 0.7071067811865470176, 1.000000000000000000),
 ( 1.000000000000000000, 0.7344871497831121365, 1.000000000000000000),
 ( 1.000000000000000000, 0.7612510203315883128, 1.000000000000000000),
 ( 1.000000000000000000, 0.8116663633847007731, 1.000000000000000000),
 ( 1.000000000000000000, 0.8353358059750350950, 1.000000000000000000),
 ( 1.000000000000000000, 0.8764699612587538713, 1.000000000000000000),
 ( 1.000000000000000000, 0.8939017358718743811, 1.000000000000000000),
 ( 1.000000000000000000, 0.9185314935647557189, 1.000000000000000000),
 ( 1.000000000000000000, 0.9256439951239916475, 1.000000000000000000),
 ( 1.000000000000000000, 0.9261623622476302664, 1.000000000000000000),
 ( 1.000000000000000000, 0.9246301385979071030, 1.000000000000000000),
 ( 1.000000000000000000, 0.9183304321347808274, 1.000000000000000000),
 ( 1.000000000000000000, 0.9135987334169072271, 1.000000000000000000),
 ( 1.000000000000000000, 0.8954110486038381334, 1.000000000000000000),
 ( 1.000000000000000000, 0.8779877431164831991, 1.000000000000000000),
 ( 1.000000000000000000, 0.8366182664708661232, 1.000000000000000000),
 ( 1.000000000000000000, 0.8126941604018734777, 1.000000000000000000),
 ( 1.000000000000000000, 0.7617527316302484808, 1.000000000000000000),
 ( 1.000000000000000000, 0.7347103785794607544, 1.000000000000000000),
 ( 1.000000000000000000, 0.7071067811865446862, 1.000000000000000000) ) ) 
 REPRESENTATION_ITEM ( '' )  SURFACE ( )  );
#9851=CARTESIAN_POINT ( 'NONE',  ( 181.8548138422182205, 33.40976562608393863, 0.000000000000000000 ) ) ;
#9852=VERTEX_POINT ( 'NONE', #20580 ) ;
#9853=AXIS2_PLACEMENT_3D ( 'NONE', #16032, #13890, #13608 ) ;
#9854=CARTESIAN_POINT ( 'NONE',  ( -13.57481594606304576, 37.03124999999999289, 0.000000000000000000 ) ) ;
#9860=VECTOR ( 'NONE', #8203, 1000.000000000000000 ) ;
#9861=CARTESIAN_POINT ( 'NONE',  ( 185.4011555911795597, 38.81718750216787583, 9.598844408820459861 ) ) ;
#9863=CARTESIAN_POINT ( 'NONE',  ( 5.444914386472297529, 38.91640625108393436, -13.14518615778179722 ) ) ;
#9864=CARTESIAN_POINT ( 'NONE',  ( -13.14518615778179900, 33.36015625108393579, -5.444914386472297529 ) ) ;
#9867=ADVANCED_FACE ( 'NONE', ( #16714 ), #26543, .T. ) ;
#9871=CARTESIAN_POINT ( 'NONE',  ( 103.1528011352953342, 84.31250000136560629, -3.152801135295383084 ) ) ;
#9872=CARTESIAN_POINT ( 'NONE',  ( 214.9999999999999716, 75.00000000000000000, 9.999999999999946709 ) ) ;
#9878=LINE ( 'NONE', #14569, #9999 ) ;
#9882=CARTESIAN_POINT ( 'NONE',  ( 208.5748159460630688, 37.57695312716787583, -5.622872871577873966 ) ) ;
#9883=CARTESIAN_POINT ( 'NONE',  ( 78.14518615778180788, 37.13046875108393863, 5.444914386472293977 ) ) ;
#9885=CARTESIAN_POINT ( 'NONE',  ( -5.622872871577816234, 39.26367187500000000, -13.57481594606310260 ) ) ;
#9890=ADVANCED_FACE ( 'NONE', ( #24925 ), #20227, .T. ) ;
#9891=CARTESIAN_POINT ( 'NONE',  ( 116.4251840539369596, 38.76757812716787299, 5.622872871577880183 ) ) ;
#9892=CARTESIAN_POINT ( 'NONE',  ( 59.37712712842223794, 40.15664062716787441, -13.57481594606315412 ) ) ;
#9894=CARTESIAN_POINT ( 'NONE',  ( 189.5550856135277229, 38.51953125108393294, 13.14518615778179722 ) ) ;
#9895=VERTEX_POINT ( 'NONE', #5411 ) ;
#9897=CARTESIAN_POINT ( 'NONE',  ( -13.09590655363597733, 36.00000000000000000, 1.137167824541468031 ) ) ;
#9898=CARTESIAN_POINT ( 'NONE',  ( 120.8198241863519939, 50.00000000000000000, 9.999999999999968026 ) ) ;
#9899=CARTESIAN_POINT ( 'NONE',  ( 95.54126587499996504, 84.37500000136563472, -1.846868145590750077 ) ) ;
#9900=CARTESIAN_POINT ( 'NONE',  ( 130.0000000000000000, 36.00000000000000000, -11.57481594606305997 ) ) ;
#9903=CARTESIAN_POINT ( 'NONE',  ( 9.432006169633215364, 36.00000000000001421, 9.391769196591040370 ) ) ;
#9905=CARTESIAN_POINT ( 'NONE',  ( 120.4011555911795455, 34.55078124999999289, -9.598844408820458085 ) ) ;
#9907=CARTESIAN_POINT ( 'NONE',  ( 104.9999999999999716, 84.56250000000002842, -2.071067811865491937 ) ) ;
#9911=CARTESIAN_POINT ( 'NONE',  ( 135.4449143864723055, 38.12265625108393152, -13.14518615778179900 ) ) ;
#9912=CARTESIAN_POINT ( 'NONE',  ( 51.85481384221820633, 39.75976562608393294, 0.000000000000000000 ) ) ;
#9913=CARTESIAN_POINT ( 'NONE',  ( 58.66170920764977126, 36.00000000000000000, 11.53992004314981656 ) ) ;
#9914=CARTESIAN_POINT ( 'NONE',  ( 13.14518615778179544, 38.56914062608393579, -1.609821015232357215E-15 ) ) ;
#9918=CARTESIAN_POINT ( 'NONE',  ( 195.0000000000000000, 32.02070312608393010, 13.14518615778179544 ) ) ;
#9921=VECTOR ( 'NONE', #10499, 1000.000000000000000 ) ;
#9923=CARTESIAN_POINT ( 'NONE',  ( 116.8508260188483234, 36.00000000000000000, -1.058935892997001416 ) ) ;
#9924=CARTESIAN_POINT ( 'NONE',  ( 195.0000000000000000, 36.00000000000000000, -2.255140518769849538E-14 ) ) ;
#9932=CARTESIAN_POINT ( 'NONE',  ( 202.1713912169989555, 31.99955315621561525, -11.52591757658528948 ) ) ;
#9935=CARTESIAN_POINT ( 'NONE',  ( 96.84719886470459471, 82.56250000136559208, 3.152801135295355994 ) ) ;
#9936=CARTESIAN_POINT ( 'NONE',  ( 51.85481384221820633, 31.87187500108393223, 5.444914386472304635 ) ) ;
#9938=FACE_OUTER_BOUND ( 'NONE', #10150, .T. ) ;
#9939=ORIENTED_EDGE ( 'NONE', *, *, #10358, .F. ) ;
#9943=CARTESIAN_POINT ( 'NONE',  ( 143.1451861577818079, 35.64218750108393152, -5.444914386472297529 ) ) ;
#9944=ORIENTED_EDGE ( 'NONE', *, *, #24476, .F. ) ;
#9947=CARTESIAN_POINT ( 'NONE',  ( 65.00000000000000000, 38.51953125216787299, -13.57481594606304576 ) ) ;
#9948=CARTESIAN_POINT ( 'NONE',  ( 95.54126587499995082, 83.37500000136563472, -1.846868145590750077 ) ) ;
#9949=CARTESIAN_POINT ( 'NONE',  ( 124.5550856135277087, 39.11484375108394573, 13.14518615778179722 ) ) ;
#9950=CARTESIAN_POINT ( 'NONE',  ( 195.0000000000000000, 37.22968749999999716, 13.57481594606304576 ) ) ;
#9951=CIRCLE ( 'NONE', #19971, 5.000000000000000000 ) ;
#9955=CARTESIAN_POINT ( 'NONE',  ( 9.598844408820456309, 39.21406250216787015, -9.598844408820458085 ) ) ;
#9960=CARTESIAN_POINT ( 'NONE',  ( 195.0000000000000000, 39.56132812608393579, -13.14518615778179544 ) ) ;
#9962=LINE ( 'NONE', #12498, #17444 ) ;
#9965=CARTESIAN_POINT ( 'NONE',  ( 2.414731522848535132E-15, 33.01289062608393721, 13.14518615778179544 ) ) ;
#9968=CARTESIAN_POINT ( 'NONE',  ( 204.2950502721270425, 32.31835937608393294, 9.295050272127046043 ) ) ;
#9977=DIRECTION ( 'NONE',  ( 0.000000000000000000, 0.000000000000000000, -1.000000000000000000 ) ) ;
#9980=CARTESIAN_POINT ( 'NONE',  ( -5.444914386472299306, 32.16953125108393152, 13.14518615778179722 ) ) ;
#9982=CARTESIAN_POINT ( 'NONE',  ( 98.15313185440925281, 82.50000000136560629, -4.458734125000016313 ) ) ;
#9985=CARTESIAN_POINT ( 'NONE',  ( 195.0000000000000000, 34.00507812608393721, -13.14518615778179544 ) ) ;
#9986=ORIENTED_EDGE ( 'NONE', *, *, #3286, .F. ) ;
#9987=CARTESIAN_POINT ( 'NONE',  ( 201.9023785737630590, 51.13402819307176372, -15.00000000000129852 ) ) ;
#9992=CARTESIAN_POINT ( 'NONE',  ( -8.312177448680279460E-16, 36.13828125216787157, -13.57481594606304576 ) ) ;
#9993=CIRCLE ( 'NONE', #10434, 4.999999999999997335 ) ;
#9994=B_SPLINE_CURVE_WITH_KNOTS ( 'NONE', 3,
 ( #21144, #1631, #25560, #6041, #23704, #15264, #17559, #21854, #12842, #10986, #21569, #25836, #23841, #13403, #10577, #2044, #10848, #8446 ),
 .UNSPECIFIED., .F., .F.,
 ( 4, 2, 2, 2, 2, 2, 2, 2, 4 ),
 ( 0.000000000000000000, 0.004618502246277155811, 0.006927753369415732415, 0.009237004492554308152, 0.01039163005412361424, 0.01154625561569292379, 0.01385550673883149432, 0.01616475786197006659, 0.01847400898510864059 ),
 .UNSPECIFIED. ) ;
#9995=CARTESIAN_POINT ( 'NONE',  ( -13.14518615778179722, 37.52734375108393294, -5.444914386472297529 ) ) ;
#9996=CARTESIAN_POINT ( 'NONE',  ( -9.295050272127044266, 31.92148437608393508, 9.295050272127047819 ) ) ;
#9999=VECTOR ( 'NONE', #24998, 1000.000000000000000 ) ;
#10003=CARTESIAN_POINT ( 'NONE',  ( 95.54126587499996504, 84.68750000136560629, -1.387778780781445676E-14 ) ) ;
#10007=VERTEX_POINT ( 'NONE', #10211 ) ;
#10009=( BOUNDED_CURVE ( )  B_SPLINE_CURVE ( 2, ( #18140, #26853, #7301, #24702, #5182, #13845, #25119, #16282, #9727 ),
 .UNSPECIFIED., .F., .F. ) 
 B_SPLINE_CURVE_WITH_KNOTS ( ( 3, 2, 2, 2, 3 ),
 ( 0.3958333333333331483, 0.4062499999999999445, 0.4166666666666667407, 0.4270833333333335369, 0.4375000000000003331 ),
 .UNSPECIFIED. ) 
 CURVE ( )  GEOMETRIC_REPRESENTATION_ITEM ( )  RATIONAL_B_SPLINE_CURVE ( ( 1.000000000000001110, 0.9238795325112855172, 1.000000000000000000, 0.9238795325112867385, 1.000000000000000000, 0.9238795325112867385, 1.000000000000000000, 0.9238795325112842960, 1.000000000000002442 ) ) 
 REPRESENTATION_ITEM ( '' )  );
#10011=EDGE_CURVE ( 'NONE', #7715, #5951, #1247, .T. ) ;
#10016=CARTESIAN_POINT ( 'NONE',  ( 116.4251840539369596, 39.46210937716787726, -5.622872871577872189 ) ) ;
#10018=CARTESIAN_POINT ( 'NONE',  ( 55.70494972787295751, 38.27148437608393294, -9.295050272127046043 ) ) ;
#10021=CYLINDRICAL_SURFACE ( 'NONE', #8939, 13.57481594606304398 ) ;
#10025=EDGE_CURVE ( 'NONE', #26363, #13933, #9951, .T. ) ;
#10026=CARTESIAN_POINT ( 'NONE',  ( 120.4011555911795455, 38.02343750216788010, 9.598844408820459861 ) ) ;
#10027=CARTESIAN_POINT ( 'NONE',  ( 181.8548138422182205, 40.65273437608393436, 0.000000000000000000 ) ) ;
#10029=CARTESIAN_POINT ( 'NONE',  ( 185.7049497278729575, 39.26367187608393294, 9.295050272127047819 ) ) ;
#10034=CYLINDRICAL_SURFACE ( 'NONE', #17423, 13.57481594606304398 ) ;
#10036=SURFACE_SIDE_STYLE ('',( #23031 ) ) ;
#10038=CARTESIAN_POINT ( 'NONE',  ( 97.92893218813445344, 81.18750000000001421, 4.999999999999948486 ) ) ;
#10039=CARTESIAN_POINT ( 'NONE',  ( 12.66784425494550703, 36.00000000000000711, 4.396229039744191880 ) ) ;
#10040=FACE_OUTER_BOUND ( 'NONE', #2457, .T. ) ;
#10043=ORIENTED_EDGE ( 'NONE', *, *, #11067, .T. ) ;
#10049=CARTESIAN_POINT ( 'NONE',  ( 139.2950502721270425, 40.45429687608393721, -9.295050272127046043 ) ) ;
#10050=CARTESIAN_POINT ( 'NONE',  ( 70.44491438647230552, 36.03906250108394005, 13.14518615778179189 ) ) ;
#10053=CARTESIAN_POINT ( 'NONE',  ( 9.295050272127046043, 37.87460937608393152, -9.295050272127046043 ) ) ;
#10056=CARTESIAN_POINT ( 'NONE',  ( 97.92893218813446765, 82.18750000000001421, 4.999999999999962697 ) ) ;
#10057=CARTESIAN_POINT ( 'NONE',  ( 208.1451861577817795, 32.16953125108393152, 5.444914386472293977 ) ) ;
#10058=CARTESIAN_POINT ( 'NONE',  ( 142.3201169669889339, 36.00000000000002132, -5.704949255836478272 ) ) ;
#10061=FACE_OUTER_BOUND ( 'NONE', #2055, .T. ) ;
#10062=CARTESIAN_POINT ( 'NONE',  ( 214.9999999999999716, 75.00000000000000000, 14.99999999999994493 ) ) ;
#10066=FACE_OUTER_BOUND ( 'NONE', #23838, .T. ) ;
#10068=CARTESIAN_POINT ( 'NONE',  ( -13.57481594606304576, 40.99999999999999289, 0.000000000000000000 ) ) ;
#10070=CARTESIAN_POINT ( 'NONE',  ( 96.46446609406721961, 80.12500000000000000, 3.535533905932727539 ) ) ;
#10071=CARTESIAN_POINT ( 'NONE',  ( 103.1528011352953342, 81.06250000136559208, -3.152801135295383084 ) ) ;
#10072=CARTESIAN_POINT ( 'NONE',  ( 59.55508561352770158, 37.72578125108395142, 13.14518615778179722 ) ) ;
#10078=CARTESIAN_POINT ( 'NONE',  ( 120.7049497278729575, 33.50898437608393010, -9.295050272127046043 ) ) ;
#10083=CARTESIAN_POINT ( 'NONE',  ( 143.1451861577818079, 38.56914062608393579, -1.609821015232357215E-15 ) ) ;
#10084=CARTESIAN_POINT ( 'NONE',  ( 59.37712712842213136, 37.27929687716787299, 13.57481594606304753 ) ) ;
#10085=CARTESIAN_POINT ( 'NONE',  ( -20.00000000000000000, 55.00000000000000000, 10.00000000000000000 ) ) ;
#10086=CARTESIAN_POINT ( 'NONE',  ( -9.598844408820458085, 40.20625000216787726, -9.598844408820458085 ) ) ;
#10089=VERTEX_POINT ( 'NONE', #18656 ) ;
#10091=CARTESIAN_POINT ( 'NONE',  ( 185.4011555911795597, 32.46718750216787441, 9.598844408820459861 ) ) ;
#10094=CARTESIAN_POINT ( 'NONE',  ( 116.8548138422182205, 37.32890625108393579, -5.444914386472297529 ) ) ;
#10095=CARTESIAN_POINT ( 'NONE',  ( 6.944426393311538881, 31.75150625057403175, -11.16113171639042356 ) ) ;
#10096=EDGE_CURVE ( 'NONE', #23999, #20385, #17050, .T. ) ;
#10100=CARTESIAN_POINT ( 'NONE',  ( 208.5748159460630120, 38.27148437500000711, -5.622872871577873077 ) ) ;
#10108=CARTESIAN_POINT ( 'NONE',  ( 13.57481594606304576, 39.80937499999999574, -1.662435489736055892E-15 ) ) ;
#10109=ORIENTED_EDGE ( 'NONE', *, *, #6660, .T. ) ;
#10110=CARTESIAN_POINT ( 'NONE',  ( 99.99999999999995737, 81.43750000136559208, -4.458734125000016313 ) ) ;
#10113=VECTOR ( 'NONE', #9655, 1000.000000000000000 ) ;
#10115=ORIENTED_EDGE ( 'NONE', *, *, #1016, .F. ) ;
#10116=CARTESIAN_POINT ( 'NONE',  ( 189.6762090360452646, 54.47170356488337006, -15.00000000000000000 ) ) ;
#10121=CARTESIAN_POINT ( 'NONE',  ( 208.5748159460630120, 39.85898437716787157, 5.622872871577869525 ) ) ;
#10124=CARTESIAN_POINT ( 'NONE',  ( 116.8548138422182205, 39.21406250108392300, 5.444914386472304635 ) ) ;
#10125=CARTESIAN_POINT ( 'NONE',  ( 5.444914386472302859, 40.20625000108394431, 13.14518615778179189 ) ) ;
#10126=EDGE_CURVE ( 'NONE', #20676, #4003, #27515, .T. ) ;
#10128=CARTESIAN_POINT ( 'NONE',  ( 78.57481594606305464, 39.01562500000000000, -1.662435489736055892E-15 ) ) ;
#10129=CARTESIAN_POINT ( 'NONE',  ( 55.40115559117954547, 39.61093750216787868, 9.598844408820459861 ) ) ;
#10133=CARTESIAN_POINT ( 'NONE',  ( 95.54126587499996504, 82.68750000136560629, -1.387778780781445676E-14 ) ) ;
#10135=CARTESIAN_POINT ( 'NONE',  ( 13.14518615778179900, 40.40468750108393436, -5.444914386472297529 ) ) ;
#10142=DIRECTION ( 'NONE',  ( -1.000000000000000000, -0.000000000000000000, 2.385244779468110248E-16 ) ) ;
#10145=CARTESIAN_POINT ( 'NONE',  ( 74.29505027212704249, 37.27929687608394005, -9.295050272127046043 ) ) ;
#10147=CARTESIAN_POINT ( 'NONE',  ( 181.8548138422181921, 32.07031250108393294, 5.444914386472304635 ) ) ;
#10149=ADVANCED_FACE ( 'NONE', ( #6098 ), #8365, .T. ) ;
#10150=EDGE_LOOP ( 'NONE', ( #21701, #18151, #27372, #16438 ) ) ;
#10152=CARTESIAN_POINT ( 'NONE',  ( -8.259611528891891652, 50.00000000056336802, -10.79618466885709083 ) ) ;
#10153=CARTESIAN_POINT ( 'NONE',  ( 204.1801758136480203, 55.00000000000000000, 14.99999999999994671 ) ) ;
#10154=CARTESIAN_POINT ( 'NONE',  ( 120.4011555911795455, 33.26093750216787726, 9.598844408820459861 ) ) ;
#10158=CARTESIAN_POINT ( 'NONE',  ( 208.1451861577817795, 36.43593750108392726, -5.444914386472297529 ) ) ;
#10161=( BOUNDED_CURVE ( )  B_SPLINE_CURVE ( 2, ( #10795, #19935, #8815, #4692, #13061, #11077, #19509, #8534, #15209 ),
 .UNSPECIFIED., .F., .F. ) 
 B_SPLINE_CURVE_WITH_KNOTS ( ( 3, 2, 2, 2, 3 ),
 ( 0.06250000000000004163, 0.07291666666666665741, 0.08333333333333325932, 0.09374999999999987510, 0.1041666666666664909 ),
 .UNSPECIFIED. ) 
 CURVE ( )  GEOMETRIC_REPRESENTATION_ITEM ( )  RATIONAL_B_SPLINE_CURVE ( ( 0.9999999999999996669, 0.9238795325112870716, 1.000000000000000000, 0.9238795325112867385, 1.000000000000000000, 0.9238795325112867385, 1.000000000000000000, 0.9238795325112880708, 0.9999999999999986677 ) ) 
 REPRESENTATION_ITEM ( '' )  );
#10163=PLANE ( 'NONE',  #4817 ) ;
#10166=CARTESIAN_POINT ( 'NONE',  ( 181.8548138422182205, 40.55351562608393579, 0.000000000000000000 ) ) ;
#10170=DIRECTION ( 'NONE',  ( 0.000000000000000000, 0.000000000000000000, 1.000000000000000000 ) ) ;
#10173=VERTEX_POINT ( 'NONE', #28179 ) ;
#10176=ORIENTED_EDGE ( 'NONE', *, *, #12095, .T. ) ;
#10178=CARTESIAN_POINT ( 'NONE',  ( 124.5550856135277087, 38.51953125108393294, 13.14518615778179722 ) ) ;
#10179=CARTESIAN_POINT ( 'NONE',  ( 51.85481384221819923, 37.32890625108393579, -5.444914386472297529 ) ) ;
#10180=LINE ( 'NONE', #23459, #12491 ) ;
#10181=CARTESIAN_POINT ( 'NONE',  ( -13.14518615778179544, 34.99726562608393721, 0.000000000000000000 ) ) ;
#10182=CARTESIAN_POINT ( 'NONE',  ( 194.0044387749465784, 36.00000000000000000, -13.45766439703020367 ) ) ;
#10183=LINE ( 'NONE', #1392, #6171 ) ;
#10184=CARTESIAN_POINT ( 'NONE',  ( 217.9999999999999716, 52.00000000000000711, 12.99999999999994316 ) ) ;
#10185=EDGE_CURVE ( 'NONE', #23121, #2928, #2524, .T. ) ;
#10186=DIRECTION ( 'NONE',  ( -1.000000000000000000, -0.000000000000000000, 2.385244779468110248E-16 ) ) ;
#10187=CYLINDRICAL_SURFACE ( 'NONE', #16636, 5.000000000000004441 ) ;
#10188=CARTESIAN_POINT ( 'NONE',  ( 13.14518615778179900, 39.31328125108392868, 5.444914386472293977 ) ) ;
#10189=CARTESIAN_POINT ( 'NONE',  ( 99.99999999999995737, 85.00000000000000000, -5.000000000000018652 ) ) ;
#10195=CARTESIAN_POINT ( 'NONE',  ( 195.0000000000000000, -7.395377635281828788, -13.57481594606306707 ) ) ;
#10199=DIRECTION ( 'NONE',  ( -1.000000000000000000, 0.000000000000000000, 0.000000000000000000 ) ) ;
#10206=CARTESIAN_POINT ( 'NONE',  ( 103.1528011352953342, 83.31250000136560629, -3.152801135295383084 ) ) ;
#10207=CARTESIAN_POINT ( 'NONE',  ( 70.44491438647230552, 37.32890625108393579, -13.14518615778179900 ) ) ;
#10211=CARTESIAN_POINT ( 'NONE',  ( 130.0000000000000000, 36.83281249999999574, -13.57481594606304576 ) ) ;
#10213=CARTESIAN_POINT ( 'NONE',  ( 120.7049497278729575, 32.71523437608393436, -9.295050272127046043 ) ) ;
#10215=CARTESIAN_POINT ( 'NONE',  ( 130.0000000000000000, 37.72578125216787726, -13.57481594606304576 ) ) ;
#10216=DIRECTION ( 'NONE',  ( 0.000000000000000000, 1.000000000000000000, 0.000000000000000000 ) ) ;
#10217=CARTESIAN_POINT ( 'NONE',  ( 95.54126587499996504, 79.43750000136559208, -1.387778780781445676E-14 ) ) ;
#10219=CARTESIAN_POINT ( 'NONE',  ( 65.00000000000000000, 38.12265625216787157, 13.57481594606304576 ) ) ;
#10220=AXIS2_PLACEMENT_3D ( 'NONE', #24759, #5239, #27051 ) ;
#10222=CARTESIAN_POINT ( 'NONE',  ( -13.57481594606304576, 36.38632812716788578, 5.622872871577880183 ) ) ;
#10227=CARTESIAN_POINT ( 'NONE',  ( 208.1451861577818079, 36.98164062608393010, -1.609821015232357215E-15 ) ) ;
#10228=CARTESIAN_POINT ( 'NONE',  ( 13.57481594606304931, 36.68398437716787441, 5.622872871577868636 ) ) ;
#10229=EDGE_CURVE ( 'NONE', #6540, #18933, #23760, .T. ) ;
#10230=CARTESIAN_POINT ( 'NONE',  ( 139.2950502721270425, 36.88242187608393152, 9.295050272127046043 ) ) ;
#10231=CARTESIAN_POINT ( 'NONE',  ( 96.46446609406721961, 80.25000000273119838, 3.535533905932727539 ) ) ;
#10233=CARTESIAN_POINT ( 'NONE',  ( 130.0000000000000000, -7.395377635281828788, 11.57481594606302799 ) ) ;
#10234=CARTESIAN_POINT ( 'NONE',  ( 130.0000000000000000, -7.395377635281828788, 13.57481594606302799 ) ) ;
#10236=CARTESIAN_POINT ( 'NONE',  ( 189.3771271284221314, 38.76757812500000000, 13.57481594606304753 ) ) ;
#10240=CARTESIAN_POINT ( 'NONE',  ( 59.55508561352770158, 37.22968750108393721, -13.14518615778179900 ) ) ;
#10245=FACE_OUTER_BOUND ( 'NONE', #14370, .T. ) ;
#10246=CARTESIAN_POINT ( 'NONE',  ( 9.598844408820459861, 38.91640624999999432, 9.598844408820456309 ) ) ;
#10247=FACE_OUTER_BOUND ( 'NONE', #726, .T. ) ;
#10249=DIRECTION ( 'NONE',  ( 0.000000000000000000, 1.000000000000000000, 0.000000000000000000 ) ) ;
#10252=DIRECTION ( 'NONE',  ( 0.000000000000000000, 0.000000000000000000, -1.000000000000000000 ) ) ;
#10253=VERTEX_POINT ( 'NONE', #25900 ) ;
#10257=ORIENTED_EDGE ( 'NONE', *, *, #10, .F. ) ;
#10260=DIRECTION ( 'NONE',  ( 0.000000000000000000, 0.000000000000000000, 1.000000000000000000 ) ) ;
#10264=CARTESIAN_POINT ( 'NONE',  ( -5.444914386472299306, 36.13828125108393152, 13.14518615778179722 ) ) ;
#10265=CARTESIAN_POINT ( 'NONE',  ( -13.14518615778179544, 31.82226562608393650, 0.000000000000000000 ) ) ;
#10267=CARTESIAN_POINT ( 'NONE',  ( 59.37712712842213136, 38.76757812500000000, 13.57481594606304753 ) ) ;
#10270=CARTESIAN_POINT ( 'NONE',  ( 203.1931556449107177, 36.00000000000000000, 10.45682415286345446 ) ) ;
#10274=CARTESIAN_POINT ( 'NONE',  ( 101.8468681455907046, 83.00000000136562051, 4.458734124999987891 ) ) ;
#10276=CARTESIAN_POINT ( 'NONE',  ( 13.14518615778179544, 38.76757812608393294, -1.609821015232357215E-15 ) ) ;
#10279=( BOUNDED_SURFACE ( )  B_SPLINE_SURFACE ( 1, 2, ( 
 ( #11826, #20549, #14248, #16254, #1031, #9702, #8120, #12509, #21381, #6260, #21098, #25511, #3718, #1993, #21513, #25642, #6125, #23376, #19511, #18949, #27658, #10382, #19367, #23789, #8254, #23514, #10797, #7978, #14791, #21238, #19231, #16814, #12656, #27932, #5991, #17077, #16677, #8391, #1720, #3993, #5856, #25376, #14656, #28070, #25782, #8536, #3849, #14526, #23241, #1860, #10524, #19089, #27797, #17222, #15070, #16941, #25927, #14933, #23654, #1586, #12379, #4129, #12795, #10660, #6401, #4265, #12925, #10240, #21657, #2133, #10937, #11361, #6814, #24214, #22222, #417, #20085, #8677, #6956, #4841, #23930, #26647, #13502, #6533, #19937, #2701, #11220, #11504, #17797, #11079, #13063, #15210, #4409, #8959, #562, #19791, #9102, #19649, #14017, #21943, #21800, #2279, #273, #4693, #7094, #17648, #17506, #26356, #2559, #131, #9243, #2836, #15503, #13354, #15651, #22082, #26499, #24350, #8817, #17936, #15793, #24496, #4981, #13647, #22362, #17368, #26064, #26207, #6670, #15356, #24071, #4547, #13209, #2421, #9664, #18367, #7378, #3545, #2970, #11645, #22653, #3395, #7814, #20514, #7525, #23067, #20221, #27073, #24780, #3264, #854, #24921, #11931, #20369, #1137, #705, #20653, #5261, #16220, #18076, #9379, #26935, #12066, #9805, #20791, #16072, #26790, #7235, #5405, #14075, #18226, #9526, #1272, #27356, #3123, #9936, #22795, #18510, #13783, #15926, #27217, #996, #25065 ),
 ( #13925, #18651, #7671, #16364, #14216, #5551, #16506, #24644, #22934, #25200, #5117, #5686, #14352, #22505, #11790, #17046, #23480, #23755, #1824, #23343, #25336, #18784, #27491, #21204, #4097, #3817, #12620, #23209, #12202, #5957, #5822, #7947, #12477, #8221, #10629, #1687, #1554, #10346, #14760, #12348, #25750, #15038, #19053, #27762, #27900, #16911, #21345, #25609, #14492, #1960, #6093, #14899, #3960, #10489, #19197, #8360, #8504, #12760, #23620, #6232, #20929, #10072, #19334, #21480, #21066, #16779, #28037, #17189, #3684, #10207, #16644, #25896, #6366, #1413, #18917, #27626, #8084, #25479, #14625, #13172, #17762, #26029, #21911, #19753, #8646, #6919, #13458, #6500, #19899, #26465, #15176, #24314, #383, #4515, #15612, #4800, #22184, #2664, #8781, #26609, #4657, #11324, #9067, #8923, #24036, #2097, #20046, #19476, #236, #525, #9206, #2519, #17900, #7055, #15322, #15754, #26319, #2244, #17335, #2386, #23895, #11044, #10765, #17611, #4233, #28175, #13030, #12891, #21621, #4374, #21767, #10906, #6780, #19615, #15465, #100, #17469, #26171, #6638, #24179, #13318, #22044, #11181, #22614, #3222, #954, #16030, #5083, #24742, #25025, #18473, #22469, #669, #7341, #18330, #3084, #1097, #5223, #9764, #13888, #2934, #5365, #11751, #1236, #20477, #815, #12029, #13745, #16326, #27317, #26750, #14175, #27181, #5507, #7773, #11604, #7483, #22892, #4942, #7632, #3357, #20327, #9625 ) ),
 .UNSPECIFIED., .F., .F., .F. ) 
 B_SPLINE_SURFACE_WITH_KNOTS ( ( 2, 2 ),
 ( 3, 2, 2, 2, 2, 2, 2, 2, 2, 2, 2, 2, 2, 2, 2, 2, 2, 2, 2, 2, 2, 2, 2, 2, 2, 2, 2, 2, 2, 2, 2, 2, 2, 2, 2, 2, 2, 2, 2, 2, 2, 2, 2, 2, 2, 2, 2, 2, 2, 2, 2, 2, 2, 2, 2, 2, 2, 2, 2, 2, 2, 2, 2, 2, 2, 2, 2, 2, 2, 2, 2, 2, 2, 2, 2, 2, 2, 2, 2, 2, 2, 2, 2, 2, 2, 2, 2, 2, 2, 2, 2, 3 ),
 ( 0.000000000000000000, 1.000000000000000000 ),
 ( 0.000000000000000000, 0.01041666666666666609, 0.02083333333333333218, 0.03125000000000000000, 0.04166666666666666435, 0.05208333333333333565, 0.06250000000000000000, 0.07291666666666667129, 0.08333333333333332871, 0.09375000000000000000, 0.1041666666666666713, 0.1145833333333333287, 0.1250000000000000000, 0.1354166666666666574, 0.1458333333333333426, 0.1562500000000000000, 0.1666666666666666574, 0.1770833333333333426, 0.1875000000000000000, 0.1979166666666666574, 0.2083333333333333426, 0.2187500000000000000, 0.2291666666666666574, 0.2395833333333333426, 0.2500000000000000000, 0.2604166666666666852, 0.2708333333333333148, 0.2812500000000000000, 0.2916666666666666852, 0.3020833333333333148, 0.3125000000000000000, 0.3229166666666666852, 0.3333333333333333148, 0.3437500000000000000, 0.3541666666666666852, 0.3645833333333333148, 0.3750000000000000000, 0.3854166666666666852, 0.3958333333333333148, 0.4062500000000000000, 0.4166666666666666852, 0.4270833333333333148, 0.4375000000000000000, 0.4479166666666666852, 0.4583333333333333148, 0.4687500000000000000, 0.4791666666666666852, 0.4895833333333333148, 0.5000000000000000000, 0.5104166666666666297, 0.5208333333333333703, 0.5312500000000000000, 0.5416666666666666297, 0.5520833333333333703, 0.5625000000000000000, 0.5729166666666666297, 0.5833333333333333703, 0.5937500000000000000, 0.6041666666666666297, 0.6145833333333333703, 0.6250000000000000000, 0.6354166666666666297, 0.6458333333333333703, 0.6562500000000000000, 0.6666666666666666297, 0.6770833333333333703, 0.6875000000000000000, 0.6979166666666666297, 0.7083333333333333703, 0.7187500000000000000, 0.7291666666666666297, 0.7395833333333333703, 0.7500000000000000000, 0.7604166666666666297, 0.7708333333333333703, 0.7812500000000000000, 0.7916666666666666297, 0.8020833333333333703, 0.8125000000000000000, 0.8229166666666666297, 0.8333333333333333703, 0.8437500000000000000, 0.8541666666666666297, 0.8645833333333333703, 0.8750000000000000000, 0.8854166666666666297, 0.8958333333333333703, 0.9062500000000000000, 0.9166666666666666297, 0.9270833333333333703, 0.9375000000000000000, 0.9448587001587775980 ),
 .UNSPECIFIED. ) 
 GEOMETRIC_REPRESENTATION_ITEM ( )  RATIONAL_B_SPLINE_SURFACE ( (
 ( 1.000000000000000000, 0.9238795325112867385, 1.000000000000000000, 0.9238795325112867385, 1.000000000000000000, 0.9238795325112867385, 1.000000000000000000, 0.9238795325112867385, 1.000000000000000000, 0.9238795325112867385, 1.000000000000000000, 0.9238795325112867385, 1.000000000000000000, 0.9238795325112867385, 1.000000000000000000, 0.9238795325112867385, 1.000000000000000000, 0.9238795325112867385, 1.000000000000000000, 0.9238795325112867385, 1.000000000000000000, 0.9238795325112867385, 1.000000000000000000, 0.9238795325112867385, 1.000000000000000000, 0.9238795325112867385, 1.000000000000000000, 0.9238795325112867385, 1.000000000000000000, 0.9238795325112867385, 1.000000000000000000, 0.9238795325112867385, 1.000000000000000000, 0.9238795325112867385, 1.000000000000000000, 0.9238795325112867385, 1.000000000000000000, 0.9238795325112867385, 1.000000000000000000, 0.9238795325112867385, 1.000000000000000000, 0.9238795325112867385, 1.000000000000000000, 0.9238795325112867385, 1.000000000000000000, 0.9238795325112867385, 1.000000000000000000, 0.9238795325112867385, 1.000000000000000000, 0.9238795325112867385, 1.000000000000000000, 0.9238795325112867385, 1.000000000000000000, 0.9238795325112867385, 1.000000000000000000, 0.9238795325112867385, 1.000000000000000000, 0.9238795325112867385, 1.000000000000000000, 0.9238795325112867385, 1.000000000000000000, 0.9238795325112867385, 1.000000000000000000, 0.9238795325112867385, 1.000000000000000000, 0.9238795325112867385, 1.000000000000000000, 0.9238795325112867385, 1.000000000000000000, 0.9238795325112867385, 1.000000000000000000, 0.9238795325112867385, 1.000000000000000000, 0.9238795325112867385, 1.000000000000000000, 0.9238795325112867385, 1.000000000000000000, 0.9238795325112867385, 1.000000000000000000, 0.9238795325112867385, 1.000000000000000000, 0.9238795325112867385, 1.000000000000000000, 0.9238795325112867385, 1.000000000000000000, 0.9238795325112867385, 1.000000000000000000, 0.9238795325112867385, 1.000000000000000000, 0.9238795325112867385, 1.000000000000000000, 0.9238795325112867385, 1.000000000000000000, 0.9238795325112867385, 1.000000000000000000, 0.9238795325112867385, 1.000000000000000000, 0.9238795325112867385, 1.000000000000000000, 0.9238795325112867385, 1.000000000000000000, 0.9238795325112867385, 1.000000000000000000, 0.9238795325112867385, 1.000000000000000000, 0.9238795325112867385, 1.000000000000000000, 0.9238795325112867385, 1.000000000000000000, 0.9238795325112867385, 1.000000000000000000, 0.9238795325112867385, 1.000000000000000000, 0.9238795325112867385, 1.000000000000000000, 0.9238795325112867385, 1.000000000000000000, 0.9238795325112867385, 1.000000000000000000, 0.9238795325112867385, 1.000000000000000000, 0.9238795325112867385, 1.000000000000000000, 0.9238795325112867385, 1.000000000000000000, 0.9238795325112867385, 1.000000000000000000, 0.9238795325112867385, 1.000000000000000000, 0.9238795325112867385, 1.000000000000000000, 0.9238795325112867385, 1.000000000000000000, 0.9238795325112867385, 1.000000000000000000, 0.9238795325112867385, 1.000000000000000000, 0.9238795325112867385, 1.000000000000000000, 0.9238795325112867385, 1.000000000000000000, 0.9238795325112867385, 1.000000000000000000, 0.9238795325112867385, 1.000000000000000000, 0.9238795325112867385, 1.000000000000000000, 0.9238795325112867385, 1.000000000000000000, 0.9238795325112867385, 1.000000000000000000, 0.9238795325112867385, 1.000000000000000000, 0.9238795325112867385, 1.000000000000000000, 0.9238795325112867385, 1.000000000000000000, 0.9238795325112867385, 1.000000000000000000, 0.9238795325112867385, 1.000000000000000000, 0.9238795325112867385, 1.000000000000000000, 0.9238795325112867385, 1.000000000000000000, 0.9238795325112867385, 1.000000000000000000, 0.9238795325112867385, 1.000000000000000000, 0.9238795325112867385, 1.000000000000000000, 0.9238795325112867385, 1.000000000000000000, 0.9238795325112867385, 1.000000000000000000, 0.9238795325112867385, 1.000000000000000000, 0.9238795325112867385, 1.000000000000000000, 0.9238795325112867385, 1.000000000000000000, 0.9462258211652395667, 0.9684275895297407288),
 ( 1.000000000000000000, 0.9238795325112867385, 1.000000000000000000, 0.9238795325112867385, 1.000000000000000000, 0.9238795325112867385, 1.000000000000000000, 0.9238795325112867385, 1.000000000000000000, 0.9238795325112867385, 1.000000000000000000, 0.9238795325112867385, 1.000000000000000000, 0.9238795325112867385, 1.000000000000000000, 0.9238795325112867385, 1.000000000000000000, 0.9238795325112867385, 1.000000000000000000, 0.9238795325112867385, 1.000000000000000000, 0.9238795325112867385, 1.000000000000000000, 0.9238795325112867385, 1.000000000000000000, 0.9238795325112867385, 1.000000000000000000, 0.9238795325112867385, 1.000000000000000000, 0.9238795325112867385, 1.000000000000000000, 0.9238795325112867385, 1.000000000000000000, 0.9238795325112867385, 1.000000000000000000, 0.9238795325112867385, 1.000000000000000000, 0.9238795325112867385, 1.000000000000000000, 0.9238795325112867385, 1.000000000000000000, 0.9238795325112867385, 1.000000000000000000, 0.9238795325112867385, 1.000000000000000000, 0.9238795325112867385, 1.000000000000000000, 0.9238795325112867385, 1.000000000000000000, 0.9238795325112867385, 1.000000000000000000, 0.9238795325112867385, 1.000000000000000000, 0.9238795325112867385, 1.000000000000000000, 0.9238795325112867385, 1.000000000000000000, 0.9238795325112867385, 1.000000000000000000, 0.9238795325112867385, 1.000000000000000000, 0.9238795325112867385, 1.000000000000000000, 0.9238795325112867385, 1.000000000000000000, 0.9238795325112867385, 1.000000000000000000, 0.9238795325112867385, 1.000000000000000000, 0.9238795325112867385, 1.000000000000000000, 0.9238795325112867385, 1.000000000000000000, 0.9238795325112867385, 1.000000000000000000, 0.9238795325112867385, 1.000000000000000000, 0.9238795325112867385, 1.000000000000000000, 0.9238795325112867385, 1.000000000000000000, 0.9238795325112867385, 1.000000000000000000, 0.9238795325112867385, 1.000000000000000000, 0.9238795325112867385, 1.000000000000000000, 0.9238795325112867385, 1.000000000000000000, 0.9238795325112867385, 1.000000000000000000, 0.9238795325112867385, 1.000000000000000000, 0.9238795325112867385, 1.000000000000000000, 0.9238795325112867385, 1.000000000000000000, 0.9238795325112867385, 1.000000000000000000, 0.9238795325112867385, 1.000000000000000000, 0.9238795325112867385, 1.000000000000000000, 0.9238795325112867385, 1.000000000000000000, 0.9238795325112867385, 1.000000000000000000, 0.9238795325112867385, 1.000000000000000000, 0.9238795325112867385, 1.000000000000000000, 0.9238795325112867385, 1.000000000000000000, 0.9238795325112867385, 1.000000000000000000, 0.9238795325112867385, 1.000000000000000000, 0.9238795325112867385, 1.000000000000000000, 0.9238795325112867385, 1.000000000000000000, 0.9238795325112867385, 1.000000000000000000, 0.9238795325112867385, 1.000000000000000000, 0.9238795325112867385, 1.000000000000000000, 0.9238795325112867385, 1.000000000000000000, 0.9238795325112867385, 1.000000000000000000, 0.9238795325112867385, 1.000000000000000000, 0.9238795325112867385, 1.000000000000000000, 0.9238795325112867385, 1.000000000000000000, 0.9238795325112867385, 1.000000000000000000, 0.9238795325112867385, 1.000000000000000000, 0.9238795325112867385, 1.000000000000000000, 0.9238795325112867385, 1.000000000000000000, 0.9238795325112867385, 1.000000000000000000, 0.9238795325112867385, 1.000000000000000000, 0.9238795325112867385, 1.000000000000000000, 0.9238795325112867385, 1.000000000000000000, 0.9238795325112867385, 1.000000000000000000, 0.9238795325112867385, 1.000000000000000000, 0.9238795325112867385, 1.000000000000000000, 0.9238795325112867385, 1.000000000000000000, 0.9238795325112867385, 1.000000000000000000, 0.9238795325112867385, 1.000000000000000000, 0.9238795325112867385, 1.000000000000000000, 0.9238795325112867385, 1.000000000000000000, 0.9238795325112867385, 1.000000000000000000, 0.9238795325112867385, 1.000000000000000000, 0.9238795325112867385, 1.000000000000000000, 0.9238795325112867385, 1.000000000000000000, 0.9238795325112867385, 1.000000000000000000, 0.9238795325112867385, 1.000000000000000000, 0.9462258211652395667, 0.9684275895297407288) ) ) 
 REPRESENTATION_ITEM ( '' )  SURFACE ( )  );
#10280=AXIS2_PLACEMENT_3D ( 'NONE', #15567, #4756, #13416 ) ;
#10286=CARTESIAN_POINT ( 'NONE',  ( 116.4251840539369596, 39.51171875216787299, 0.000000000000000000 ) ) ;
#10287=VECTOR ( 'NONE', #3176, 1000.000000000000000 ) ;
#10289=CARTESIAN_POINT ( 'NONE',  ( 78.14518615778180788, 38.02343750108395426, -5.444914386472297529 ) ) ;
#10290=CARTESIAN_POINT ( 'NONE',  ( 94.99999999999995737, 83.12500000273119838, -1.387778780781445676E-14 ) ) ;
#10291=CARTESIAN_POINT ( 'NONE',  ( 204.2950502721270425, 32.51679687608393721, -9.295050272127046043 ) ) ;
#10292=ORIENTED_EDGE ( 'NONE', *, *, #24047, .T. ) ;
#10295=CARTESIAN_POINT ( 'NONE',  ( 139.5988444088204403, 36.83281250216787583, -9.598844408820458085 ) ) ;
#10296=CARTESIAN_POINT ( 'NONE',  ( 116.4251840539369596, 33.95546875216787441, 0.000000000000000000 ) ) ;
#10298=CARTESIAN_POINT ( 'NONE',  ( 78.14518615778179367, 40.40468750108393436, -5.444914386472297529 ) ) ;
#10299=CARTESIAN_POINT ( 'NONE',  ( 185.7049497278729575, 38.46992187608393721, 9.295050272127047819 ) ) ;
#10300=ORIENTED_EDGE ( 'NONE', *, *, #15897, .F. ) ;
#10301=VERTEX_POINT ( 'NONE', #15043 ) ;
#10309=CARTESIAN_POINT ( 'NONE',  ( 12.32011696698886816, 36.00000000000001421, -5.704949255836485378 ) ) ;
#10311=CARTESIAN_POINT ( 'NONE',  ( 120.4011555911795455, 32.36796874999999574, 9.598844408820459861 ) ) ;
#10315=CIRCLE ( 'NONE', #17614, 13.57481594606304398 ) ;
#10317=CARTESIAN_POINT ( 'NONE',  ( 116.8548138422182205, 39.16445312608393436, 0.000000000000000000 ) ) ;
#10319=CARTESIAN_POINT ( 'NONE',  ( 65.00000000000000000, 37.57695312608392868, 13.14518615778179544 ) ) ;
#10320=CARTESIAN_POINT ( 'NONE',  ( 189.5550856135277229, 39.31328125108394289, 13.14518615778179722 ) ) ;
#10321=EDGE_CURVE ( 'NONE', #25975, #8262, #2680, .T. ) ;
#10323=CARTESIAN_POINT ( 'NONE',  ( -9.295050272127046043, 35.69179687608393436, -9.295050272127046043 ) ) ;
#10325=CARTESIAN_POINT ( 'NONE',  ( 195.7050241099688606, 35.99999999999999289, 13.13343125082109175 ) ) ;
#10327=CARTESIAN_POINT ( 'NONE',  ( 95.27063293749995410, 84.84375000068281736, -1.387778780781445676E-14 ) ) ;
#10328=CARTESIAN_POINT ( 'NONE',  ( 13.14518615778179900, 37.03125000108393294, -5.444914386472297529 ) ) ;
#10329=CARTESIAN_POINT ( 'NONE',  ( 143.3933367278051207, 36.00000000000001421, -2.034633736484514621 ) ) ;
#10334=CARTESIAN_POINT ( 'NONE',  ( 116.4251840539369596, 40.25585937716787299, -5.622872871577872189 ) ) ;
#10344=CARTESIAN_POINT ( 'NONE',  ( 185.4011555911795313, 36.23750000216787726, -9.598844408820458085 ) ) ;
#10345=CARTESIAN_POINT ( 'NONE',  ( 104.4587341249999781, 84.12500000136560629, 1.846868145590721655 ) ) ;
#10346=CARTESIAN_POINT ( 'NONE',  ( 70.44491438647230552, 38.91640625108393436, -13.14518615778179900 ) ) ;
#10348=CARTESIAN_POINT ( 'NONE',  ( -9.295050272127046043, 40.45429687608393721, -9.295050272127046043 ) ) ;
#10350=CARTESIAN_POINT ( 'NONE',  ( 65.00000000000000000, 38.51953125216787299, -13.57481594606304576 ) ) ;
#10352=CARTESIAN_POINT ( 'NONE',  ( 133.7556381558600265, 31.78804748261757140, -13.14518615778179367 ) ) ;
#10353=EDGE_LOOP ( 'NONE', ( #24402, #16652, #16829, #15544 ) ) ;
#10354=CARTESIAN_POINT ( 'NONE',  ( -20.00000000000000000, 55.00000000000000000, 10.00000000000000178 ) ) ;
#10356=CARTESIAN_POINT ( 'NONE',  ( 104.4587341249999639, 79.93750000136559208, -1.442382525525748735E-14 ) ) ;
#10357=CARTESIAN_POINT ( 'NONE',  ( 124.5550856135277087, 40.40468750108393436, -13.14518615778179900 ) ) ;
#10358=EDGE_CURVE ( 'NONE', #24596, #21433, #17670, .T. ) ;
#10359=CARTESIAN_POINT ( 'NONE',  ( 59.37712712842213136, 36.48554687716787015, 13.57481594606304753 ) ) ;
#10361=CARTESIAN_POINT ( 'NONE',  ( -13.57481594606304576, 34.74921875216787726, 0.000000000000000000 ) ) ;
#10363=ADVANCED_FACE ( 'NONE', ( #8927 ), #17616, .T. ) ;
#10364=AXIS2_PLACEMENT_3D ( 'NONE', #17044, #14897, #15463 ) ;
#10368=CARTESIAN_POINT ( 'NONE',  ( 181.8548138422181921, 37.32890625108393579, -5.444914386472297529 ) ) ;
#10372=CARTESIAN_POINT ( 'NONE',  ( 116.8548138422182205, 36.58476562608393579, 0.000000000000000000 ) ) ;
#10374=CARTESIAN_POINT ( 'NONE',  ( 135.6228728715778686, 37.57695312499999574, -13.57481594606304753 ) ) ;
#10376=CARTESIAN_POINT ( 'NONE',  ( 65.00000000000000000, 38.51953125216787299, -13.57481594606304576 ) ) ;
#10378=CARTESIAN_POINT ( 'NONE',  ( 181.4251840539369596, 38.66835937499999432, 5.622872871577880183 ) ) ;
#10382=CARTESIAN_POINT ( 'NONE',  ( 70.44491438647230552, 39.51171875108392584, -13.14518615778179900 ) ) ;
#10384=CARTESIAN_POINT ( 'NONE',  ( 139.1801758136479918, 55.00000000000000000, 9.999999999999964473 ) ) ;
#10386=DIRECTION ( 'NONE',  ( 0.000000000000000000, 0.000000000000000000, -1.000000000000000000 ) ) ;
#10387=CARTESIAN_POINT ( 'NONE',  ( -13.57481594606304576, 38.61874999999999147, 0.000000000000000000 ) ) ;
#10388=CARTESIAN_POINT ( 'NONE',  ( 116.8548138422182205, 39.95820312608393010, 0.000000000000000000 ) ) ;
#10389=AXIS2_PLACEMENT_3D ( 'NONE', #9872, #22721, #11858 ) ;
#10392=CARTESIAN_POINT ( 'NONE',  ( 103.1528011352953342, 81.06250000136559208, 3.152801135295355106 ) ) ;
#10393=VECTOR ( 'NONE', #24442, 1000.000000000000000 ) ;
#10395=VERTEX_POINT ( 'NONE', #20190 ) ;
#10397=CARTESIAN_POINT ( 'NONE',  ( 78.14518615778179367, 35.64218750108393152, -5.444914386472297529 ) ) ;
#10400=CARTESIAN_POINT ( 'NONE',  ( 124.6826484225240961, 54.47013368152369850, -15.00000000000000000 ) ) ;
#10401=ADVANCED_FACE ( 'NONE', ( #18189 ), #18762, .T. ) ;
#10403=VERTEX_POINT ( 'NONE', #25160 ) ;
#10404=DIRECTION ( 'NONE',  ( 1.000000000000000000, 0.000000000000000000, -2.385244779468110248E-16 ) ) ;
#10406=CARTESIAN_POINT ( 'NONE',  ( 181.4251840539369596, 38.71796875216787726, 0.000000000000000000 ) ) ;
#10408=CARTESIAN_POINT ( 'NONE',  ( 77.07727640983618755, 35.99999999999999289, -6.197985357348142266 ) ) ;
#10409=CARTESIAN_POINT ( 'NONE',  ( 201.1198436276839629, 51.28708186915499567, 14.99999999999995204 ) ) ;
#10410=CARTESIAN_POINT ( 'NONE',  ( -13.09590655363597733, 35.99999999999999289, 1.137167824541468031 ) ) ;
#10411=CARTESIAN_POINT ( 'NONE',  ( 9.295050272127047819, 38.66835937608393436, 9.295050272127046043 ) ) ;
#10413=COLOUR_RGB ( '', 0.09019608, 0.27058824, 0.51372549) ;
#10414=CARTESIAN_POINT ( 'NONE',  ( 65.00000000000000000, 38.02343749999999289, 13.57481594606304576 ) ) ;
#10416=CARTESIAN_POINT ( 'NONE',  ( 130.0000000000000000, 40.10703125216787157, -13.57481594606304576 ) ) ;
#10417=( BOUNDED_SURFACE ( )  B_SPLINE_SURFACE ( 1, 2, ( 
 ( #12396, #3315, #18567, #1049, #7998, #18423, #18834, #5740, #23124, #10121, #3599, #27541, #9721, #12257, #21117, #7582, #1604, #11986, #20710, #27269, #7725, #23396, #19252, #23811, #17247, #6146, #23952, #13086, #27954, #19532, #4434, #3869, #10406, #27678, #21404, #12531, #21681, #17100, #8411, #8698, #21259, #21826, #4288, #4012, #27820, #12946, #2301, #25803, #25664, #10961, #19388, #8141, #2156, #17389, #16835, #6011, #10817, #12813, #2012, #6280, #23676, #25531, #14, #26088, #28093, #6554, #14675, #6422, #15234, #1740, #19112, #12678, #25947, #8273, #16964, #14811, #14957, #23536, #15091, #1882, #10545, #4153, #21536, #10681, #8556, #15379, #2441, #19672, #13375, #4569, #13669, #9124, #11243, #728, #13230, #5140, #15814, #24234, #19815, #5006, #22529, #17817, #17672, #2996, #11385, #156, #24519, #9400, #8840, #26232, #22383, #4860, #22246, #19961, #15673, #15950, #20243, #2857, #13526, #17531, #6690, #18099, #21962, #26812, #9263, #24094, #17957, #11102, #8983, #298, #11524, #7260, #26521, #6977, #6836, #26380, #15527, #4716, #22105, #24665, #13806, #438, #2583, #24372, #2724, #20107, #585, #26668, #7114, #16385, #7694, #5428, #1161, #18804, #1432, #14097, #18250, #18533, #10091, #25084, #22958, #20390, #23090, #27096, #23229, #877, #9826, #5572, #9691, #11815, #3564, #27510, #22816, #7966, #11669, #9548, #18673, #7549, #16667, #14236, #12223, #20537, #25363 ),
 ( #27238, #3284, #18390, #20811, #3420, #5843, #12088, #16245, #14512, #1020, #27374, #20951, #26958, #5284, #7401, #1291, #16094, #24942, #24802, #13948, #9960, #22675, #3148, #11955, #7833, #20678, #16527, #25219, #5709, #14375, #8663, #10784, #19497, #25631, #8107, #19354, #23364, #19216, #17210, #2117, #25915, #10511, #12782, #25498, #17065, #19077, #6387, #28057, #15058, #23775, #4252, #5978, #21368, #27920, #12911, #25769, #1848, #21643, #1709, #1574, #8380, #6248, #21498, #28195, #14779, #10368, #6520, #23641, #15197, #8523, #17354, #3706, #10227, #26050, #14920, #4116, #23500, #1979, #12367, #21086, #18937, #10648, #27646, #16801, #14645, #3836, #12497, #21224, #27782, #8240, #16930, #6113, #3979, #12642, #9228, #13340, #22069, #11065, #7219, #6655, #15341, #26342, #7079, #11488, #24199, #19635, #9365, #4968, #691, #258, #6941, #4532, #405, #19921, #17631, #2545, #2820, #13629, #6799, #2266, #11206, #22349, #9087, #15637, #4394, #15775, #19775, #23914, #13050, #17783, #117, #15485, #21787, #10926, #24057, #4678, #8801, #26486, #26774, #17492, #13194, #20204, #26190, #21929, #547, #18059, #24338, #2405, #4824, #8943, #13484, #22206, #2686, #11346, #20069, #17921, #26632, #24481, #13910, #1258, #11629, #5246, #9648, #24765, #3529, #11774, #5104, #20353, #27059, #10057, #20774, #16202, #9918, #5389, #22638, #25048, #22779, #20914, #11915, #20498, #12185, #3106, #3378 ) ),
 .UNSPECIFIED., .F., .F., .T. ) 
 B_SPLINE_SURFACE_WITH_KNOTS ( ( 2, 2 ),
 ( 3, 2, 2, 2, 2, 2, 2, 2, 2, 2, 2, 2, 2, 2, 2, 2, 2, 2, 2, 2, 2, 2, 2, 2, 2, 2, 2, 2, 2, 2, 2, 2, 2, 2, 2, 2, 2, 2, 2, 2, 2, 2, 2, 2, 2, 2, 2, 2, 2, 2, 2, 2, 2, 2, 2, 2, 2, 2, 2, 2, 2, 2, 2, 2, 2, 2, 2, 2, 2, 2, 2, 2, 2, 2, 2, 2, 2, 2, 2, 2, 2, 2, 2, 2, 2, 2, 2, 2, 2, 2, 2, 3 ),
 ( 0.000000000000000000, 1.000000000000000000 ),
 ( 0.000000000000000000, 0.01041666666666666609, 0.02083333333333333218, 0.03125000000000000000, 0.04166666666666666435, 0.05208333333333333565, 0.06250000000000000000, 0.07291666666666667129, 0.08333333333333332871, 0.09375000000000000000, 0.1041666666666666713, 0.1145833333333333287, 0.1250000000000000000, 0.1354166666666666574, 0.1458333333333333426, 0.1562500000000000000, 0.1666666666666666574, 0.1770833333333333426, 0.1875000000000000000, 0.1979166666666666574, 0.2083333333333333426, 0.2187500000000000000, 0.2291666666666666574, 0.2395833333333333426, 0.2500000000000000000, 0.2604166666666666852, 0.2708333333333333148, 0.2812500000000000000, 0.2916666666666666852, 0.3020833333333333148, 0.3125000000000000000, 0.3229166666666666852, 0.3333333333333333148, 0.3437500000000000000, 0.3541666666666666852, 0.3645833333333333148, 0.3750000000000000000, 0.3854166666666666852, 0.3958333333333333148, 0.4062500000000000000, 0.4166666666666666852, 0.4270833333333333148, 0.4375000000000000000, 0.4479166666666666852, 0.4583333333333333148, 0.4687500000000000000, 0.4791666666666666852, 0.4895833333333333148, 0.5000000000000000000, 0.5104166666666666297, 0.5208333333333333703, 0.5312500000000000000, 0.5416666666666666297, 0.5520833333333333703, 0.5625000000000000000, 0.5729166666666666297, 0.5833333333333333703, 0.5937500000000000000, 0.6041666666666666297, 0.6145833333333333703, 0.6250000000000000000, 0.6354166666666666297, 0.6458333333333333703, 0.6562500000000000000, 0.6666666666666666297, 0.6770833333333333703, 0.6875000000000000000, 0.6979166666666666297, 0.7083333333333333703, 0.7187500000000000000, 0.7291666666666666297, 0.7395833333333333703, 0.7500000000000000000, 0.7604166666666666297, 0.7708333333333333703, 0.7812500000000000000, 0.7916666666666666297, 0.8020833333333333703, 0.8125000000000000000, 0.8229166666666666297, 0.8333333333333333703, 0.8437500000000000000, 0.8541666666666666297, 0.8645833333333333703, 0.8750000000000000000, 0.8854166666666666297, 0.8958333333333333703, 0.9062500000000000000, 0.9166666666666666297, 0.9270833333333333703, 0.9375000000000000000, 0.9448586970929392370 ),
 .UNSPECIFIED. ) 
 GEOMETRIC_REPRESENTATION_ITEM ( )  RATIONAL_B_SPLINE_SURFACE ( (
 ( 1.000000000000000000, 0.9238795325112867385, 1.000000000000000000, 0.9238795325112867385, 1.000000000000000000, 0.9238795325112867385, 1.000000000000000000, 0.9238795325112867385, 1.000000000000000000, 0.9238795325112867385, 1.000000000000000000, 0.9238795325112867385, 1.000000000000000000, 0.9238795325112867385, 1.000000000000000000, 0.9238795325112867385, 1.000000000000000000, 0.9238795325112867385, 1.000000000000000000, 0.9238795325112867385, 1.000000000000000000, 0.9238795325112867385, 1.000000000000000000, 0.9238795325112867385, 1.000000000000000000, 0.9238795325112867385, 1.000000000000000000, 0.9238795325112867385, 1.000000000000000000, 0.9238795325112867385, 1.000000000000000000, 0.9238795325112867385, 1.000000000000000000, 0.9238795325112867385, 1.000000000000000000, 0.9238795325112867385, 1.000000000000000000, 0.9238795325112867385, 1.000000000000000000, 0.9238795325112867385, 1.000000000000000000, 0.9238795325112867385, 1.000000000000000000, 0.9238795325112867385, 1.000000000000000000, 0.9238795325112867385, 1.000000000000000000, 0.9238795325112867385, 1.000000000000000000, 0.9238795325112867385, 1.000000000000000000, 0.9238795325112867385, 1.000000000000000000, 0.9238795325112867385, 1.000000000000000000, 0.9238795325112867385, 1.000000000000000000, 0.9238795325112867385, 1.000000000000000000, 0.9238795325112867385, 1.000000000000000000, 0.9238795325112867385, 1.000000000000000000, 0.9238795325112867385, 1.000000000000000000, 0.9238795325112867385, 1.000000000000000000, 0.9238795325112867385, 1.000000000000000000, 0.9238795325112867385, 1.000000000000000000, 0.9238795325112867385, 1.000000000000000000, 0.9238795325112867385, 1.000000000000000000, 0.9238795325112867385, 1.000000000000000000, 0.9238795325112867385, 1.000000000000000000, 0.9238795325112867385, 1.000000000000000000, 0.9238795325112867385, 1.000000000000000000, 0.9238795325112867385, 1.000000000000000000, 0.9238795325112867385, 1.000000000000000000, 0.9238795325112867385, 1.000000000000000000, 0.9238795325112867385, 1.000000000000000000, 0.9238795325112867385, 1.000000000000000000, 0.9238795325112867385, 1.000000000000000000, 0.9238795325112867385, 1.000000000000000000, 0.9238795325112867385, 1.000000000000000000, 0.9238795325112867385, 1.000000000000000000, 0.9238795325112867385, 1.000000000000000000, 0.9238795325112867385, 1.000000000000000000, 0.9238795325112867385, 1.000000000000000000, 0.9238795325112867385, 1.000000000000000000, 0.9238795325112867385, 1.000000000000000000, 0.9238795325112867385, 1.000000000000000000, 0.9238795325112867385, 1.000000000000000000, 0.9238795325112867385, 1.000000000000000000, 0.9238795325112867385, 1.000000000000000000, 0.9238795325112867385, 1.000000000000000000, 0.9238795325112867385, 1.000000000000000000, 0.9238795325112867385, 1.000000000000000000, 0.9238795325112867385, 1.000000000000000000, 0.9238795325112867385, 1.000000000000000000, 0.9238795325112867385, 1.000000000000000000, 0.9238795325112867385, 1.000000000000000000, 0.9238795325112867385, 1.000000000000000000, 0.9238795325112867385, 1.000000000000000000, 0.9238795325112867385, 1.000000000000000000, 0.9238795325112867385, 1.000000000000000000, 0.9238795325112867385, 1.000000000000000000, 0.9238795325112867385, 1.000000000000000000, 0.9238795325112867385, 1.000000000000000000, 0.9238795325112867385, 1.000000000000000000, 0.9238795325112867385, 1.000000000000000000, 0.9238795325112867385, 1.000000000000000000, 0.9238795325112867385, 1.000000000000000000, 0.9238795325112867385, 1.000000000000000000, 0.9238795325112867385, 1.000000000000000000, 0.9238795325112867385, 1.000000000000000000, 0.9238795325112867385, 1.000000000000000000, 0.9238795325112867385, 1.000000000000000000, 0.9238795325112867385, 1.000000000000000000, 0.9238795325112867385, 1.000000000000000000, 0.9238795325112867385, 1.000000000000000000, 0.9238795325112867385, 1.000000000000000000, 0.9238795325112867385, 1.000000000000000000, 0.9238795325112867385, 1.000000000000000000, 0.9238795325112867385, 1.000000000000000000, 0.9238795325112867385, 1.000000000000000000, 0.9462258435690522607, 0.9684275710300105366),
 ( 1.000000000000000000, 0.9238795325112867385, 1.000000000000000000, 0.9238795325112867385, 1.000000000000000000, 0.9238795325112867385, 1.000000000000000000, 0.9238795325112867385, 1.000000000000000000, 0.9238795325112867385, 1.000000000000000000, 0.9238795325112867385, 1.000000000000000000, 0.9238795325112867385, 1.000000000000000000, 0.9238795325112867385, 1.000000000000000000, 0.9238795325112867385, 1.000000000000000000, 0.9238795325112867385, 1.000000000000000000, 0.9238795325112867385, 1.000000000000000000, 0.9238795325112867385, 1.000000000000000000, 0.9238795325112867385, 1.000000000000000000, 0.9238795325112867385, 1.000000000000000000, 0.9238795325112867385, 1.000000000000000000, 0.9238795325112867385, 1.000000000000000000, 0.9238795325112867385, 1.000000000000000000, 0.9238795325112867385, 1.000000000000000000, 0.9238795325112867385, 1.000000000000000000, 0.9238795325112867385, 1.000000000000000000, 0.9238795325112867385, 1.000000000000000000, 0.9238795325112867385, 1.000000000000000000, 0.9238795325112867385, 1.000000000000000000, 0.9238795325112867385, 1.000000000000000000, 0.9238795325112867385, 1.000000000000000000, 0.9238795325112867385, 1.000000000000000000, 0.9238795325112867385, 1.000000000000000000, 0.9238795325112867385, 1.000000000000000000, 0.9238795325112867385, 1.000000000000000000, 0.9238795325112867385, 1.000000000000000000, 0.9238795325112867385, 1.000000000000000000, 0.9238795325112867385, 1.000000000000000000, 0.9238795325112867385, 1.000000000000000000, 0.9238795325112867385, 1.000000000000000000, 0.9238795325112867385, 1.000000000000000000, 0.9238795325112867385, 1.000000000000000000, 0.9238795325112867385, 1.000000000000000000, 0.9238795325112867385, 1.000000000000000000, 0.9238795325112867385, 1.000000000000000000, 0.9238795325112867385, 1.000000000000000000, 0.9238795325112867385, 1.000000000000000000, 0.9238795325112867385, 1.000000000000000000, 0.9238795325112867385, 1.000000000000000000, 0.9238795325112867385, 1.000000000000000000, 0.9238795325112867385, 1.000000000000000000, 0.9238795325112867385, 1.000000000000000000, 0.9238795325112867385, 1.000000000000000000, 0.9238795325112867385, 1.000000000000000000, 0.9238795325112867385, 1.000000000000000000, 0.9238795325112867385, 1.000000000000000000, 0.9238795325112867385, 1.000000000000000000, 0.9238795325112867385, 1.000000000000000000, 0.9238795325112867385, 1.000000000000000000, 0.9238795325112867385, 1.000000000000000000, 0.9238795325112867385, 1.000000000000000000, 0.9238795325112867385, 1.000000000000000000, 0.9238795325112867385, 1.000000000000000000, 0.9238795325112867385, 1.000000000000000000, 0.9238795325112867385, 1.000000000000000000, 0.9238795325112867385, 1.000000000000000000, 0.9238795325112867385, 1.000000000000000000, 0.9238795325112867385, 1.000000000000000000, 0.9238795325112867385, 1.000000000000000000, 0.9238795325112867385, 1.000000000000000000, 0.9238795325112867385, 1.000000000000000000, 0.9238795325112867385, 1.000000000000000000, 0.9238795325112867385, 1.000000000000000000, 0.9238795325112867385, 1.000000000000000000, 0.9238795325112867385, 1.000000000000000000, 0.9238795325112867385, 1.000000000000000000, 0.9238795325112867385, 1.000000000000000000, 0.9238795325112867385, 1.000000000000000000, 0.9238795325112867385, 1.000000000000000000, 0.9238795325112867385, 1.000000000000000000, 0.9238795325112867385, 1.000000000000000000, 0.9238795325112867385, 1.000000000000000000, 0.9238795325112867385, 1.000000000000000000, 0.9238795325112867385, 1.000000000000000000, 0.9238795325112867385, 1.000000000000000000, 0.9238795325112867385, 1.000000000000000000, 0.9238795325112867385, 1.000000000000000000, 0.9238795325112867385, 1.000000000000000000, 0.9238795325112867385, 1.000000000000000000, 0.9238795325112867385, 1.000000000000000000, 0.9238795325112867385, 1.000000000000000000, 0.9238795325112867385, 1.000000000000000000, 0.9238795325112867385, 1.000000000000000000, 0.9238795325112867385, 1.000000000000000000, 0.9238795325112867385, 1.000000000000000000, 0.9238795325112867385, 1.000000000000000000, 0.9462258435690522607, 0.9684275710300105366) ) ) 
 REPRESENTATION_ITEM ( '' )  SURFACE ( )  );
#10421=CARTESIAN_POINT ( 'NONE',  ( 98.15313185440923860, 81.87500000136560629, 4.458734124999987891 ) ) ;
#10428=CARTESIAN_POINT ( 'NONE',  ( 102.0710678118654329, 83.43750000273121259, 4.999999999999989342 ) ) ;
#10433=CARTESIAN_POINT ( 'NONE',  ( 51.85481384221820633, 38.32109375108394289, -5.444914386472297529 ) ) ;
#10434=AXIS2_PLACEMENT_3D ( 'NONE', #18412, #5866, #10249 ) ;
#10436=DIRECTION ( 'NONE',  ( 0.000000000000000000, -0.000000000000000000, 1.000000000000000000 ) ) ;
#10439=CARTESIAN_POINT ( 'NONE',  ( -6.412866676253197618, 50.00000000108475717, -11.99502265407683943 ) ) ;
#10440=CARTESIAN_POINT ( 'NONE',  ( 99.99999999999995737, 80.87500000273119838, -5.000000000000018652 ) ) ;
#10441=AXIS2_PLACEMENT_3D ( 'NONE', #21439, #6593, #10586 ) ;
#10442=CARTESIAN_POINT ( 'NONE',  ( 116.4251840539369596, 34.00507812716787015, 5.622872871577880183 ) ) ;
#10443=CARTESIAN_POINT ( 'NONE',  ( 59.55508561352770158, 39.80937500108392868, -13.14518615778179900 ) ) ;
#10445=CARTESIAN_POINT ( 'NONE',  ( 204.2950502721270425, 39.46210937608393721, 9.295050272127046043 ) ) ;
#10448=ORIENTED_EDGE ( 'NONE', *, *, #4953, .F. ) ;
#10452=CARTESIAN_POINT ( 'NONE',  ( 5.622872871577742515, 39.66054687500000142, 13.57481594606318076 ) ) ;
#10453=CARTESIAN_POINT ( 'NONE',  ( 103.1528011352953342, 84.06250000136560629, -3.152801135295383084 ) ) ;
#10458=DIRECTION ( 'NONE',  ( 1.000000000000000000, 0.000000000000000000, -3.469446951953613696E-16 ) ) ;
#10459=LINE ( 'NONE', #21170, #7597 ) ;
#10460=ORIENTED_EDGE ( 'NONE', *, *, #25852, .F. ) ;
#10464=CARTESIAN_POINT ( 'NONE',  ( 124.5550856135277087, 37.72578125108395142, 13.14518615778179722 ) ) ;
#10465=CARTESIAN_POINT ( 'NONE',  ( 74.29505027212704249, 37.87460937608393152, -9.295050272127046043 ) ) ;
#10466=CARTESIAN_POINT ( 'NONE',  ( 189.5550856135277229, 39.01562500108394005, -13.14518615778179900 ) ) ;
#10467=CARTESIAN_POINT ( 'NONE',  ( 51.94161814354912110, 36.00000000000000000, 1.569311539113921405 ) ) ;
#10468=CARTESIAN_POINT ( 'NONE',  ( -8.049105076161786076E-16, 36.38632812608393152, -13.14518615778179544 ) ) ;
#10472=AXIS2_PLACEMENT_3D ( 'NONE', #6844, #2731, #736 ) ;
#10473=CARTESIAN_POINT ( 'NONE',  ( -5.444914386472297529, 38.81718750108393579, -13.14518615778179900 ) ) ;
#10474=CARTESIAN_POINT ( 'NONE',  ( 7.616525325480809627, 54.91574374957784244, 14.99999999999999467 ) ) ;
#10488=CARTESIAN_POINT ( 'NONE',  ( 96.84719886470459471, 84.56250000136560629, -3.152801135295383084 ) ) ;
#10489=CARTESIAN_POINT ( 'NONE',  ( 70.44491438647230552, 38.12265625108393152, -13.14518615778179900 ) ) ;
#10490=EDGE_CURVE ( 'NONE', #27733, #23414, #24415, .T. ) ;
#10495=CARTESIAN_POINT ( 'NONE',  ( 55.40115559117954547, 38.81718750216787583, 9.598844408820459861 ) ) ;
#10497=CARTESIAN_POINT ( 'NONE',  ( 116.8548138422182205, 32.81445312608393294, 0.000000000000000000 ) ) ;
#10499=DIRECTION ( 'NONE',  ( 1.000000000000000000, -0.000000000000000000, -7.228014483236696740E-18 ) ) ;
#10502=CARTESIAN_POINT ( 'NONE',  ( 130.0000000000000000, 39.56132812608393579, -13.14518615778179544 ) ) ;
#10503=CARTESIAN_POINT ( 'NONE',  ( 59.37712712842213136, 35.69179687716786731, 13.57481594606304753 ) ) ;
#10506=CARTESIAN_POINT ( 'NONE',  ( -13.57481594606304576, 34.79882812716787299, 5.622872871577880183 ) ) ;
#10510=EDGE_CURVE ( 'NONE', #5473, #6416, #22255, .T. ) ;
#10511=CARTESIAN_POINT ( 'NONE',  ( 208.1451861577817795, 38.51953125108393294, 5.444914386472293977 ) ) ;
#10513=CARTESIAN_POINT ( 'NONE',  ( 120.7049497278729575, 38.86679687608393863, -9.295050272127046043 ) ) ;
#10514=DIRECTION ( 'NONE',  ( -0.000000000000000000, 1.000000000000000000, -0.000000000000000000 ) ) ;
#10519=ADVANCED_FACE ( 'NONE', ( #10040 ), #14594, .T. ) ;
#10520=CARTESIAN_POINT ( 'NONE',  ( 181.4251840539369596, 36.18789062499999432, -5.622872871577873077 ) ) ;
#10522=CARTESIAN_POINT ( 'NONE',  ( 126.8638263786525044, 36.00000000000000711, 12.79489613812760851 ) ) ;
#10524=CARTESIAN_POINT ( 'NONE',  ( 55.70494972787295751, 38.07304687608393579, -9.295050272127046043 ) ) ;
#10529=FACE_BOUND ( 'NONE', #3637, .T. ) ;
#10530=CARTESIAN_POINT ( 'NONE',  ( -9.598844408820458085, 40.90078124999999432, -9.598844408820458085 ) ) ;
#10533=ORIENTED_EDGE ( 'NONE', *, *, #11012, .F. ) ;
#10534=CARTESIAN_POINT ( 'NONE',  ( 103.1528011352953342, 83.06250000136560629, 3.152801135295355106 ) ) ;
#10535=ORIENTED_EDGE ( 'NONE', *, *, #24994, .T. ) ;
#10538=CARTESIAN_POINT ( 'NONE',  ( 78.14518615778179367, 35.54296875108394715, 5.444914386472293977 ) ) ;
#10545=CARTESIAN_POINT ( 'NONE',  ( 181.4251840539369596, 36.33671875216787583, 0.000000000000000000 ) ) ;
#10547=DIRECTION ( 'NONE',  ( 0.8660254037844407060, 0.4999999999999963363, 0.000000000000000000 ) ) ;
#10548=CARTESIAN_POINT ( 'NONE',  ( 190.9374164594231615, 50.00000000116092735, 12.98908657125209665 ) ) ;
#10549=ADVANCED_FACE ( 'NONE', ( #8328 ), #27322, .T. ) ;
#10550=CARTESIAN_POINT ( 'NONE',  ( 143.1451861577818079, 38.76757812608393294, -1.609821015232357215E-15 ) ) ;
#10551=CARTESIAN_POINT ( 'NONE',  ( -13.14518615778179544, 37.57695312608393579, 0.000000000000000000 ) ) ;
#10553=CARTESIAN_POINT ( 'NONE',  ( 74.59884440882045453, 38.32109374999999574, -9.598844408820458085 ) ) ;
#10557=CARTESIAN_POINT ( 'NONE',  ( 94.99999999999995737, 84.12500000273119838, -1.387778780781445676E-14 ) ) ;
#10559=EDGE_CURVE ( 'NONE', #2183, #13505, #18669, .T. ) ;
#10562=CARTESIAN_POINT ( 'NONE',  ( 101.8468681455907046, 80.00000000136560629, 4.458734124999987891 ) ) ;
#10564=CARTESIAN_POINT ( 'NONE',  ( -13.14518615778179189, 38.42031250108393436, 5.444914386472304635 ) ) ;
#10567=EDGE_LOOP ( 'NONE', ( #18325, #19276 ) ) ;
#10569=DIRECTION ( 'NONE',  ( -0.000000000000000000, 1.000000000000000000, -0.000000000000000000 ) ) ;
#10573=CARTESIAN_POINT ( 'NONE',  ( 185.7049497278729575, 39.66054687608393436, -9.295050272127046043 ) ) ;
#10574=EDGE_LOOP ( 'NONE', ( #20522, #21819, #9847, #5998 ) ) ;
#10575=DIRECTION ( 'NONE',  ( 1.000000000000000000, 0.000000000000000000, -2.385244779468110248E-16 ) ) ;
#10577=CARTESIAN_POINT ( 'NONE',  ( 58.92091997948118376, 54.65154858643462887, -15.00000000000000355 ) ) ;
#10580=CARTESIAN_POINT ( 'NONE',  ( -9.180175813648011385, 50.00000000000000000, -9.999999999999978684 ) ) ;
#10583=CARTESIAN_POINT ( 'NONE',  ( 116.4251840539369596, 35.54296875216788010, 0.000000000000000000 ) ) ;
#10584=( BOUNDED_SURFACE ( )  B_SPLINE_SURFACE ( 3, 2, ( 
 ( #23740, #2225, #28019 ),
 ( #23876, #12872, #17312 ),
 ( #21602, #8485, #6764 ),
 ( #8341, #14881, #2080 ),
 ( #24020, #19459, #4498 ),
 ( #25876, #79, #26012 ),
 ( #4354, #4215, #15447 ),
 ( #6619, #2367, #25729 ),
 ( #17595, #6483, #26302 ),
 ( #23596, #2503, #13010 ),
 ( #24162, #11024, #19736 ),
 ( #10889, #19177, #8906 ),
 ( #22025, #12741, #4639 ),
 ( #21749, #10748, #19596 ),
 ( #13298, #27880, #26152 ),
 ( #17027, #21465, #1942 ),
 ( #10611, #19318, #17174 ),
 ( #15020, #28157, #15304 ),
 ( #20030, #940, #11164 ),
 ( #16015, #5351, #24585 ) ),
 .UNSPECIFIED., .F., .F., .T. ) 
 B_SPLINE_SURFACE_WITH_KNOTS ( ( 4, 2, 2, 2, 2, 2, 2, 2, 2, 4 ),
 ( 3, 3 ),
 ( 0.009073803551359458167, 0.01139250602759180747, 0.01371120850382415851, 0.01602991098005650955, 0.01834861345628885712, 0.01950796469440502917, 0.02066731593252120469, 0.02298601840875355573, 0.02530472088498590677, 0.02762342336121825434 ),
 ( 0.000000000000000000, 1.000000000000000000 ),
 .UNSPECIFIED. ) 
 GEOMETRIC_REPRESENTATION_ITEM ( )  RATIONAL_B_SPLINE_SURFACE ( (
 ( 1.000000000000000000, 0.7071067811865482389, 1.000000000000000000),
 ( 1.000000000000000000, 0.7344871497829537077, 1.000000000000000000),
 ( 1.000000000000000000, 0.7612510203318018087, 1.000000000000000000),
 ( 1.000000000000000000, 0.8116663633844866110, 1.000000000000000000),
 ( 1.000000000000000000, 0.8353358059749917963, 1.000000000000000000),
 ( 1.000000000000000000, 0.8764699612587962818, 1.000000000000000000),
 ( 1.000000000000000000, 0.8939017358718740480, 1.000000000000000000),
 ( 1.000000000000000000, 0.9185314935647553858, 1.000000000000000000),
 ( 1.000000000000000000, 0.9256439951239483488, 1.000000000000000000),
 ( 1.000000000000000000, 0.9261623622476518047, 1.000000000000000000),
 ( 1.000000000000000000, 0.9246301385978411558, 1.000000000000000000),
 ( 1.000000000000000000, 0.9183304321348458865, 1.000000000000000000),
 ( 1.000000000000000000, 0.9135987334167114948, 1.000000000000000000),
 ( 1.000000000000000000, 0.8954110486042292649, 1.000000000000000000),
 ( 1.000000000000000000, 0.8779877431164835322, 1.000000000000000000),
 ( 1.000000000000000000, 0.8366182664708665673, 1.000000000000000000),
 ( 1.000000000000000000, 0.8126941604013132592, 1.000000000000000000),
 ( 1.000000000000000000, 0.7617527316308130292, 1.000000000000000000),
 ( 1.000000000000000000, 0.7347103785790367603, 1.000000000000000000),
 ( 1.000000000000000000, 0.7071067811865459074, 1.000000000000000000) ) ) 
 REPRESENTATION_ITEM ( '' )  SURFACE ( )  );
#10585=CARTESIAN_POINT ( 'NONE',  ( 102.0710678118654045, 81.43750000273119838, 5.000000000000019540 ) ) ;
#10586=DIRECTION ( 'NONE',  ( 0.000000000000000000, 0.000000000000000000, 1.000000000000000000 ) ) ;
#10587=CARTESIAN_POINT ( 'NONE',  ( 200.4449143864723055, 34.65000000108393863, 13.14518615778179189 ) ) ;
#10588=VERTEX_POINT ( 'NONE', #4342 ) ;
#10589=ORIENTED_EDGE ( 'NONE', *, *, #151, .T. ) ;
#10592=CARTESIAN_POINT ( 'NONE',  ( 97.92893218813449607, 84.18750000000000000, 4.999999999999981348 ) ) ;
#10593=CARTESIAN_POINT ( 'NONE',  ( 51.85481384221821344, 39.80937500108393579, 5.444914386472304635 ) ) ;
#10594=CARTESIAN_POINT ( 'NONE',  ( 51.42518405393695957, 36.38632812716788578, 5.622872871577880183 ) ) ;
#10599=CARTESIAN_POINT ( 'NONE',  ( 189.5550856135277229, 39.80937500108393579, -13.14518615778179722 ) ) ;
#10602=VERTEX_POINT ( 'NONE', #9037 ) ;
#10606=CARTESIAN_POINT ( 'NONE',  ( 116.8548138422182205, 37.57695312608393579, 0.000000000000000000 ) ) ;
#10607=CARTESIAN_POINT ( 'NONE',  ( 78.14518615778179367, 36.23750000108393010, -5.444914386472297529 ) ) ;
#10608=CARTESIAN_POINT ( 'NONE',  ( 208.1451861577817795, 32.26875000108393721, -5.444914386472297529 ) ) ;
#10610=CARTESIAN_POINT ( 'NONE',  ( 13.14518615778179544, 34.60039062608392868, -1.609821015232357215E-15 ) ) ;
#10611=CARTESIAN_POINT ( 'NONE',  ( 122.9105827276628418, 49.99999999943648987, -11.59823041028630364 ) ) ;
#10613=DIRECTION ( 'NONE',  ( -0.000000000000000000, 1.000000000000000000, -0.000000000000000000 ) ) ;
#10614=CARTESIAN_POINT ( 'NONE',  ( -8.049105076161786076E-16, 39.56132812608393579, -13.14518615778179544 ) ) ;
#10615=( BOUNDED_CURVE ( )  B_SPLINE_CURVE ( 2, ( #25593, #17175, #23464, #27606, #25317, #12601, #12330, #21326, #23191 ),
 .UNSPECIFIED., .F., .F. ) 
 B_SPLINE_CURVE_WITH_KNOTS ( ( 3, 2, 2, 2, 3 ),
 ( 0.06250000000000004163, 0.07291666666666665741, 0.08333333333333325932, 0.09374999999999987510, 0.1041666666666664909 ),
 .UNSPECIFIED. ) 
 CURVE ( )  GEOMETRIC_REPRESENTATION_ITEM ( )  RATIONAL_B_SPLINE_CURVE ( ( 0.9999999999999996669, 0.9238795325112870716, 1.000000000000000000, 0.9238795325112867385, 1.000000000000000000, 0.9238795325112867385, 1.000000000000000000, 0.9238795325112880708, 0.9999999999999986677 ) ) 
 REPRESENTATION_ITEM ( '' )  );
#10616=CARTESIAN_POINT ( 'NONE',  ( 1.887528725876407965, 53.66306546785492060, 14.99999999999999822 ) ) ;
#10618=CARTESIAN_POINT ( 'NONE',  ( 61.28346588621581503, 51.46663580899082291, 14.99999999999794298 ) ) ;
#10627=CARTESIAN_POINT ( 'NONE',  ( 120.4011555911795455, 38.81718750216787583, 9.598844408820459861 ) ) ;
#10628=CARTESIAN_POINT ( 'NONE',  ( 101.8468681455906903, 80.75000000136560629, 4.458734124999987891 ) ) ;
#10629=CARTESIAN_POINT ( 'NONE',  ( 55.70494972787295751, 39.06523437608392868, -9.295050272127046043 ) ) ;
#10631=CARTESIAN_POINT ( 'NONE',  ( -5.444914386472299306, 39.90859375108392726, 13.14518615778179722 ) ) ;
#10632=DIRECTION ( 'NONE',  ( 0.000000000000000000, 0.000000000000000000, 1.000000000000000000 ) ) ;
#10635=CARTESIAN_POINT ( 'NONE',  ( 139.2950502721270425, 32.51679687608393721, -9.295050272127046043 ) ) ;
#10637=LINE ( 'NONE', #6374, #10827 ) ;
#10639=CARTESIAN_POINT ( 'NONE',  ( 95.54126587499995082, 81.37500000136563472, -1.846868145590750077 ) ) ;
#10640=CARTESIAN_POINT ( 'NONE',  ( 130.0000000000000000, 36.38632812608393152, -13.14518615778179544 ) ) ;
#10641=CARTESIAN_POINT ( 'NONE',  ( 70.62287287157786864, 37.67617187716787441, -13.57481594606304753 ) ) ;
#10643=EDGE_CURVE ( 'NONE', #27310, #1696, #11150, .T. ) ;
#10645=CARTESIAN_POINT ( 'NONE',  ( 9.598844408820459861, 35.04687500216787299, 9.598844408820456309 ) ) ;
#10648=CARTESIAN_POINT ( 'NONE',  ( 181.8548138422181921, 36.53515625108392584, -5.444914386472297529 ) ) ;
#10649=CARTESIAN_POINT ( 'NONE',  ( 78.57481594606305464, 39.06523437499999574, -5.622872871577873966 ) ) ;
#10652=CARTESIAN_POINT ( 'NONE',  ( 208.5748159460630688, 39.11484375216787157, -1.662435489736055892E-15 ) ) ;
#10653=CARTESIAN_POINT ( 'NONE',  ( 65.00000000000000000, 36.83281249999999574, -13.57481594606304576 ) ) ;
#10656=CARTESIAN_POINT ( 'NONE',  ( 200.6228728715778686, 38.07304687499998863, 13.57481594606304576 ) ) ;
#10660=CARTESIAN_POINT ( 'NONE',  ( 51.85481384221820633, 37.42812500108393436, 5.444914386472304635 ) ) ;
#10665=CARTESIAN_POINT ( 'NONE',  ( -13.57481594606304753, 38.56914062500000284, -5.622872871577873077 ) ) ;
#10666=CARTESIAN_POINT ( 'NONE',  ( 124.5550856135277087, 40.10703125108393152, 13.14518615778179722 ) ) ;
#10668=CARTESIAN_POINT ( 'NONE',  ( 99.99999999999995737, 83.25000000000000000, 4.999999999999990230 ) ) ;
#10670=ORIENTED_EDGE ( 'NONE', *, *, #27379, .F. ) ;
#10671=CARTESIAN_POINT ( 'NONE',  ( 195.0000000000000000, 37.72578125216787726, -13.57481594606304576 ) ) ;
#10672=CARTESIAN_POINT ( 'NONE',  ( 59.55508561352770158, 33.45937500108394147, -13.14518615778179900 ) ) ;
#10674=ADVANCED_FACE ( 'NONE', ( #8611 ), #17583, .T. ) ;
#10675=CARTESIAN_POINT ( 'NONE',  ( 126.9606029491974510, 53.88964894337311762, -14.99999999999999822 ) ) ;
#10678=ORIENTED_EDGE ( 'NONE', *, *, #4769, .T. ) ;
#10681=CARTESIAN_POINT ( 'NONE',  ( 189.3771271284221314, 36.18789062716787441, -13.57481594606304753 ) ) ;
#10685=CARTESIAN_POINT ( 'NONE',  ( 124.5550856135277087, 38.51953125108393294, 13.14518615778179722 ) ) ;
#10686=CARTESIAN_POINT ( 'NONE',  ( 5.444914386472297529, 38.91640625108393436, -13.14518615778179900 ) ) ;
#10687=AXIS2_PLACEMENT_3D ( 'NONE', #25152, #16457, #5642 ) ;
#10688=CARTESIAN_POINT ( 'NONE',  ( 120.7049497278729575, 34.30273437608393294, 9.295050272127047819 ) ) ;
#10689=CARTESIAN_POINT ( 'NONE',  ( 78.57481594606304043, 39.06523437499998863, -5.622872871577873077 ) ) ;
#10690=CARTESIAN_POINT ( 'NONE',  ( 116.8548138422182205, 40.55351562608393579, 0.000000000000000000 ) ) ;
#10696=DIRECTION ( 'NONE',  ( -1.000000000000000000, 0.000000000000000000, 0.000000000000000000 ) ) ;
#10698=CARTESIAN_POINT ( 'NONE',  ( 103.1528011352953342, 80.31250000136559208, -3.152801135295383084 ) ) ;
#10700=CARTESIAN_POINT ( 'NONE',  ( -9.295050272127044266, 40.05742187608393579, 9.295050272127047819 ) ) ;
#10704=( BOUNDED_CURVE ( )  B_SPLINE_CURVE ( 2, ( #6620, #15306, #6765, #15983, #17596, #7583, #16276, #24974, #5459 ),
 .UNSPECIFIED., .F., .F. ) 
 B_SPLINE_CURVE_WITH_KNOTS ( ( 3, 2, 2, 2, 3 ),
 ( 0.1875000000000001388, 0.1979166666666667407, 0.2083333333333333703, 0.2187499999999999722, 0.2291666666666665741 ),
 .UNSPECIFIED. ) 
 CURVE ( )  GEOMETRIC_REPRESENTATION_ITEM ( )  RATIONAL_B_SPLINE_CURVE ( ( 0.9999999999999990008, 0.9238795325112877377, 1.000000000000000000, 0.9238795325112867385, 1.000000000000000000, 0.9238795325112867385, 1.000000000000000000, 0.9238795325112872936, 0.9999999999999994449 ) ) 
 REPRESENTATION_ITEM ( '' )  );
#10707=CARTESIAN_POINT ( 'NONE',  ( 181.4251840539369596, 36.18789062499999432, -5.622872871577872189 ) ) ;
#10708=EDGE_CURVE ( 'NONE', #17655, #23999, #197, .T. ) ;
#10709=CARTESIAN_POINT ( 'NONE',  ( 181.8548138422182205, 39.75976562608393294, 0.000000000000000000 ) ) ;
#10714=EDGE_LOOP ( 'NONE', ( #20022, #4712, #19101, #1106 ) ) ;
#10717=AXIS2_PLACEMENT_3D ( 'NONE', #103, #17473, #8785 ) ;
#10719=EDGE_CURVE ( 'NONE', #15111, #28147, #4191, .T. ) ;
#10720=CARTESIAN_POINT ( 'NONE',  ( 116.4251840539369454, 34.69960937716787441, -5.622872871577873077 ) ) ;
#10721=CARTESIAN_POINT ( 'NONE',  ( 70.44491438647230552, 39.71015625108393010, -13.14518615778179900 ) ) ;
#10723=CARTESIAN_POINT ( 'NONE',  ( 189.5550856135277229, 33.75703125108393721, 13.14518615778179722 ) ) ;
#10725=EDGE_LOOP ( 'NONE', ( #27641, #21354, #15523, #7168, #9604, #13466, #16171, #25107, #23025, #1343, #21881, #2188, #12389, #15896, #7602 ) ) ;
#10730=CARTESIAN_POINT ( 'NONE',  ( 65.00000000000000000, 39.56132812608393579, -13.14518615778179544 ) ) ;
#10731=CARTESIAN_POINT ( 'NONE',  ( 95.54126587499996504, 80.50000000136560629, 1.846868145590724986 ) ) ;
#10732=CARTESIAN_POINT ( 'NONE',  ( 181.8548138422182205, 37.37851562608393863, 0.000000000000000000 ) ) ;
#10733=DIRECTION ( 'NONE',  ( 0.000000000000000000, 0.000000000000000000, 1.000000000000000000 ) ) ;
#10736=CARTESIAN_POINT ( 'NONE',  ( 65.00000000000000000, 39.61093749999999147, 13.57481594606304576 ) ) ;
#10738=EDGE_LOOP ( 'NONE', ( #21172, #18691, #27892, #22802 ) ) ;
#10742=CARTESIAN_POINT ( 'NONE',  ( 135.4449143864723055, 37.03125000108393294, 13.14518615778179189 ) ) ;
#10743=CARTESIAN_POINT ( 'NONE',  ( 59.55508561352770158, 34.35234375108392868, 13.14518615778179722 ) ) ;
#10744=CARTESIAN_POINT ( 'NONE',  ( 204.2950502721270425, 38.66835937608393436, 9.295050272127046043 ) ) ;
#10747=CARTESIAN_POINT ( 'NONE',  ( -13.14518615778179544, 32.61601562608393579, 0.000000000000000000 ) ) ;
#10748=CARTESIAN_POINT ( 'NONE',  ( 126.3635037532130951, 51.46815297078914142, -14.99999999999931077 ) ) ;
#10749=AXIS2_PLACEMENT_3D ( 'NONE', #15529, #22249, #9265 ) ;
#10753=CARTESIAN_POINT ( 'NONE',  ( 9.295050272127046043, 37.87460937608393152, -9.295050272127046043 ) ) ;
#10754=AXIS2_PLACEMENT_3D ( 'NONE', #20495, #1255, #7795 ) ;
#10755=CARTESIAN_POINT ( 'NONE',  ( 99.99999999999995737, 85.00000000000000000, -1.387778780781445676E-14 ) ) ;
#10758=EDGE_LOOP ( 'NONE', ( #7915, #10176, #16995, #9514 ) ) ;
#10761=CARTESIAN_POINT ( 'NONE',  ( 125.0749732163386483, 49.99999999893126557, 12.67776588292038653 ) ) ;
#10763=CARTESIAN_POINT ( 'NONE',  ( 116.4251840539369596, 38.71796875216787726, 0.000000000000000000 ) ) ;
#10764=CARTESIAN_POINT ( 'NONE',  ( 99.99999999999995737, 80.93750000136559208, 4.458734124999988779 ) ) ;
#10765=CARTESIAN_POINT ( 'NONE',  ( 74.29505027212704249, 34.69960937608393436, 9.295050272127046043 ) ) ;
#10767=CARTESIAN_POINT ( 'NONE',  ( 9.295050272127046043, 39.46210937608393010, -9.295050272127046043 ) ) ;
#10769=CARTESIAN_POINT ( 'NONE',  ( -20.00000000000000355, 75.00000000000000000, -10.00000000000000000 ) ) ;
#10772=CARTESIAN_POINT ( 'NONE',  ( 124.3771271284221314, 39.26367187499999289, -13.57481594606304753 ) ) ;
#10773=ORIENTED_EDGE ( 'NONE', *, *, #18711, .T. ) ;
#10777=CARTESIAN_POINT ( 'NONE',  ( 120.7049497278729575, 35.09648437608392868, 9.295050272127047819 ) ) ;
#10778=CARTESIAN_POINT ( 'NONE',  ( 59.37712712842213136, 33.80664062716786589, -13.57481594606304753 ) ) ;
#10780=CARTESIAN_POINT ( 'NONE',  ( 13.57481594606304753, 36.78320312716786589, -5.622872871577873077 ) ) ;
#10784=CARTESIAN_POINT ( 'NONE',  ( 181.8548138422181921, 39.01562500108393294, 5.444914386472304635 ) ) ;
#10785=VECTOR ( 'NONE', #15773, 1000.000000000000000 ) ;
#10787=FACE_OUTER_BOUND ( 'NONE', #10983, .T. ) ;
#10791=CARTESIAN_POINT ( 'NONE',  ( 65.00000000000000000, 37.22968749999999716, 13.57481594606304576 ) ) ;
#10794=CARTESIAN_POINT ( 'NONE',  ( 181.4251840539369596, 33.80664062500000000, -5.622872871577873077 ) ) ;
#10795=CARTESIAN_POINT ( 'NONE',  ( 65.00000000000000000, 40.40468749999999432, 13.57481594606304576 ) ) ;
#10796=DIRECTION ( 'NONE',  ( -0.000000000000000000, 1.000000000000000000, -0.000000000000000000 ) ) ;
#10797=CARTESIAN_POINT ( 'NONE',  ( 74.29505027212704249, 39.26367187608393294, 9.295050272127046043 ) ) ;
#10803=CARTESIAN_POINT ( 'NONE',  ( 13.57481594606304576, 36.63437499999999858, -1.662435489736055892E-15 ) ) ;
#10804=CARTESIAN_POINT ( 'NONE',  ( 65.00000000000000000, 36.93203125216787441, -13.57481594606304576 ) ) ;
#10805=VERTEX_POINT ( 'NONE', #23419 ) ;
#10806=CARTESIAN_POINT ( 'NONE',  ( 103.1528011352953342, 80.06250000136559208, 3.152801135295355106 ) ) ;
#10810=CARTESIAN_POINT ( 'NONE',  ( 59.55508561352770158, 36.13828125108393863, 13.14518615778179722 ) ) ;
#10811=ORIENTED_EDGE ( 'NONE', *, *, #4430, .T. ) ;
#10812=CARTESIAN_POINT ( 'NONE',  ( 122.3834746745191921, 54.91574374957785665, -15.00000000000000000 ) ) ;
#10817=CARTESIAN_POINT ( 'NONE',  ( 208.5748159460630688, 37.52734375216787299, -1.662435489736055892E-15 ) ) ;
#10820=CARTESIAN_POINT ( 'NONE',  ( 195.8765262653620596, 51.45968077934941931, 14.99999999999961098 ) ) ;
#10821=CARTESIAN_POINT ( 'NONE',  ( 208.5748159460630688, 39.95820312716787726, -5.622872871577873966 ) ) ;
#10823=CARTESIAN_POINT ( 'NONE',  ( -5.444914386472297529, 37.42812500108394147, -13.14518615778179900 ) ) ;
#10824=CARTESIAN_POINT ( 'NONE',  ( 124.5550856135277087, 35.93984375108392726, 13.14518615778179722 ) ) ;
#10825=CARTESIAN_POINT ( 'NONE',  ( 51.42518405393695957, 35.39414062499999147, -5.622872871577873077 ) ) ;
#10827=VECTOR ( 'NONE', #23764, 1000.000000000000000 ) ;
#10833=DIRECTION ( 'NONE',  ( 0.000000000000000000, 1.000000000000000000, 0.000000000000000000 ) ) ;
#10834=CARTESIAN_POINT ( 'NONE',  ( 98.15313185440923860, 79.87500000136560629, 4.458734124999987891 ) ) ;
#10836=CARTESIAN_POINT ( 'NONE',  ( 2.414731522848535132E-15, 36.18789062608393436, 13.14518615778179544 ) ) ;
#10842=CARTESIAN_POINT ( 'NONE',  ( 195.0000000000000000, 36.03906250000000000, -13.57481594606304576 ) ) ;
#10843=CARTESIAN_POINT ( 'NONE',  ( 185.7049497278729575, 39.06523437608392868, 9.295050272127047819 ) ) ;
#10848=CARTESIAN_POINT ( 'NONE',  ( 56.60778470836161347, 54.99999999999999289, -15.00000000000000178 ) ) ;
#10852=AXIS2_PLACEMENT_3D ( 'NONE', #13013, #6905, #21897 ) ;
#10853=CARTESIAN_POINT ( 'NONE',  ( 99.99999999999995737, 81.37500000273119838, 4.999999999999990230 ) ) ;
#10854=CARTESIAN_POINT ( 'NONE',  ( 120.4011555911795455, 32.26875000216787726, -9.598844408820458085 ) ) ;
#10855=CARTESIAN_POINT ( 'NONE',  ( 65.00000000000000000, -7.395377635281828788, -7.517135062566165128E-15 ) ) ;
#10856=ADVANCED_FACE ( 'NONE', ( #21006 ), #12420, .T. ) ;
#10858=CARTESIAN_POINT ( 'NONE',  ( 51.85481384221819923, 39.90859375108394147, -5.444914386472297529 ) ) ;
#10860=CARTESIAN_POINT ( 'NONE',  ( 204.2950502721270425, 36.28710937608393294, 9.295050272127046043 ) ) ;
#10862=ORIENTED_EDGE ( 'NONE', *, *, #7944, .T. ) ;
#10868=CARTESIAN_POINT ( 'NONE',  ( 55.70494972787295751, 39.06523437608392868, 9.295050272127047819 ) ) ;
#10869=CARTESIAN_POINT ( 'NONE',  ( 96.84719886470459471, 82.56250000136559208, 3.152801135295355994 ) ) ;
#10870=CARTESIAN_POINT ( 'NONE',  ( 200.4449143864723055, 39.21406250108392300, 13.14518615778179189 ) ) ;
#10874=CARTESIAN_POINT ( 'NONE',  ( 65.00000000000000000, 39.71015625216787015, 13.57481594606304576 ) ) ;
#10875=VECTOR ( 'NONE', #13889, 1000.000000000000000 ) ;
#10883=CARTESIAN_POINT ( 'NONE',  ( 120.7049497278729575, 35.09648437608393579, -9.295050272127046043 ) ) ;
#10884=CARTESIAN_POINT ( 'NONE',  ( 51.85481384221819923, 34.94765625108392726, -5.444914386472297529 ) ) ;
#10886=CARTESIAN_POINT ( 'NONE',  ( 208.1451861577817795, 36.43593750108392726, -5.444914386472297529 ) ) ;
#10889=CARTESIAN_POINT ( 'NONE',  ( 127.9753722744671194, 50.00000000050989968, -13.43320860980974807 ) ) ;
#10891=CARTESIAN_POINT ( 'NONE',  ( 143.5748159460630404, 39.95820312716787726, -5.622872871577873077 ) ) ;
#10893=CARTESIAN_POINT ( 'NONE',  ( 9.295050272127046043, 33.90585937608393152, -9.295050272127046043 ) ) ;
#10894=CARTESIAN_POINT ( 'NONE',  ( 9.180175813647995398, 50.00000000000000000, 9.999999999999994671 ) ) ;
#10904=CYLINDRICAL_SURFACE ( 'NONE', #10364, 13.57481594606304398 ) ;
#10905=CARTESIAN_POINT ( 'NONE',  ( 99.99999999999995737, 81.93750000136559208, 4.458734124999988779 ) ) ;
#10906=CARTESIAN_POINT ( 'NONE',  ( 59.55508561352770158, 34.25312500108393010, -13.14518615778179900 ) ) ;
#10908=FACE_OUTER_BOUND ( 'NONE', #2512, .T. ) ;
#10909=CARTESIAN_POINT ( 'NONE',  ( -15.00000000000000355, 75.00000000000000000, -9.999999999999998224 ) ) ;
#10912=CARTESIAN_POINT ( 'NONE',  ( 130.0000000000000000, 38.02343749999999289, 13.57481594606304576 ) ) ;
#10915=LINE ( 'NONE', #4105, #1750 ) ;
#10919=CARTESIAN_POINT ( 'NONE',  ( 116.8548138422182063, 35.74140625108393721, -5.444914386472297529 ) ) ;
#10920=CARTESIAN_POINT ( 'NONE',  ( 74.59884440882045453, 35.24531250216787726, -9.598844408820458085 ) ) ;
#10923=CARTESIAN_POINT ( 'NONE',  ( -13.14518615778179544, 40.55351562608393579, 0.000000000000000000 ) ) ;
#10926=CARTESIAN_POINT ( 'NONE',  ( 200.4449143864723055, 33.95546875108393436, -13.14518615778179900 ) ) ;
#10927=DIRECTION ( 'NONE',  ( 0.000000000000000000, 0.000000000000000000, -1.000000000000000000 ) ) ;
#10930=CARTESIAN_POINT ( 'NONE',  ( 195.0000000000000000, 39.31328125216787583, -13.57481594606304576 ) ) ;
#10935=CARTESIAN_POINT ( 'NONE',  ( 208.5748159460630688, 35.84062499999999574, -1.662435489736055892E-15 ) ) ;
#10937=CARTESIAN_POINT ( 'NONE',  ( 74.29505027212704249, 37.08085937608393579, -9.295050272127046043 ) ) ;
#10942=CARTESIAN_POINT ( 'NONE',  ( 13.57481594606304576, 35.04687499999999289, -1.662435489736055892E-15 ) ) ;
#10943=CARTESIAN_POINT ( 'NONE',  ( 116.8548138422182205, 37.57695312608393579, 0.000000000000000000 ) ) ;
#10945=ORIENTED_EDGE ( 'NONE', *, *, #3383, .T. ) ;
#10946=CARTESIAN_POINT ( 'NONE',  ( 96.46446609406721961, 82.87500000000000000, -3.535533905932755072 ) ) ;
#10948=CARTESIAN_POINT ( 'NONE',  ( 102.0710678118654329, 82.81250000273119838, -5.000000000000018652 ) ) ;
#10950=CARTESIAN_POINT ( 'NONE',  ( 57.60596795766428357, 36.00000000000002842, -11.20317769887112647 ) ) ;
#10953=CARTESIAN_POINT ( 'NONE',  ( 74.29505027212704249, 35.69179687608394147, -9.295050272127046043 ) ) ;
#10955=AXIS2_PLACEMENT_3D ( 'NONE', #7224, #15489, #21932 ) ;
#10959=CARTESIAN_POINT ( 'NONE',  ( 96.46446609406721961, 82.00000000273119838, -3.535533905932755072 ) ) ;
#10961=CARTESIAN_POINT ( 'NONE',  ( 181.4251840539369596, 37.87460937716787868, -5.622872871577873077 ) ) ;
#10963=LINE ( 'NONE', #19674, #23071 ) ;
#10964=CARTESIAN_POINT ( 'NONE',  ( 120.7049497278729575, 36.88242187608393152, 9.295050272127047819 ) ) ;
#10965=CARTESIAN_POINT ( 'NONE',  ( -9.295050272127044266, 39.26367187608393294, 9.295050272127047819 ) ) ;
#10966=CARTESIAN_POINT ( 'NONE',  ( 124.5550856135277087, 36.43593750108392726, -13.14518615778179900 ) ) ;
#10967=CARTESIAN_POINT ( 'NONE',  ( 70.62287287157786864, 35.98945312499999716, -13.57481594606304753 ) ) ;
#10970=CARTESIAN_POINT ( 'NONE',  ( 207.8921516136353773, 35.99999999999997868, -4.169510824908014612 ) ) ;
#10973=CARTESIAN_POINT ( 'NONE',  ( 9.598844408820456309, 39.21406250216787015, -9.598844408820458085 ) ) ;
#10976=CARTESIAN_POINT ( 'NONE',  ( 9.295050272127046043, 35.69179687608394147, -9.295050272127046043 ) ) ;
#10978=VERTEX_POINT ( 'NONE', #1486 ) ;
#10980=DIRECTION ( 'NONE',  ( 0.000000000000000000, 0.000000000000000000, 1.000000000000000000 ) ) ;
#10982=CARTESIAN_POINT ( 'NONE',  ( 181.8548138422181921, 37.42812500108393436, 5.444914386472304635 ) ) ;
#10983=EDGE_LOOP ( 'NONE', ( #17146, #14669, #18388, #24357 ) ) ;
#10984=CARTESIAN_POINT ( 'NONE',  ( 2.385244779468109360E-15, 80.00000000000000000, 9.999999999999996447 ) ) ;
#10985=CARTESIAN_POINT ( 'NONE',  ( 2.493653234604083739E-15, 39.71015625216787015, 13.57481594606304576 ) ) ;
#10986=CARTESIAN_POINT ( 'NONE',  ( 63.49898087569502536, 53.60014735326987534, -15.00000000000000000 ) ) ;
#10991=CARTESIAN_POINT ( 'NONE',  ( 96.46446609406721961, 81.00000000273119838, -3.535533905932755072 ) ) ;
#10992=CARTESIAN_POINT ( 'NONE',  ( 116.4251840539369596, 32.36796875216787583, 0.000000000000000000 ) ) ;
#10993=CARTESIAN_POINT ( 'NONE',  ( 13.14518615778179722, 40.40468750108393436, -5.444914386472297529 ) ) ;
#10995=CARTESIAN_POINT ( 'NONE',  ( 51.85481384221819923, 38.32109375108394289, -5.444914386472297529 ) ) ;
#10997=CARTESIAN_POINT ( 'NONE',  ( 189.5550856135277229, 34.55078125108393294, 13.14518615778179722 ) ) ;
#10998=EDGE_LOOP ( 'NONE', ( #6419, #6770, #25486, #5631 ) ) ;
#10999=ORIENTED_EDGE ( 'NONE', *, *, #24239, .F. ) ;
#11005=CARTESIAN_POINT ( 'NONE',  ( 99.99999999999995737, 81.18750000136559208, -4.458734125000016313 ) ) ;
#11006=CARTESIAN_POINT ( 'NONE',  ( 208.1451861577818079, 38.51953125108393294, 5.444914386472293977 ) ) ;
#11008=DIRECTION ( 'NONE',  ( -1.000000000000000000, 0.000000000000000000, 0.000000000000000000 ) ) ;
#11009=CARTESIAN_POINT ( 'NONE',  ( 208.1451861577818079, 40.30546875108393579, 5.444914386472293977 ) ) ;
#11012=EDGE_CURVE ( 'NONE', #19984, #27020, #9878, .T. ) ;
#11015=ORIENTED_EDGE ( 'NONE', *, *, #27810, .T. ) ;
#11016=CARTESIAN_POINT ( 'NONE',  ( 130.0000000000000000, 36.58476562608393579, -13.14518615778179544 ) ) ;
#11017=CARTESIAN_POINT ( 'NONE',  ( 55.70494972787295751, 34.89804687608393152, -9.295050272127046043 ) ) ;
#11019=CARTESIAN_POINT ( 'NONE',  ( 181.8548138422182205, 35.98945312608393721, 0.000000000000000000 ) ) ;
#11022=CARTESIAN_POINT ( 'NONE',  ( -9.295050272127046043, 33.31054687608393294, -9.295050272127046043 ) ) ;
#11023=( BOUNDED_CURVE ( )  B_SPLINE_CURVE ( 2, ( #21983, #6304, #14980, #23699, #12972, #10707, #21705, #2180, #10842 ),
 .UNSPECIFIED., .F., .T. ) 
 B_SPLINE_CURVE_WITH_KNOTS ( ( 3, 2, 2, 2, 3 ),
 ( 0.4791666666666667962, 0.4895833333333333703, 0.5000000000000000000, 0.5104166666666665186, 0.5208333333333332593 ),
 .UNSPECIFIED. ) 
 CURVE ( )  GEOMETRIC_REPRESENTATION_ITEM ( )  RATIONAL_B_SPLINE_CURVE ( ( 0.9999999999999992228, 0.9238795325112875156, 1.000000000000000000, 0.9238795325112867385, 1.000000000000000000, 0.9238795325112867385, 1.000000000000000000, 0.9238795325112875156, 0.9999999999999992228 ) ) 
 REPRESENTATION_ITEM ( '' )  );
#11024=CARTESIAN_POINT ( 'NONE',  ( 129.1234737346379688, 51.45968077934942642, -15.00000000000033928 ) ) ;
#11025=ADVANCED_FACE ( 'NONE', ( #12140 ), #21679, .T. ) ;
#11027=CARTESIAN_POINT ( 'NONE',  ( 124.3771271284221314, 39.66054687716786731, 13.57481594606304753 ) ) ;
#11033=CARTESIAN_POINT ( 'NONE',  ( 181.8548138422182205, 40.55351562608393579, 0.000000000000000000 ) ) ;
#11036=ORIENTED_EDGE ( 'NONE', *, *, #899, .F. ) ;
#11039=CARTESIAN_POINT ( 'NONE',  ( 130.7238719380277132, 53.51529642094861572, 14.99999999999996447 ) ) ;
#11043=CARTESIAN_POINT ( 'NONE',  ( 104.4587341249999781, 83.12500000136560629, 1.846868145590721655 ) ) ;
#11044=CARTESIAN_POINT ( 'NONE',  ( 78.14518615778179367, 34.74921875108395142, 5.444914386472293977 ) ) ;
#11046=CARTESIAN_POINT ( 'NONE',  ( -13.14518615778179189, 36.63437500108393863, 5.444914386472304635 ) ) ;
#11049=CARTESIAN_POINT ( 'NONE',  ( 130.0000000000000000, 36.03906250000000000, -13.57481594606304576 ) ) ;
#11051=CARTESIAN_POINT ( 'NONE',  ( 143.5748159460630404, 38.96601562499999005, 5.622872871577869525 ) ) ;
#11056=CARTESIAN_POINT ( 'NONE',  ( 135.4449143864723055, 37.62656250108393863, 13.14518615778179189 ) ) ;
#11057=CARTESIAN_POINT ( 'NONE',  ( 59.37712712842213136, 34.89804687716787868, 13.57481594606304753 ) ) ;
#11058=EDGE_CURVE ( 'NONE', #3039, #27020, #25503, .T. ) ;
#11060=CARTESIAN_POINT ( 'NONE',  ( -5.444914386472297529, 40.40468750108393436, -13.14518615778179900 ) ) ;
#11062=AXIS2_PLACEMENT_3D ( 'NONE', #20354, #24200, #20070 ) ;
#11064=ADVANCED_FACE ( 'NONE', ( #5437 ), #18110, .F. ) ;
#11065=CARTESIAN_POINT ( 'NONE',  ( 181.8548138422181921, 35.74140625108393721, -5.444914386472297529 ) ) ;
#11067=EDGE_CURVE ( 'NONE', #12084, #12573, #7412, .T. ) ;
#11069=CARTESIAN_POINT ( 'NONE',  ( -8.312177448680279460E-16, 39.21406249999999716, -13.57481594606304576 ) ) ;
#11076=CARTESIAN_POINT ( 'NONE',  ( 204.5988444088204687, 34.94765624999999432, 9.598844408820456309 ) ) ;
#11077=CARTESIAN_POINT ( 'NONE',  ( 51.42518405393695957, 40.15664062499999432, -5.622872871577872189 ) ) ;
#11079=CARTESIAN_POINT ( 'NONE',  ( 78.14518615778179367, 36.13828125108393863, 5.444914386472293977 ) ) ;
#11085=CARTESIAN_POINT ( 'NONE',  ( 2.493653234604083739E-15, 36.43593749999999432, 13.57481594606304576 ) ) ;
#11086=CARTESIAN_POINT ( 'NONE',  ( 135.4449143864723055, 37.03125000108393294, 13.14518615778179189 ) ) ;
#11089=CARTESIAN_POINT ( 'NONE',  ( 104.9999999999999574, 82.43750000000002842, 2.071067811865462627 ) ) ;
#11090=CARTESIAN_POINT ( 'NONE',  ( 103.5355339059327093, 80.75000000273119838, -3.535533905932755072 ) ) ;
#11094=CARTESIAN_POINT ( 'NONE',  ( 55.40115559117954547, 40.30546874999999574, 9.598844408820459861 ) ) ;
#11099=EDGE_LOOP ( 'NONE', ( #5801, #8695, #3968, #5777, #10257 ) ) ;
#11102=CARTESIAN_POINT ( 'NONE',  ( 181.4251840539369596, 34.00507812716787015, 5.622872871577880183 ) ) ;
#11104=CARTESIAN_POINT ( 'NONE',  ( 51.85481384221820633, 40.65273437608393436, 0.000000000000000000 ) ) ;
#11105=CARTESIAN_POINT ( 'NONE',  ( 135.4449143864723339, 37.82500000108392868, 13.14518615778179189 ) ) ;
#11106=CARTESIAN_POINT ( 'NONE',  ( -9.295050272127046043, 35.89023437608393152, -9.295050272127046043 ) ) ;
#11107=CARTESIAN_POINT ( 'NONE',  ( 135.4449143864723055, 33.95546875108393436, -13.14518615778179900 ) ) ;
#11108=CARTESIAN_POINT ( 'NONE',  ( 59.37712712842213136, 34.00507812499999716, 13.57481594606304753 ) ) ;
#11115=CARTESIAN_POINT ( 'NONE',  ( 101.8468681455907046, 81.00000000136560629, 4.458734124999987891 ) ) ;
#11117=CARTESIAN_POINT ( 'NONE',  ( -5.444914386472297529, 35.04687500108393294, -13.14518615778179900 ) ) ;
#11123=CARTESIAN_POINT ( 'NONE',  ( 200.4449143864723055, 37.92421875108392726, -13.14518615778179900 ) ) ;
#11128=ORIENTED_EDGE ( 'NONE', *, *, #7333, .T. ) ;
#11132=CARTESIAN_POINT ( 'NONE',  ( 135.6228728715778686, 32.11992187716787583, -13.57481594606304753 ) ) ;
#11135=CARTESIAN_POINT ( 'NONE',  ( 65.00000000000000000, 37.37851562608393863, -13.14518615778179544 ) ) ;
#11136=CARTESIAN_POINT ( 'NONE',  ( 73.40231578122690337, 54.99999999485618929, -15.00000000000000000 ) ) ;
#11137=CARTESIAN_POINT ( 'NONE',  ( 189.3771271284221314, 40.85117187499999147, -13.57481594606304753 ) ) ;
#11138=CARTESIAN_POINT ( 'NONE',  ( 70.36494796471481550, 36.00000000000002842, 12.09311862596063136 ) ) ;
#11144=CARTESIAN_POINT ( 'NONE',  ( 96.84719886470459471, 80.31250000136559208, -3.152801135295383084 ) ) ;
#11145=CARTESIAN_POINT ( 'NONE',  ( 204.2950502721270425, 40.25585937608393294, -9.295050272127046043 ) ) ;
#11150=LINE ( 'NONE', #13142, #8642 ) ;
#11153=VERTEX_POINT ( 'NONE', #24951 ) ;
#11156=CIRCLE ( 'NONE', #12963, 13.57481594606304398 ) ;
#11158=CARTESIAN_POINT ( 'NONE',  ( 136.9444263933115167, 31.75150625057403175, -11.16113171639042356 ) ) ;
#11159=CARTESIAN_POINT ( 'NONE',  ( 74.29505027212704249, 33.70742187608393436, 9.295050272127046043 ) ) ;
#11160=CARTESIAN_POINT ( 'NONE',  ( 200.4449143864723055, 36.53515625108393294, -13.14518615778179900 ) ) ;
#11161=VERTEX_POINT ( 'NONE', #15960 ) ;
#11163=CARTESIAN_POINT ( 'NONE',  ( 13.14518615778179900, 33.75703125108393010, 5.444914386472293977 ) ) ;
#11164=CARTESIAN_POINT ( 'NONE',  ( 121.6040612587083416, 54.99999999495823033, -15.00000000000000000 ) ) ;
#11166=CARTESIAN_POINT ( 'NONE',  ( 116.4251840539369596, 40.30546875216787583, 0.000000000000000000 ) ) ;
#11171=EDGE_LOOP ( 'NONE', ( #12932, #15147, #4562, #2491 ) ) ;
#11173=AXIS2_PLACEMENT_3D ( 'NONE', #17806, #6168, #26509 ) ;
#11177=CARTESIAN_POINT ( 'NONE',  ( 126.2834658862103225, 51.46663580899353718, 14.99999999999996270 ) ) ;
#11179=CARTESIAN_POINT ( 'NONE',  ( 130.0000000000000000, 38.51953125216787299, -13.57481594606304576 ) ) ;
#11180=CARTESIAN_POINT ( 'NONE',  ( 98.15313185440925281, 80.87500000136560629, 4.458734124999987891 ) ) ;
#11181=CARTESIAN_POINT ( 'NONE',  ( 55.70494972787295751, 33.70742187608393436, 9.295050272127047819 ) ) ;
#11183=CARTESIAN_POINT ( 'NONE',  ( -13.14518615778179544, 38.96601562608393721, 0.000000000000000000 ) ) ;
#11188=CARTESIAN_POINT ( 'NONE',  ( 116.4251840539369596, 37.82499999999999574, 0.000000000000000000 ) ) ;
#11189=ORIENTED_EDGE ( 'NONE', *, *, #6021, .T. ) ;
#11191=EDGE_CURVE ( 'NONE', #17588, #17231, #12650, .T. ) ;
#11197=CARTESIAN_POINT ( 'NONE',  ( 139.2950502721270425, 35.49335937608393010, -9.295050272127046043 ) ) ;
#11198=CARTESIAN_POINT ( 'NONE',  ( 74.59884440882045453, 33.65781250216787157, -9.598844408820458085 ) ) ;
#11199=ORIENTED_EDGE ( 'NONE', *, *, #246, .T. ) ;
#11201=CARTESIAN_POINT ( 'NONE',  ( 9.598844408820459861, 32.66562500216787157, 9.598844408820456309 ) ) ;
#11202=VECTOR ( 'NONE', #13979, 1000.000000000000000 ) ;
#11206=CARTESIAN_POINT ( 'NONE',  ( 208.1451861577818079, 34.60039062608392868, -1.609821015232357215E-15 ) ) ;
#11216=CARTESIAN_POINT ( 'NONE',  ( 204.5988444088204687, 33.36015624999999574, 9.598844408820456309 ) ) ;
#11220=CARTESIAN_POINT ( 'NONE',  ( 74.29505027212704249, 36.28710937608393294, -9.295050272127046043 ) ) ;
#11224=EDGE_CURVE ( 'NONE', #2100, #21367, #21096, .T. ) ;
#11225=CARTESIAN_POINT ( 'NONE',  ( 195.0000000000000000, 50.00000000000000000, -2.255140518769849538E-14 ) ) ;
#11226=CARTESIAN_POINT ( 'NONE',  ( 9.598844408820456309, 35.93984374999999432, -9.598844408820458085 ) ) ;
#11227=CARTESIAN_POINT ( 'NONE',  ( 116.8548138422182205, 39.16445312608393436, 0.000000000000000000 ) ) ;
#11229=CARTESIAN_POINT ( 'NONE',  ( 94.99999999999995737, 82.93750000000000000, -2.071067811865491048 ) ) ;
#11231=CARTESIAN_POINT ( 'NONE',  ( 102.0710678118654329, 82.43750000273119838, 4.999999999999989342 ) ) ;
#11233=CARTESIAN_POINT ( 'NONE',  ( 130.0000000000000000, 40.80156249999999574, -13.57481594606304576 ) ) ;
#11236=CARTESIAN_POINT ( 'NONE',  ( 65.00000000000000000, 40.40468749999999432, 13.57481594606304576 ) ) ;
#11237=ORIENTED_EDGE ( 'NONE', *, *, #14372, .T. ) ;
#11243=CARTESIAN_POINT ( 'NONE',  ( 195.0000000000000000, 35.74140625216787015, 13.57481594606304576 ) ) ;
#11246=CARTESIAN_POINT ( 'NONE',  ( -13.57481594606304753, 40.95039062499999005, -5.622872871577872189 ) ) ;
#11247=CARTESIAN_POINT ( 'NONE',  ( 124.5550856135277087, 37.42812500108394147, -13.14518615778179722 ) ) ;
#11249=CARTESIAN_POINT ( 'NONE',  ( 9.295050272127046043, 34.10429687608393579, -9.295050272127046043 ) ) ;
#11250=( BOUNDED_CURVE ( )  B_SPLINE_CURVE ( 2, ( #7422, #3305, #11545, #7716, #20262, #24686, #7135, #11976, #13689 ),
 .UNSPECIFIED., .F., .F. ) 
 B_SPLINE_CURVE_WITH_KNOTS ( ( 3, 2, 2, 2, 3 ),
 ( 0.3958333333333331483, 0.4062499999999999445, 0.4166666666666667407, 0.4270833333333335369, 0.4375000000000003331 ),
 .UNSPECIFIED. ) 
 CURVE ( )  GEOMETRIC_REPRESENTATION_ITEM ( )  RATIONAL_B_SPLINE_CURVE ( ( 1.000000000000001110, 0.9238795325112855172, 1.000000000000000000, 0.9238795325112867385, 1.000000000000000000, 0.9238795325112867385, 1.000000000000000000, 0.9238795325112842960, 1.000000000000002442 ) ) 
 REPRESENTATION_ITEM ( '' )  );
#11251=CARTESIAN_POINT ( 'NONE',  ( 116.8548138422182063, 31.87187500108393223, 5.444914386472304635 ) ) ;
#11252=CARTESIAN_POINT ( 'NONE',  ( 51.42518405393695957, 36.23749999999999005, 0.000000000000000000 ) ) ;
#11255=CARTESIAN_POINT ( 'NONE',  ( 99.99999999999995737, 80.87500000273119838, -5.000000000000018652 ) ) ;
#11258=DIRECTION ( 'NONE',  ( 0.000000000000000000, 1.000000000000000000, 0.000000000000000000 ) ) ;
#11261=CARTESIAN_POINT ( 'NONE',  ( 13.14518615778179544, 37.97382812608393721, -1.609821015232357215E-15 ) ) ;
#11264=DIRECTION ( 'NONE',  ( 1.000000000000000000, 0.000000000000000000, -7.228014483236696740E-18 ) ) ;
#11267=EDGE_CURVE ( 'NONE', #23999, #8135, #26594, .T. ) ;
#11268=CARTESIAN_POINT ( 'NONE',  ( 200.4449143864723055, 37.13046875108393152, -13.14518615778179900 ) ) ;
#11269=ORIENTED_EDGE ( 'NONE', *, *, #13761, .T. ) ;
#11272=ORIENTED_EDGE ( 'NONE', *, *, #22909, .T. ) ;
#11276=VECTOR ( 'NONE', #19789, 1000.000000000000000 ) ;
#11277=CARTESIAN_POINT ( 'NONE',  ( 124.5550856135277087, 40.40468750108393436, -13.14518615778179900 ) ) ;
#11278=CARTESIAN_POINT ( 'NONE',  ( 13.14518615778179544, 39.56132812608393579, -1.609821015232357215E-15 ) ) ;
#11280=( BOUNDED_CURVE ( )  B_SPLINE_CURVE ( 2, ( #27983, #327, #4459, #17704, #4178 ),
 .UNSPECIFIED., .F., .T. ) 
 B_SPLINE_CURVE_WITH_KNOTS ( ( 3, 2, 3 ),
 ( 0.4375000000000003331, 0.4479166666666667962, 0.4520580917964571177 ),
 .UNSPECIFIED. ) 
 CURVE ( )  GEOMETRIC_REPRESENTATION_ITEM ( )  RATIONAL_B_SPLINE_CURVE ( ( 0.9999999999999975575, 0.9238795325112891810, 1.000000000000000000, 0.9697362671728813055, 0.9635368512068493985 ) ) 
 REPRESENTATION_ITEM ( '' )  );
#11281=CARTESIAN_POINT ( 'NONE',  ( 51.85481384221819923, 36.73359375108393010, -5.444914386472297529 ) ) ;
#11282=CARTESIAN_POINT ( 'NONE',  ( 64.01693481490168836, 49.99999999948997242, -13.54930971656747474 ) ) ;
#11283=CARTESIAN_POINT ( 'NONE',  ( 200.4449143864723055, 33.06250000108393294, 13.14518615778179189 ) ) ;
#11289=CARTESIAN_POINT ( 'NONE',  ( 70.44491438647229131, 37.62656250108393152, 13.14518615778179189 ) ) ;
#11291=CARTESIAN_POINT ( 'NONE',  ( 195.0000000000000000, 39.56132812608393579, -13.14518615778179544 ) ) ;
#11294=CARTESIAN_POINT ( 'NONE',  ( 189.5550856135277229, 36.63437500108393863, -13.14518615778179722 ) ) ;
#11297=VECTOR ( 'NONE', #7433, 1000.000000000000000 ) ;
#11301=ORIENTED_EDGE ( 'NONE', *, *, #8104, .F. ) ;
#11302=CARTESIAN_POINT ( 'NONE',  ( 139.2950502721270425, 34.10429687608393579, -9.295050272127046043 ) ) ;
#11303=CARTESIAN_POINT ( 'NONE',  ( 78.14518615778179367, 33.01289062608393010, -1.609821015232357215E-15 ) ) ;
#11304=CARTESIAN_POINT ( 'NONE',  ( 181.8548138422182205, 36.78320312608393294, 0.000000000000000000 ) ) ;
#11307=CARTESIAN_POINT ( 'NONE',  ( -5.444914386472299306, 33.55859375108393294, 13.14518615778179722 ) ) ;
#11309=CARTESIAN_POINT ( 'NONE',  ( 135.6228728715778686, 40.05742187716786873, -13.57481594606304753 ) ) ;
#11310=CARTESIAN_POINT ( 'NONE',  ( 65.00000000000000000, 52.00000000000000711, -11.57481594606305109 ) ) ;
#11314=CARTESIAN_POINT ( 'NONE',  ( 73.75489895324048462, 50.00000000000000000, 10.39041163855394068 ) ) ;
#11315=EDGE_LOOP ( 'NONE', ( #24088, #17751, #23216, #23112 ) ) ;
#11317=ORIENTED_EDGE ( 'NONE', *, *, #26747, .T. ) ;
#11321=AXIS2_PLACEMENT_3D ( 'NONE', #21423, #23416, #23141 ) ;
#11323=CARTESIAN_POINT ( 'NONE',  ( 78.57481594606305464, 39.16445312716788152, -5.622872871577873966 ) ) ;
#11324=CARTESIAN_POINT ( 'NONE',  ( 70.44491438647230552, 35.74140625108393721, -13.14518615778179900 ) ) ;
#11327=CARTESIAN_POINT ( 'NONE',  ( 13.14518615778179544, 37.77539062608393294, -1.609821015232357215E-15 ) ) ;
#11329=CARTESIAN_POINT ( 'NONE',  ( 6.873508243573242638, 51.14166184781125679, 15.00000000000065548 ) ) ;
#11331=CARTESIAN_POINT ( 'NONE',  ( 124.3771271284221314, 36.88242187499999858, -13.57481594606304753 ) ) ;
#11332=ORIENTED_EDGE ( 'NONE', *, *, #14922, .F. ) ;
#11333=ORIENTED_EDGE ( 'NONE', *, *, #13179, .T. ) ;
#11334=PLANE ( 'NONE',  #7189 ) ;
#11338=CARTESIAN_POINT ( 'NONE',  ( 130.0000000000000000, 34.00507812608393721, -13.14518615778179544 ) ) ;
#11339=CARTESIAN_POINT ( 'NONE',  ( 65.00000000000000000, 35.34453125216787583, -13.57481594606304576 ) ) ;
#11341=CARTESIAN_POINT ( 'NONE',  ( -13.57481594606304576, 31.62382812716787228, 5.622872871577880183 ) ) ;
#11344=DIRECTION ( 'NONE',  ( -1.156482317317871478E-16, 0.000000000000000000, -1.000000000000000000 ) ) ;
#11346=CARTESIAN_POINT ( 'NONE',  ( 208.1451861577817795, 32.96328125108393436, 5.444914386472293977 ) ) ;
#11348=CARTESIAN_POINT ( 'NONE',  ( 99.99999999999995737, 85.00000000000000000, -1.387778780781445676E-14 ) ) ;
#11357=CARTESIAN_POINT ( 'NONE',  ( 185.4011555911795597, 35.54296874999999289, 9.598844408820459861 ) ) ;
#11360=DIRECTION ( 'NONE',  ( -0.000000000000000000, -1.000000000000000000, -0.000000000000000000 ) ) ;
#11361=CARTESIAN_POINT ( 'NONE',  ( 78.14518615778179367, 37.03125000108393294, -5.444914386472297529 ) ) ;
#11364=( BOUNDED_CURVE ( )  B_SPLINE_CURVE ( 2, ( #10671, #11870, #14948, #9882, #25939, #3199, #12522, #19104, #18590 ),
 .UNSPECIFIED., .F., .T. ) 
 B_SPLINE_CURVE_WITH_KNOTS ( ( 3, 2, 2, 2, 3 ),
 ( 0.2708333333333330928, 0.2812499999999998890, 0.2916666666666666852, 0.3020833333333334259, 0.3125000000000002220 ),
 .UNSPECIFIED. ) 
 CURVE ( )  GEOMETRIC_REPRESENTATION_ITEM ( )  RATIONAL_B_SPLINE_CURVE ( ( 1.000000000000001554, 0.9238795325112850731, 1.000000000000000000, 0.9238795325112867385, 1.000000000000000000, 0.9238795325112867385, 1.000000000000000000, 0.9238795325112850731, 1.000000000000001554 ) ) 
 REPRESENTATION_ITEM ( '' )  );
#11367=CARTESIAN_POINT ( 'NONE',  ( 5.622872871577871301, 35.98945312499999716, -13.57481594606304753 ) ) ;
#11368=CARTESIAN_POINT ( 'NONE',  ( 135.4449143864723055, 37.82500000108392868, 13.14518615778179189 ) ) ;
#11370=CARTESIAN_POINT ( 'NONE',  ( 96.46446609406721961, 80.12500000000000000, 3.535533905932727539 ) ) ;
#11372=CARTESIAN_POINT ( 'NONE',  ( 99.99999999999995737, 85.00000000000000000, -1.387778780781445676E-14 ) ) ;
#11373=CARTESIAN_POINT ( 'NONE',  ( 94.99999999999995737, 82.12500000273119838, -1.387778780781445676E-14 ) ) ;
#11375=CARTESIAN_POINT ( 'NONE',  ( 56.33088789466297186, 36.00000000000002842, -10.16963847934322906 ) ) ;
#11379=CARTESIAN_POINT ( 'NONE',  ( 70.44491438647230552, 33.06250000108393294, 13.14518615778179189 ) ) ;
#11380=ORIENTED_EDGE ( 'NONE', *, *, #8087, .F. ) ;
#11383=ORIENTED_EDGE ( 'NONE', *, *, #23409, .T. ) ;
#11385=CARTESIAN_POINT ( 'NONE',  ( 208.5748159460630688, 35.14609375216787157, -1.662435489736055892E-15 ) ) ;
#11389=DIRECTION ( 'NONE',  ( -0.000000000000000000, 1.000000000000000000, -0.000000000000000000 ) ) ;
#11391=CARTESIAN_POINT ( 'NONE',  ( -5.444914386472299306, 33.75703125108393721, 13.14518615778179722 ) ) ;
#11393=ADVANCED_FACE ( 'NONE', ( #19087 ), #27795, .T. ) ;
#11395=CARTESIAN_POINT ( 'NONE',  ( 59.37712712842213136, 34.79882812499998579, 13.57481594606304753 ) ) ;
#11404=CARTESIAN_POINT ( 'NONE',  ( 13.14518615778179900, 37.22968750108393721, -5.444914386472297529 ) ) ;
#11406=ORIENTED_EDGE ( 'NONE', *, *, #17196, .F. ) ;
#11409=VECTOR ( 'NONE', #26779, 1000.000000000000000 ) ;
#11410=CARTESIAN_POINT ( 'NONE',  ( 204.2950502721270425, 34.50117187608393010, 9.295050272127046043 ) ) ;
#11412=CARTESIAN_POINT ( 'NONE',  ( 203.7583343923459154, 50.00000000000000000, -10.38725784494393345 ) ) ;
#11419=CARTESIAN_POINT ( 'NONE',  ( 130.0000000000000000, 39.95820312608393010, 13.14518615778179544 ) ) ;
#11421=CARTESIAN_POINT ( 'NONE',  ( -9.295050272127046043, 35.69179687608393436, -9.295050272127046043 ) ) ;
#11424=CARTESIAN_POINT ( 'NONE',  ( 78.14518615778179367, 38.76757812608393294, -1.609821015232357215E-15 ) ) ;
#11425=CARTESIAN_POINT ( 'NONE',  ( 72.11549039185503318, 49.99999999945668350, -11.58166858714116998 ) ) ;
#11427=EDGE_CURVE ( 'NONE', #23060, #5791, #15442, .T. ) ;
#11428=CARTESIAN_POINT ( 'NONE',  ( 201.9444236247691720, 31.75150628229955529, -11.16113343896966370 ) ) ;
#11429=CARTESIAN_POINT ( 'NONE',  ( 77.07727640983618755, 35.99999999999999289, -6.197985357348143154 ) ) ;
#11432=CARTESIAN_POINT ( 'NONE',  ( 66.13716782454086740, 35.99999999999998579, 13.09590655363602707 ) ) ;
#11433=CARTESIAN_POINT ( 'NONE',  ( 55.40115559117954547, 38.71796874999999716, 9.598844408820459861 ) ) ;
#11434=CARTESIAN_POINT ( 'NONE',  ( 200.4449143864723055, 36.83281250108392868, 13.14518615778179189 ) ) ;
#11438=CARTESIAN_POINT ( 'NONE',  ( 204.2950502721270425, 36.48554687608393721, -9.295050272127046043 ) ) ;
#11440=ORIENTED_EDGE ( 'NONE', *, *, #8464, .T. ) ;
#11443=ORIENTED_EDGE ( 'NONE', *, *, #6166, .F. ) ;
#11444=CARTESIAN_POINT ( 'NONE',  ( 135.4449143864723055, 34.15390625108393863, -13.14518615778179900 ) ) ;
#11446=CARTESIAN_POINT ( 'NONE',  ( 181.8548138422182205, 35.19570312608393436, 0.000000000000000000 ) ) ;
#11447=ORIENTED_EDGE ( 'NONE', *, *, #19485, .T. ) ;
#11449=CARTESIAN_POINT ( 'NONE',  ( 4.062583540575953833, 50.00000000116115473, -12.98908657125259580 ) ) ;
#11451=( BOUNDED_CURVE ( )  B_SPLINE_CURVE ( 2, ( #633, #11859, #11433, #5332, #1064, #7162, #17866, #4909, #20581 ),
 .UNSPECIFIED., .F., .F. ) 
 B_SPLINE_CURVE_WITH_KNOTS ( ( 3, 2, 2, 2, 3 ),
 ( 0.2291666666666665741, 0.2395833333333332316, 0.2499999999999998335, 0.2604166666666665186, 0.2708333333333330928 ),
 .UNSPECIFIED. ) 
 CURVE ( )  GEOMETRIC_REPRESENTATION_ITEM ( )  RATIONAL_B_SPLINE_CURVE ( ( 1.000000000000000666, 0.9238795325112861834, 1.000000000000000000, 0.9238795325112867385, 1.000000000000000000, 0.9238795325112867385, 1.000000000000000000, 0.9238795325112884038, 0.9999999999999983347 ) ) 
 REPRESENTATION_ITEM ( '' )  );
#11452=CARTESIAN_POINT ( 'NONE',  ( 78.57481594606305464, 40.60312499999999858, -1.662435489736055892E-15 ) ) ;
#11454=LINE ( 'NONE', #801, #6083 ) ;
#11456=CARTESIAN_POINT ( 'NONE',  ( 72.62196353419399486, 54.91641323977498246, 14.99999999999997868 ) ) ;
#11463=CARTESIAN_POINT ( 'NONE',  ( 138.2596115288800434, 50.00000000056351723, 10.79618466886582340 ) ) ;
#11465=CARTESIAN_POINT ( 'NONE',  ( -13.05838185645087357, 36.00000000000000000, 1.569311539113920739 ) ) ;
#11466=FACE_OUTER_BOUND ( 'NONE', #6109, .T. ) ;
#11469=CARTESIAN_POINT ( 'NONE',  ( -13.14518615778179722, 36.53515625108393294, -5.444914386472297529 ) ) ;
#11470=DIRECTION ( 'NONE',  ( -0.000000000000000000, 1.000000000000000000, -0.000000000000000000 ) ) ;
#11471=CARTESIAN_POINT ( 'NONE',  ( -9.180175813647995398, 55.00000000000000711, 14.99999999999999822 ) ) ;
#11473=CARTESIAN_POINT ( 'NONE',  ( 130.0000000000000000, 36.03906250000000000, -13.57481594606304576 ) ) ;
#11476=ORIENTED_EDGE ( 'NONE', *, *, #4634, .T. ) ;
#11481=CARTESIAN_POINT ( 'NONE',  ( 116.8548138422182205, 32.61601562608393579, 0.000000000000000000 ) ) ;
#11482=CARTESIAN_POINT ( 'NONE',  ( 74.29505027212704249, 39.26367187608393294, 9.295050272127046043 ) ) ;
#11483=CARTESIAN_POINT ( 'NONE',  ( 103.5355339059327093, 80.62500000000000000, -3.535533905932755072 ) ) ;
#11484=CARTESIAN_POINT ( 'NONE',  ( 9.598844408820456309, 32.07031250216787299, -9.598844408820458085 ) ) ;
#11485=DIRECTION ( 'NONE',  ( -1.000000000000000000, 0.000000000000000000, 3.469446951953615175E-16 ) ) ;
#11488=CARTESIAN_POINT ( 'NONE',  ( 208.1451861577817795, 35.44375000108393436, -5.444914386472297529 ) ) ;
#11497=CARTESIAN_POINT ( 'NONE',  ( -7.228014483236695816E-17, 80.00000000000000000, -9.999999999999998224 ) ) ;
#11500=CARTESIAN_POINT ( 'NONE',  ( 208.5748159460630120, 32.71523437500000142, -5.622872871577873077 ) ) ;
#11502=DIRECTION ( 'NONE',  ( 0.000000000000000000, 0.000000000000000000, -1.000000000000000000 ) ) ;
#11503=CARTESIAN_POINT ( 'NONE',  ( 104.4587341249999781, 82.00000000136560629, -1.846868145590750299 ) ) ;
#11504=CARTESIAN_POINT ( 'NONE',  ( 78.14518615778179367, 36.23750000108393010, -5.444914386472297529 ) ) ;
#11507=CARTESIAN_POINT ( 'NONE',  ( 13.57481594606304931, 37.37851562499999858, 5.622872871577868636 ) ) ;
#11508=CARTESIAN_POINT ( 'NONE',  ( -9.598844408820454532, 33.16171874999999858, 9.598844408820459861 ) ) ;
#11509=CARTESIAN_POINT ( 'NONE',  ( 116.8548138422182205, 36.78320312608393294, 0.000000000000000000 ) ) ;
#11512=EDGE_CURVE ( 'NONE', #26308, #3039, #20500, .T. ) ;
#11514=CARTESIAN_POINT ( 'NONE',  ( 101.8468681455906903, 83.12500000136560629, -4.458734125000016313 ) ) ;
#11518=CARTESIAN_POINT ( 'NONE',  ( 65.00000000000000000, 31.82226562608393650, -13.14518615778179544 ) ) ;
#11522=ORIENTED_EDGE ( 'NONE', *, *, #21171, .T. ) ;
#11524=CARTESIAN_POINT ( 'NONE',  ( 185.4011555911795313, 33.85625000216787583, -9.598844408820458085 ) ) ;
#11525=ORIENTED_EDGE ( 'NONE', *, *, #1184, .F. ) ;
#11529=CARTESIAN_POINT ( 'NONE',  ( -5.444914386472297529, 35.04687500108393294, -13.14518615778179900 ) ) ;
#11530=CARTESIAN_POINT ( 'NONE',  ( 143.1451861577818079, 32.21914062608393436, -1.609821015232357215E-15 ) ) ;
#11534=CARTESIAN_POINT ( 'NONE',  ( 65.00000000000000000, 36.93203125216787441, -13.57481594606304576 ) ) ;
#11537=LINE ( 'NONE', #20252, #6235 ) ;
#11541=CARTESIAN_POINT ( 'NONE',  ( 103.5355339059327093, 83.50000000273119838, 3.535533905932726206 ) ) ;
#11542=DIRECTION ( 'NONE',  ( 1.000000000000000000, -0.000000000000000000, -7.228014483236696740E-18 ) ) ;
#11543=CARTESIAN_POINT ( 'NONE',  ( 2.414731522848535132E-15, 33.80664062608393294, 13.14518615778179544 ) ) ;
#11545=CARTESIAN_POINT ( 'NONE',  ( 120.4011555911795455, 37.13046874999999147, 9.598844408820459861 ) ) ;
#11546=CARTESIAN_POINT ( 'NONE',  ( -13.57481594606304576, 37.82499999999999574, 0.000000000000000000 ) ) ;
#11549=ADVANCED_FACE ( 'NONE', ( #2232 ), #17178, .T. ) ;
#11550=CARTESIAN_POINT ( 'NONE',  ( 189.5550856135277229, 34.35234375108392868, 13.14518615778179722 ) ) ;
#11551=ORIENTED_EDGE ( 'NONE', *, *, #18399, .T. ) ;
#11557=CYLINDRICAL_SURFACE ( 'NONE', #20837, 5.000000000000000888 ) ;
#11558=EDGE_CURVE ( 'NONE', #12573, #15363, #2944, .T. ) ;
#11559=CARTESIAN_POINT ( 'NONE',  ( 116.8548138422182205, 38.96601562608393721, 0.000000000000000000 ) ) ;
#11560=CARTESIAN_POINT ( 'NONE',  ( 9.295050272127046043, 36.48554687608393721, -9.295050272127046043 ) ) ;
#11561=CARTESIAN_POINT ( 'NONE',  ( 5.444914386472302859, 34.45156250108393436, 13.14518615778179189 ) ) ;
#11563=CARTESIAN_POINT ( 'NONE',  ( 58.88015637230197541, 51.28708186914660416, -14.99999999999791100 ) ) ;
#11565=CARTESIAN_POINT ( 'NONE',  ( 189.3771271284221314, 40.05742187499999574, -13.57481594606304753 ) ) ;
#11567=CARTESIAN_POINT ( 'NONE',  ( 68.82956275799186585, 36.00000000000000711, 12.63428651647593703 ) ) ;
#11568=VERTEX_POINT ( 'NONE', #2374 ) ;
#11571=CARTESIAN_POINT ( 'NONE',  ( 78.14518615778180788, 38.61875000108392442, -5.444914386472297529 ) ) ;
#11573=CARTESIAN_POINT ( 'NONE',  ( 181.8548138422182205, 36.53515625108393294, -5.444914386472297529 ) ) ;
#11577=CARTESIAN_POINT ( 'NONE',  ( 185.7049497278729575, 37.67617187608393436, 9.295050272127047819 ) ) ;
#11579=ORIENTED_EDGE ( 'NONE', *, *, #23099, .T. ) ;
#11580=CIRCLE ( 'NONE', #27110, 11.57481594606304398 ) ;
#11583=VERTEX_POINT ( 'NONE', #22173 ) ;
#11584=CARTESIAN_POINT ( 'NONE',  ( 130.0000000000000000, 32.61601562608393579, -13.14518615778179544 ) ) ;
#11585=CARTESIAN_POINT ( 'NONE',  ( 65.00000000000000000, 36.83281249999999574, -13.57481594606304576 ) ) ;
#11587=CARTESIAN_POINT ( 'NONE',  ( 200.4449143864723055, 32.56640625108394005, -13.14518615778179900 ) ) ;
#11588=EDGE_LOOP ( 'NONE', ( #6863, #27028, #872, #70 ) ) ;
#11592=CARTESIAN_POINT ( 'NONE',  ( 143.5748159460630404, 36.78320312716786589, -5.622872871577873077 ) ) ;
#11596=CARTESIAN_POINT ( 'NONE',  ( 69.50488708631583279, 51.44650206077173493, 15.00000000000263611 ) ) ;
#11601=CARTESIAN_POINT ( 'NONE',  ( 134.8584992904650051, 49.99999999891522151, 12.70434618648776137 ) ) ;
#11604=CARTESIAN_POINT ( 'NONE',  ( 51.85481384221820633, 32.07031250108393294, 5.444914386472304635 ) ) ;
#11605=CARTESIAN_POINT ( 'NONE',  ( -8.312177448680279460E-16, 40.10703125216787157, -13.57481594606304576 ) ) ;
#11607=CARTESIAN_POINT ( 'NONE',  ( 9.295050272127047819, 36.88242187608393152, 9.295050272127046043 ) ) ;
#11610=CARTESIAN_POINT ( 'NONE',  ( 2.529583995170619826, 49.99999999938378892, 13.34625891065936543 ) ) ;
#11612=CARTESIAN_POINT ( 'NONE',  ( 143.5748159460630404, 33.50898437499999716, -5.622872871577873077 ) ) ;
#11613=ORIENTED_EDGE ( 'NONE', *, *, #368, .F. ) ;
#11614=FACE_OUTER_BOUND ( 'NONE', #10758, .T. ) ;
#11619=CARTESIAN_POINT ( 'NONE',  ( 135.4449143864723055, 34.45156250108393436, 13.14518615778179189 ) ) ;
#11620=CARTESIAN_POINT ( 'NONE',  ( 59.55508561352770158, 40.40468750108393436, -13.14518615778179900 ) ) ;
#11623=FACE_OUTER_BOUND ( 'NONE', #25191, .T. ) ;
#11624=CARTESIAN_POINT ( 'NONE',  ( -13.14518615778179900, 39.71015625108393010, -5.444914386472297529 ) ) ;
#11629=CARTESIAN_POINT ( 'NONE',  ( 181.8548138422182205, 32.61601562608393579, 0.000000000000000000 ) ) ;
#11630=AXIS2_PLACEMENT_3D ( 'NONE', #11372, #13363, #17945 ) ;
#11631=CYLINDRICAL_SURFACE ( 'NONE', #26579, 13.57481594606304398 ) ;
#11635=CARTESIAN_POINT ( 'NONE',  ( 124.3771271284221740, 36.48554687716787726, 13.57481594606311504 ) ) ;
#11636=CARTESIAN_POINT ( 'NONE',  ( 99.99999999999995737, 85.00000000000000000, -1.387778780781445676E-14 ) ) ;
#11643=CARTESIAN_POINT ( 'NONE',  ( 5.622872871578008080, 36.78320312499999289, -13.57481594606290898 ) ) ;
#11645=CARTESIAN_POINT ( 'NONE',  ( 70.44491438647230552, 33.65781250108393152, 13.14518615778179189 ) ) ;
#11651=CARTESIAN_POINT ( 'NONE',  ( 214.9999999999999716, 75.00000000000000000, -10.00000000000000000 ) ) ;
#11652=CARTESIAN_POINT ( 'NONE',  ( 135.4449143864723055, 35.44375000108393436, 13.14518615778179189 ) ) ;
#11654=CARTESIAN_POINT ( 'NONE',  ( 99.99999999999995737, 81.25000000000000000, 4.999999999999990230 ) ) ;
#11656=CARTESIAN_POINT ( 'NONE',  ( 101.8468681455906903, 82.75000000136560629, 4.458734124999987891 ) ) ;
#11659=CARTESIAN_POINT ( 'NONE',  ( 204.5988444088204687, 37.32890624999999574, 9.598844408820456309 ) ) ;
#11661=CARTESIAN_POINT ( 'NONE',  ( 65.00000000000000000, 40.00781250000000000, -13.57481594606304576 ) ) ;
#11662=CARTESIAN_POINT ( 'NONE',  ( -9.598844408820454532, 38.02343750216788010, 9.598844408820459861 ) ) ;
#11663=VERTEX_POINT ( 'NONE', #26739 ) ;
#11669=CARTESIAN_POINT ( 'NONE',  ( 185.4011555911795597, 31.67343750216787512, 9.598844408820459861 ) ) ;
#11672=CARTESIAN_POINT ( 'NONE',  ( 195.0000000000000000, 36.13828125216787157, -13.57481594606304576 ) ) ;
#11673=CARTESIAN_POINT ( 'NONE',  ( 116.8548138422182205, 40.50390625108394005, -5.444914386472297529 ) ) ;
#11674=CARTESIAN_POINT ( 'NONE',  ( -9.295050272127044266, 35.29492187608393294, 9.295050272127047819 ) ) ;
#11676=CARTESIAN_POINT ( 'NONE',  ( 120.7049497278729575, 31.92148437608393508, 9.295050272127047819 ) ) ;
#11678=CARTESIAN_POINT ( 'NONE',  ( 124.4309414480975136, 36.00000000000002842, 11.91493531101283843 ) ) ;
#11680=CARTESIAN_POINT ( 'NONE',  ( -13.57481594606304753, 37.87460937716787868, -5.622872871577872189 ) ) ;
#11683=CYLINDRICAL_SURFACE ( 'NONE', #23016, 13.57481594606304398 ) ;
#11685=CARTESIAN_POINT ( 'NONE',  ( 13.14518615778179544, 33.21132812608393436, -1.609821015232357215E-15 ) ) ;
#11690=CARTESIAN_POINT ( 'NONE',  ( -13.57481594606304398, 36.28710937499999289, 5.622872871577880183 ) ) ;
#11691=CARTESIAN_POINT ( 'NONE',  ( 204.2950502721270425, 36.08867187608392868, 9.295050272127046043 ) ) ;
#11695=ORIENTED_EDGE ( 'NONE', *, *, #22026, .F. ) ;
#11698=CARTESIAN_POINT ( 'NONE',  ( 65.00000000000000000, 40.10703125216787157, -13.57481594606304576 ) ) ;
#11700=CARTESIAN_POINT ( 'NONE',  ( 130.0000000000000000, -7.395377635281828788, -13.57481594606305997 ) ) ;
#11701=CARTESIAN_POINT ( 'NONE',  ( 124.5550856135277087, 38.81718750108393579, -13.14518615778179900 ) ) ;
#11702=CARTESIAN_POINT ( 'NONE',  ( -9.295050272127046043, 37.47773437608393010, -9.295050272127046043 ) ) ;
#11703=CARTESIAN_POINT ( 'NONE',  ( 9.295050272127046043, 35.49335937608393010, -9.295050272127046043 ) ) ;
#11705=VECTOR ( 'NONE', #10186, 1000.000000000000000 ) ;
#11706=VECTOR ( 'NONE', #25806, 1000.000000000000000 ) ;
#11707=CARTESIAN_POINT ( 'NONE',  ( 63.18564464541649528, 51.46618445021698562, -14.99999999999862865 ) ) ;
#11713=CARTESIAN_POINT ( 'NONE',  ( 78.14518615778180788, 37.82500000108392868, -5.444914386472297529 ) ) ;
#11720=CARTESIAN_POINT ( 'NONE',  ( 204.2950502721270425, 38.66835937608393436, 9.295050272127046043 ) ) ;
#11722=ORIENTED_EDGE ( 'NONE', *, *, #17150, .F. ) ;
#11726=CARTESIAN_POINT ( 'NONE',  ( 120.7049497278729575, 33.70742187608393436, 9.295050272127047819 ) ) ;
#11727=CARTESIAN_POINT ( 'NONE',  ( 181.4251840539369596, 37.13046875216787868, 0.000000000000000000 ) ) ;
#11728=CARTESIAN_POINT ( 'NONE',  ( 195.0000000000000000, 33.40976562608393863, -13.14518615778179544 ) ) ;
#11734=CARTESIAN_POINT ( 'NONE',  ( 120.4011555911795455, 36.23750000216787726, -9.598844408820458085 ) ) ;
#11739=CARTESIAN_POINT ( 'NONE',  ( 67.27614684454866278, 51.46995505939283078, 14.99999999999998046 ) ) ;
#11745=CARTESIAN_POINT ( 'NONE',  ( -9.839381608887936892, 36.00000000000000711, -9.004033604613056241 ) ) ;
#11749=AXIS2_PLACEMENT_3D ( 'NONE', #21765, #8779, #8502 ) ;
#11750=DIRECTION ( 'NONE',  ( -0.000000000000000000, 1.000000000000000000, -0.000000000000000000 ) ) ;
#11751=CARTESIAN_POINT ( 'NONE',  ( 55.70494972787295751, 32.71523437608393436, -9.295050272127046043 ) ) ;
#11754=CARTESIAN_POINT ( 'NONE',  ( 13.14518615778179544, 36.18789062608393436, -1.609821015232357215E-15 ) ) ;
#11756=CARTESIAN_POINT ( 'NONE',  ( -7.115490391851705176, 49.99999999945661244, 11.58166858714319147 ) ) ;
#11757=CARTESIAN_POINT ( 'NONE',  ( 65.00000000000000000, 40.80156249999999574, -13.57481594606304576 ) ) ;
#11758=CARTESIAN_POINT ( 'NONE',  ( 120.4011555911795455, 32.96328124999999432, -9.598844408820458085 ) ) ;
#11761=FACE_OUTER_BOUND ( 'NONE', #25941, .T. ) ;
#11765=CARTESIAN_POINT ( 'NONE',  ( 143.1451861577818079, 33.85625000108393579, -5.444914386472297529 ) ) ;
#11766=CARTESIAN_POINT ( 'NONE',  ( 59.37712712842213136, 31.42539062716787157, -13.57481594606304753 ) ) ;
#11767=CARTESIAN_POINT ( 'NONE',  ( 103.5355339059327093, 80.37500000000000000, 3.535533905932726206 ) ) ;
#11768=CARTESIAN_POINT ( 'NONE',  ( 5.444914386472297529, 40.30546875108393579, -13.14518615778179900 ) ) ;
#11770=CARTESIAN_POINT ( 'NONE',  ( 182.0005117698094352, 35.99999999999999289, 1.999176114741937349 ) ) ;
#11771=CARTESIAN_POINT ( 'NONE',  ( 95.54126587499996504, 84.68750000136560629, -1.387778780781445676E-14 ) ) ;
#11774=CARTESIAN_POINT ( 'NONE',  ( 200.4449143864723055, 32.36796875108393579, -13.14518615778179900 ) ) ;
#11775=DIRECTION ( 'NONE',  ( 0.000000000000000000, 1.000000000000000000, 0.000000000000000000 ) ) ;
#11779=CARTESIAN_POINT ( 'NONE',  ( 121.3308878946625384, 36.00000000000000711, -10.16963847934280096 ) ) ;
#11783=DIRECTION ( 'NONE',  ( -0.000000000000000000, 1.000000000000000000, -0.000000000000000000 ) ) ;
#11790=CARTESIAN_POINT ( 'NONE',  ( 55.70494972787295751, 40.05742187608393579, 9.295050272127047819 ) ) ;
#11794=CARTESIAN_POINT ( 'NONE',  ( 130.0000000000000000, 36.00000000000000000, 11.57481594606302799 ) ) ;
#11795=CARTESIAN_POINT ( 'NONE',  ( 5.622872871577871301, 33.60820312499998863, -13.57481594606304753 ) ) ;
#11797=CARTESIAN_POINT ( 'NONE',  ( 143.1451861577818079, 33.21132812608393436, -1.609821015232357215E-15 ) ) ;
#11802=CARTESIAN_POINT ( 'NONE',  ( 103.5355339059327093, 79.50000000273119838, 3.535533905932726206 ) ) ;
#11804=AXIS2_PLACEMENT_3D ( 'NONE', #23556, #21002, #27698 ) ;
#11805=CARTESIAN_POINT ( 'NONE',  ( 51.42518405393695957, 38.76757812716787299, 5.622872871577880183 ) ) ;
#11807=CARTESIAN_POINT ( 'NONE',  ( 181.8548138422181921, 32.56640625108394005, -5.444914386472297529 ) ) ;
#11808=CARTESIAN_POINT ( 'NONE',  ( -5.622872871577873077, 40.15664062716787441, -13.57481594606304753 ) ) ;
#11810=CARTESIAN_POINT ( 'NONE',  ( 182.4334932752013287, 36.00000000000000000, -4.295155080288603600 ) ) ;
#11815=CARTESIAN_POINT ( 'NONE',  ( 208.5748159460630120, 31.92148437716787512, 5.622872871577869525 ) ) ;
#11819=CARTESIAN_POINT ( 'NONE',  ( -13.14518615778179544, 32.02070312608393010, 0.000000000000000000 ) ) ;
#11820=CARTESIAN_POINT ( 'NONE',  ( 120.7049497278729575, 32.71523437608393436, 9.295050272127047819 ) ) ;
#11826=CARTESIAN_POINT ( 'NONE',  ( 51.85481384221820633, 40.55351562608393579, 0.000000000000000000 ) ) ;
#11830=CARTESIAN_POINT ( 'NONE',  ( 181.4251840539369596, 40.30546875216787583, 0.000000000000000000 ) ) ;
#11832=CARTESIAN_POINT ( 'NONE',  ( 13.14518615778179900, 34.05468750108394005, -5.444914386472297529 ) ) ;
#11838=CARTESIAN_POINT ( 'NONE',  ( 200.4449143864723055, 35.24531250108393010, 13.14518615778179189 ) ) ;
#11840=CARTESIAN_POINT ( 'NONE',  ( 194.2761280619777153, 53.51529642094860861, -15.00000000000000000 ) ) ;
#11848=CARTESIAN_POINT ( 'NONE',  ( 130.0000000000000000, 37.18007812608393436, -13.14518615778179544 ) ) ;
#11849=CARTESIAN_POINT ( 'NONE',  ( 13.14518615778179722, 38.71796875108393721, 5.444914386472293977 ) ) ;
#11850=CARTESIAN_POINT ( 'NONE',  ( -5.444914386472297529, 35.64218750108392442, -13.14518615778179900 ) ) ;
#11854=DIRECTION ( 'NONE',  ( 0.000000000000000000, 0.000000000000000000, -1.000000000000000000 ) ) ;
#11857=CARTESIAN_POINT ( 'NONE',  ( 55.70494972787295751, 36.48554687608393721, -9.295050272127046043 ) ) ;
#11858=DIRECTION ( 'NONE',  ( 1.000000000000000000, 0.000000000000000000, 0.000000000000000000 ) ) ;
#11859=CARTESIAN_POINT ( 'NONE',  ( 59.37712712842216689, 38.76757812499998579, 13.57481594606308128 ) ) ;
#11860=CARTESIAN_POINT ( 'NONE',  ( 208.1451861577818079, 36.13828125108393152, 5.444914386472293977 ) ) ;
#11864=CARTESIAN_POINT ( 'NONE',  ( 204.2950502721270425, 38.07304687608393579, -9.295050272127046043 ) ) ;
#11866=EDGE_CURVE ( 'NONE', #27029, #3371, #14591, .T. ) ;
#11869=ORIENTED_EDGE ( 'NONE', *, *, #25266, .T. ) ;
#11870=CARTESIAN_POINT ( 'NONE',  ( 200.6228728715777834, 37.67617187716787441, -13.57481594606313990 ) ) ;
#11871=CARTESIAN_POINT ( 'NONE',  ( 55.70494972787295751, 39.85898437608393152, -9.295050272127046043 ) ) ;
#11872=CARTESIAN_POINT ( 'NONE',  ( 185.7049497278729575, 33.70742187608393436, 9.295050272127047819 ) ) ;
#11873=VERTEX_POINT ( 'NONE', #6052 ) ;
#11877=CARTESIAN_POINT ( 'NONE',  ( 120.4011555911795455, 38.81718750216787583, 9.598844408820459861 ) ) ;
#11878=DIRECTION ( 'NONE',  ( 0.000000000000000000, -1.000000000000000000, -0.000000000000000000 ) ) ;
#11880=CARTESIAN_POINT ( 'NONE',  ( 185.7049497278729575, 40.65273437608393436, -9.295050272127046043 ) ) ;
#11881=ORIENTED_EDGE ( 'NONE', *, *, #8674, .T. ) ;
#11887=CARTESIAN_POINT ( 'NONE',  ( -8.125303917791546482, 36.00000000000000711, 10.34220695173551263 ) ) ;
#11888=CARTESIAN_POINT ( 'NONE',  ( 78.57481594606305464, 37.47773437716787015, 5.622872871577868636 ) ) ;
#11889=CARTESIAN_POINT ( 'NONE',  ( -18.00000000000000711, 78.00000000000000000, 2.081668171172169302E-15 ) ) ;
#11893=CARTESIAN_POINT ( 'NONE',  ( 219.9999999999999716, 50.00000000000000000, -10.00000000000000000 ) ) ;
#11894=CARTESIAN_POINT ( 'NONE',  ( 6.412866676253258014, 50.00000000108448006, 11.99502265407631185 ) ) ;
#11895=CARTESIAN_POINT ( 'NONE',  ( 139.5988444088204403, 40.70234374999999716, -9.598844408820458085 ) ) ;
#11896=CARTESIAN_POINT ( 'NONE',  ( 139.5988444088204403, 32.76484374999999716, -9.598844408820458085 ) ) ;
#11903=CARTESIAN_POINT ( 'NONE',  ( 124.5550856135277087, 31.97109375108393436, 13.14518615778179722 ) ) ;
#11905=CARTESIAN_POINT ( 'NONE',  ( 65.00000000000000000, 32.16953125216787157, -13.57481594606304576 ) ) ;
#11907=CARTESIAN_POINT ( 'NONE',  ( 13.57481594606304753, 37.57695312716787583, -5.622872871577873966 ) ) ;
#11908=CARTESIAN_POINT ( 'NONE',  ( 13.14518615778179900, 37.82500000108392868, -5.444914386472297529 ) ) ;
#11911=CARTESIAN_POINT ( 'NONE',  ( 182.2616098421445656, 36.00000000000000000, 3.273369733618571420 ) ) ;
#11913=VERTEX_POINT ( 'NONE', #3909 ) ;
#11915=CARTESIAN_POINT ( 'NONE',  ( 185.7049497278729575, 31.72304687608393081, -9.295050272127046043 ) ) ;
#11918=EDGE_CURVE ( 'NONE', #444, #10301, #7900, .T. ) ;
#11920=CARTESIAN_POINT ( 'NONE',  ( 185.4011555911795597, 39.51171874999999289, 9.598844408820459861 ) ) ;
#11929=CARTESIAN_POINT ( 'NONE',  ( 195.0000000000000000, 36.03906250000000000, -13.57481594606304576 ) ) ;
#11931=CARTESIAN_POINT ( 'NONE',  ( 78.14518615778179367, 33.01289062608393010, -1.609821015232357215E-15 ) ) ;
#11935=CARTESIAN_POINT ( 'NONE',  ( 9.598844408820456309, 37.52734375000000000, -9.598844408820458085 ) ) ;
#11936=CARTESIAN_POINT ( 'NONE',  ( -13.57481594606304753, 33.01289062500000426, -5.622872871577873077 ) ) ;
#11938=CARTESIAN_POINT ( 'NONE',  ( 116.8548138422182205, 35.98945312608393721, 0.000000000000000000 ) ) ;
#11942=CARTESIAN_POINT ( 'NONE',  ( 200.6228728715779255, 36.58476562716786873, 13.57481594606297115 ) ) ;
#11943=CARTESIAN_POINT ( 'NONE',  ( 104.4587341249999781, 81.87500000136559208, 1.846868145590721655 ) ) ;
#11945=CARTESIAN_POINT ( 'NONE',  ( 59.37712712842213136, 40.15664062716787441, -13.57481594606304753 ) ) ;
#11947=CARTESIAN_POINT ( 'NONE',  ( 185.7049497278729575, 39.85898437608393152, -9.295050272127046043 ) ) ;
#11948=CARTESIAN_POINT ( 'NONE',  ( -8.312177448680279460E-16, 39.31328125216787583, -13.57481594606304576 ) ) ;
#11953=VERTEX_POINT ( 'NONE', #12155 ) ;
#11955=CARTESIAN_POINT ( 'NONE',  ( 208.1451861577817795, 39.41250000108393436, -5.444914386472297529 ) ) ;
#11957=CARTESIAN_POINT ( 'NONE',  ( 0.000000000000000000, -7.395377635281828788, 0.000000000000000000 ) ) ;
#11960=CARTESIAN_POINT ( 'NONE',  ( 13.14518615778179544, 33.21132812608393436, -1.609821015232357215E-15 ) ) ;
#11962=CARTESIAN_POINT ( 'NONE',  ( 65.00000000000000000, 32.07031249999999289, -13.57481594606304576 ) ) ;
#11967=LINE ( 'NONE', #20690, #17141 ) ;
#11970=FACE_OUTER_BOUND ( 'NONE', #18695, .T. ) ;
#11973=CARTESIAN_POINT ( 'NONE',  ( 5.444914386472297529, 32.56640625108394005, -13.14518615778179900 ) ) ;
#11975=ORIENTED_EDGE ( 'NONE', *, *, #7194, .F. ) ;
#11976=CARTESIAN_POINT ( 'NONE',  ( 124.3771271284222877, 36.88242187499999858, -13.57481594606318254 ) ) ;
#11977=DIRECTION ( 'NONE',  ( -1.000000000000000000, 0.000000000000000000, 7.228014483236696740E-18 ) ) ;
#11979=CARTESIAN_POINT ( 'NONE',  ( 208.1451861577817795, 32.96328125108393436, 5.444914386472293977 ) ) ;
#11986=CARTESIAN_POINT ( 'NONE',  ( 181.4251840539369596, 39.46210937716787726, -5.622872871577873077 ) ) ;
#11988=CARTESIAN_POINT ( 'NONE',  ( 116.8548138422182063, 37.32890625108393579, -5.444914386472297529 ) ) ;
#11989=CARTESIAN_POINT ( 'NONE',  ( 5.444914386472297529, 38.12265625108393863, -13.14518615778179722 ) ) ;
#11991=CARTESIAN_POINT ( 'NONE',  ( -9.295050272127044266, 32.71523437608393436, 9.295050272127047819 ) ) ;
#11993=FACE_OUTER_BOUND ( 'NONE', #3056, .T. ) ;
#11996=CARTESIAN_POINT ( 'NONE',  ( 99.99999999999995737, 82.43750000136559208, -4.458734125000016313 ) ) ;
#11998=DIRECTION ( 'NONE',  ( -0.000000000000000000, 1.000000000000000000, -0.000000000000000000 ) ) ;
#12001=( BOUNDED_CURVE ( )  B_SPLINE_CURVE ( 2, ( #22503, #11643, #20219, #13500, #13645, #22360, #15924, #16218, #20651 ),
 .UNSPECIFIED., .F., .F. ) 
 B_SPLINE_CURVE_WITH_KNOTS ( ( 3, 2, 2, 2, 3 ),
 ( 0.4375000000000003331, 0.4479166666666669627, 0.4583333333333335369, 0.4687500000000001665, 0.4791666666666667962 ),
 .UNSPECIFIED. ) 
 CURVE ( )  GEOMETRIC_REPRESENTATION_ITEM ( )  RATIONAL_B_SPLINE_CURVE ( ( 0.9999999999999975575, 0.9238795325112891810, 1.000000000000000000, 0.9238795325112867385, 1.000000000000000000, 0.9238795325112867385, 1.000000000000000000, 0.9238795325112859613, 1.000000000000000888 ) ) 
 REPRESENTATION_ITEM ( '' )  );
#12006=CARTESIAN_POINT ( 'NONE',  ( 124.3771271284221172, 39.66054687716787441, 13.57481594606302444 ) ) ;
#12009=CARTESIAN_POINT ( 'NONE',  ( 65.00000000000000000, 52.00000000000000711, -7.517135062566165128E-15 ) ) ;
#12012=CARTESIAN_POINT ( 'NONE',  ( 200.4449143864723055, 33.06250000108393294, 13.14518615778179189 ) ) ;
#12016=CARTESIAN_POINT ( 'NONE',  ( 3.716534113787486771, 51.46663580899624435, -15.00000000000203215 ) ) ;
#12017=CARTESIAN_POINT ( 'NONE',  ( 193.3947281234233913, 53.60388944777321285, 14.99999999999995559 ) ) ;
#12018=CARTESIAN_POINT ( 'NONE',  ( 143.5748159460630688, 36.73359375216787015, -1.662435489736055892E-15 ) ) ;
#12021=CARTESIAN_POINT ( 'NONE',  ( 200.4449143864723055, 38.61875000108393152, 13.14518615778179189 ) ) ;
#12026=CARTESIAN_POINT ( 'NONE',  ( -10.54595693695916125, 36.00000000000001421, -8.172591659953413412 ) ) ;
#12029=CARTESIAN_POINT ( 'NONE',  ( 74.29505027212704249, 32.51679687608393721, -9.295050272127046043 ) ) ;
#12031=CARTESIAN_POINT ( 'NONE',  ( -9.598844408820454532, 39.61093750216787868, 9.598844408820459861 ) ) ;
#12032=CARTESIAN_POINT ( 'NONE',  ( 214.9999999999999716, 75.00000000000000000, 9.999999999999946709 ) ) ;
#12034=CARTESIAN_POINT ( 'NONE',  ( 130.0000000000000000, 34.05468749999999289, 13.57481594606304576 ) ) ;
#12036=CARTESIAN_POINT ( 'NONE',  ( 78.57481594606305464, 36.58476562499999574, 5.622872871577868636 ) ) ;
#12040=CARTESIAN_POINT ( 'NONE',  ( 130.0000000000000000, 40.15664062608393436, 13.14518615778179544 ) ) ;
#12041=CARTESIAN_POINT ( 'NONE',  ( 55.70494972787295751, 40.45429687608393721, -9.295050272127046043 ) ) ;
#12042=CARTESIAN_POINT ( 'NONE',  ( 53.73518119781812175, 35.99999999999999289, 6.828991891054477570 ) ) ;
#12043=CARTESIAN_POINT ( 'NONE',  ( -8.049105076161786076E-16, 37.18007812608393436, -13.14518615778179544 ) ) ;
#12045=CARTESIAN_POINT ( 'NONE',  ( 184.2131532318158804, 36.00000000000001421, 7.561388982944599491 ) ) ;
#12049=DIRECTION ( 'NONE',  ( 0.000000000000000000, 0.000000000000000000, 1.000000000000000000 ) ) ;
#12050=CARTESIAN_POINT ( 'NONE',  ( 142.6678442549459191, 36.00000000000000711, 4.396229039743236200 ) ) ;
#12053=CARTESIAN_POINT ( 'NONE',  ( 125.0271122604905116, 36.00000000000001421, -12.48139679469847252 ) ) ;
#12054=CARTESIAN_POINT ( 'NONE',  ( 120.4011555911795455, 40.20625000216787726, -9.598844408820458085 ) ) ;
#12057=VECTOR ( 'NONE', #4468, 1000.000000000000000 ) ;
#12062=CARTESIAN_POINT ( 'NONE',  ( 185.4011555911795313, 32.16953124999999147, -9.598844408820458085 ) ) ;
#12064=CARTESIAN_POINT ( 'NONE',  ( 65.00000000000000000, 39.31328125216787583, -13.57481594606304576 ) ) ;
#12065=CARTESIAN_POINT ( 'NONE',  ( 103.1528011352953342, 82.81250000136560629, 3.152801135295355106 ) ) ;
#12066=CARTESIAN_POINT ( 'NONE',  ( 55.70494972787295751, 32.51679687608393721, -9.295050272127046043 ) ) ;
#12071=CARTESIAN_POINT ( 'NONE',  ( -13.57481594606304576, 32.26874999999999716, 0.000000000000000000 ) ) ;
#12073=CARTESIAN_POINT ( 'NONE',  ( 139.2950502721270425, 35.69179687608394147, -9.295050272127046043 ) ) ;
#12075=CARTESIAN_POINT ( 'NONE',  ( 65.00000000000000000, 39.21406249999999716, -13.57481594606304576 ) ) ;
#12077=FACE_OUTER_BOUND ( 'NONE', #2991, .T. ) ;
#12078=CARTESIAN_POINT ( 'NONE',  ( 95.54126587499996504, 84.43750000136560629, -1.387778780781445676E-14 ) ) ;
#12079=CARTESIAN_POINT ( 'NONE',  ( 116.8548138422182063, 38.91640625108393436, -5.444914386472297529 ) ) ;
#12080=CARTESIAN_POINT ( 'NONE',  ( 116.4251840539369596, 38.56914062499999574, -5.622872871577872189 ) ) ;
#12082=CARTESIAN_POINT ( 'NONE',  ( -13.57481594606304753, 38.66835937716786731, -5.622872871577873077 ) ) ;
#12083=AXIS2_PLACEMENT_3D ( 'NONE', #11225, #15215, #4697 ) ;
#12084=VERTEX_POINT ( 'NONE', #17568 ) ;
#12088=CARTESIAN_POINT ( 'NONE',  ( 204.2950502721270425, 40.25585937608393294, -9.295050272127046043 ) ) ;
#12090=CARTESIAN_POINT ( 'NONE',  ( 116.8548138422182205, 39.71015625108393010, -5.444914386472297529 ) ) ;
#12092=DIRECTION ( 'NONE',  ( -0.000000000000000000, 1.000000000000000000, -0.000000000000000000 ) ) ;
#12095=EDGE_CURVE ( 'NONE', #19811, #747, #2052, .T. ) ;
#12096=CARTESIAN_POINT ( 'NONE',  ( 181.8548138422181921, 31.97109375108393436, -5.444914386472297529 ) ) ;
#12097=CARTESIAN_POINT ( 'NONE',  ( 122.2214956318786392, 36.00000000000002132, 10.60546543669468278 ) ) ;
#12103=AXIS2_PLACEMENT_3D ( 'NONE', #12997, #19584, #15144 ) ;
#12105=DIRECTION ( 'NONE',  ( 1.156482317317871478E-16, 0.000000000000000000, 1.000000000000000000 ) ) ;
#12106=CARTESIAN_POINT ( 'NONE',  ( 9.295050272127046043, 34.10429687608393579, -9.295050272127046043 ) ) ;
#12108=EDGE_LOOP ( 'NONE', ( #6597, #22609, #24010, #27440 ) ) ;
#12109=CARTESIAN_POINT ( 'NONE',  ( 101.8468681455906903, 81.37500000136563472, -4.458734125000016313 ) ) ;
#12110=CARTESIAN_POINT ( 'NONE',  ( -13.57481594606304398, 37.87460937499999147, 5.622872871577880183 ) ) ;
#12112=CARTESIAN_POINT ( 'NONE',  ( 195.0000000000000000, 33.60820312608392868, 13.14518615778179544 ) ) ;
#12115=CARTESIAN_POINT ( 'NONE',  ( 194.6713997234275269, 53.49358765998905341, -15.00000000000000000 ) ) ;
#12117=VERTEX_POINT ( 'NONE', #14854 ) ;
#12122=VECTOR ( 'NONE', #20888, 1000.000000000000000 ) ;
#12123=CARTESIAN_POINT ( 'NONE',  ( -9.295050272127044266, 38.46992187608393721, 9.295050272127047819 ) ) ;
#12124=CARTESIAN_POINT ( 'NONE',  ( -5.444914386472297529, 33.26093750108393721, -13.14518615778179900 ) ) ;
#12130=VECTOR ( 'NONE', #11998, 1000.000000000000000 ) ;
#12131=CARTESIAN_POINT ( 'NONE',  ( 96.84719886470459471, 81.56250000136559208, -3.152801135295383084 ) ) ;
#12133=CARTESIAN_POINT ( 'NONE',  ( -8.312177448680279460E-16, 38.51953125216787299, -13.57481594606304576 ) ) ;
#12135=CARTESIAN_POINT ( 'NONE',  ( 189.3771271284220177, 38.46992187499999005, -13.57481594606295339 ) ) ;
#12140=FACE_OUTER_BOUND ( 'NONE', #8881, .T. ) ;
#12145=CARTESIAN_POINT ( 'NONE',  ( 55.70494972787295751, 36.88242187608393152, 9.295050272127047819 ) ) ;
#12146=DIRECTION ( 'NONE',  ( 0.000000000000000000, 0.000000000000000000, -1.000000000000000000 ) ) ;
#12147=CARTESIAN_POINT ( 'NONE',  ( 204.2950502721270425, 32.31835937608393294, 9.295050272127046043 ) ) ;
#12151=CARTESIAN_POINT ( 'NONE',  ( -5.323790963956732902, 54.47170356488336296, -15.00000000000000000 ) ) ;
#12152=CARTESIAN_POINT ( 'NONE',  ( 185.8198241863519797, 55.00000000000000000, 14.99999999999995204 ) ) ;
#12153=CARTESIAN_POINT ( 'NONE',  ( 139.5988444088204687, 38.22187500216787015, 9.598844408820456309 ) ) ;
#12155=CARTESIAN_POINT ( 'NONE',  ( 185.8198241863519797, 55.00000000000000000, 14.99999999999995204 ) ) ;
#12156=CARTESIAN_POINT ( 'NONE',  ( 181.8548138422182205, 36.78320312608393294, 0.000000000000000000 ) ) ;
#12157=VERTEX_POINT ( 'NONE', #27994 ) ;
#12159=ORIENTED_EDGE ( 'NONE', *, *, #1638, .F. ) ;
#12161=CARTESIAN_POINT ( 'NONE',  ( -12.56650672479864461, 36.00000000000000000, -4.295155080288879823 ) ) ;
#12163=CARTESIAN_POINT ( 'NONE',  ( 1.662435489736055498E-15, -7.395377635281828788, -13.57481594606304398 ) ) ;
#12166=CARTESIAN_POINT ( 'NONE',  ( 13.57481594606304576, 40.60312499999999858, -1.662435489736055892E-15 ) ) ;
#12168=CARTESIAN_POINT ( 'NONE',  ( 94.99999999999995737, 83.00000000000000000, -1.387778780781445676E-14 ) ) ;
#12169=CARTESIAN_POINT ( 'NONE',  ( 139.5988444088204687, 35.74140624999999716, 9.598844408820456309 ) ) ;
#12170=ORIENTED_EDGE ( 'NONE', *, *, #24323, .T. ) ;
#12172=CARTESIAN_POINT ( 'NONE',  ( 65.00000000000000000, 36.83281249999999574, -13.57481594606304576 ) ) ;
#12176=CARTESIAN_POINT ( 'NONE',  ( 139.2950502721270425, 38.07304687608393579, -9.295050272127046043 ) ) ;
#12177=CARTESIAN_POINT ( 'NONE',  ( 78.14518615778179367, 37.72578125108393721, 5.444914386472293977 ) ) ;
#12178=ORIENTED_EDGE ( 'NONE', *, *, #26923, .F. ) ;
#12181=CARTESIAN_POINT ( 'NONE',  ( -5.444914386472299306, 39.11484375108394573, 13.14518615778179722 ) ) ;
#12183=CARTESIAN_POINT ( 'NONE',  ( 181.9040934463640156, 36.00000000000000000, 1.137167824541468031 ) ) ;
#12185=CARTESIAN_POINT ( 'NONE',  ( 195.0000000000000000, 31.62382812608393579, -13.14518615778179544 ) ) ;
#12186=CARTESIAN_POINT ( 'NONE',  ( 140.5630829503604673, 36.00000000000000711, 8.196709705857037065 ) ) ;
#12190=CARTESIAN_POINT ( 'NONE',  ( 119.4540428948962330, 35.99999999999999289, -8.172591786207229703 ) ) ;
#12201=CARTESIAN_POINT ( 'NONE',  ( 95.54126587499995082, 83.75000000136560629, 1.846868145590724986 ) ) ;
#12202=CARTESIAN_POINT ( 'NONE',  ( 65.00000000000000000, 39.36289062608393152, 13.14518615778179544 ) ) ;
#12208=CARTESIAN_POINT ( 'NONE',  ( 116.8548138422182205, 34.40195312608393152, 0.000000000000000000 ) ) ;
#12210=CARTESIAN_POINT ( 'NONE',  ( 143.5748159460630688, 37.47773437716787015, 5.622872871577868636 ) ) ;
#12213=CARTESIAN_POINT ( 'NONE',  ( 143.1451861577818079, 38.51953125108393294, 5.444914386472293977 ) ) ;
#12214=CARTESIAN_POINT ( 'NONE',  ( 78.57481594606304043, 39.85898437716787157, 5.622872871577869525 ) ) ;
#12218=CARTESIAN_POINT ( 'NONE',  ( 5.622872871577878406, 39.75976562716787299, 13.57481594606304576 ) ) ;
#12223=CARTESIAN_POINT ( 'NONE',  ( 195.0000000000000000, 31.37578125216787583, -13.57481594606304576 ) ) ;
#12226=CARTESIAN_POINT ( 'NONE',  ( 124.5550856135277087, 37.52734375108393294, 13.14518615778179722 ) ) ;
#12228=CARTESIAN_POINT ( 'NONE',  ( 130.0000000000000000, -7.395377635281828788, -13.57481594606305997 ) ) ;
#12231=CARTESIAN_POINT ( 'NONE',  ( 208.5748159460630688, 37.42812499999999432, -1.662435489736055892E-15 ) ) ;
#12233=CARTESIAN_POINT ( 'NONE',  ( 130.2703369776646696, 35.99999999999998579, 13.14949859323919945 ) ) ;
#12235=CARTESIAN_POINT ( 'NONE',  ( -8.312177448680279460E-16, 37.72578125216787726, -13.57481594606304576 ) ) ;
#12238=( GEOMETRIC_REPRESENTATION_CONTEXT ( 3 ) GLOBAL_UNCERTAINTY_ASSIGNED_CONTEXT ( ( #14956 ) ) GLOBAL_UNIT_ASSIGNED_CONTEXT ( ( #13307, #228, #17752 ) ) REPRESENTATION_CONTEXT ( 'NONE', 'WORKASPACE' ) );
#12241=DIRECTION ( 'NONE',  ( 0.000000000000000000, -0.000000000000000000, 1.000000000000000000 ) ) ;
#12242=CARTESIAN_POINT ( 'NONE',  ( 9.598844408820456309, 40.70234374999999716, -9.598844408820458085 ) ) ;
#12243=EDGE_LOOP ( 'NONE', ( #27189, #27506, #24159, #21542 ) ) ;
#12244=CARTESIAN_POINT ( 'NONE',  ( 103.1528011352953342, 84.31250000136560629, -3.152801135295383084 ) ) ;
#12245=ADVANCED_FACE ( 'NONE', ( #55 ), #19571, .T. ) ;
#12246=( BOUNDED_CURVE ( )  B_SPLINE_CURVE ( 2, ( #21051, #27203, #28128, #3528, #9789, #7655, #7929, #14476, #7797 ),
 .UNSPECIFIED., .F., .F. ) 
 B_SPLINE_CURVE_WITH_KNOTS ( ( 3, 2, 2, 2, 3 ),
 ( 0.02083333333333358892, 0.03125000000000020123, 0.04166666666666681007, 0.05208333333333342585, 0.06250000000000004163 ),
 .UNSPECIFIED. ) 
 CURVE ( )  GEOMETRIC_REPRESENTATION_ITEM ( )  RATIONAL_B_SPLINE_CURVE ( ( 0.9999999999999981126, 0.9238795325112886259, 1.000000000000000000, 0.9238795325112867385, 1.000000000000000000, 0.9238795325112867385, 1.000000000000000000, 0.9238795325112864054, 1.000000000000000222 ) ) 
 REPRESENTATION_ITEM ( '' )  );
#12249=ORIENTED_EDGE ( 'NONE', *, *, #2356, .T. ) ;
#12250=EDGE_CURVE ( 'NONE', #24277, #8963, #8735, .T. ) ;
#12251=CARTESIAN_POINT ( 'NONE',  ( 192.7238531554485803, 51.46995505939284499, -14.99999999999966072 ) ) ;
#12257=CARTESIAN_POINT ( 'NONE',  ( 189.3771271284221314, 39.66054687716786731, 13.57481594606304753 ) ) ;
#12260=ADVANCED_FACE ( 'NONE', ( #8876 ), #14580, .T. ) ;
#12262=CARTESIAN_POINT ( 'NONE',  ( 120.7049497278729575, 38.27148437608393294, -9.295050272127046043 ) ) ;
#12263=CARTESIAN_POINT ( 'NONE',  ( -9.295050272127046043, 31.72304687608393081, -9.295050272127046043 ) ) ;
#12264=CARTESIAN_POINT ( 'NONE',  ( 78.57481594606304043, 38.17226562499999432, 5.622872871577869525 ) ) ;
#12265=DIRECTION ( 'NONE',  ( 0.000000000000000000, 0.000000000000000000, 1.000000000000000000 ) ) ;
#12266=EDGE_CURVE ( 'NONE', #16468, #8963, #10009, .T. ) ;
#12270=CARTESIAN_POINT ( 'NONE',  ( 99.99999999999995737, 81.43750000136559208, -4.458734125000016313 ) ) ;
#12273=CARTESIAN_POINT ( 'NONE',  ( 72.61652532548083627, 54.91574374957784954, 14.99999999999997691 ) ) ;
#12274=ORIENTED_EDGE ( 'NONE', *, *, #19255, .F. ) ;
#12277=DIRECTION ( 'NONE',  ( 0.000000000000000000, -1.000000000000000000, 0.000000000000000000 ) ) ;
#12280=CARTESIAN_POINT ( 'NONE',  ( -13.57481594606304398, 40.25585937499999289, 5.622872871577880183 ) ) ;
#12282=AXIS2_PLACEMENT_3D ( 'NONE', #26066, #25644, #19513 ) ;
#12285=ORIENTED_EDGE ( 'NONE', *, *, #3429, .F. ) ;
#12286=CARTESIAN_POINT ( 'NONE',  ( 74.29505027212704249, 38.66835937608393436, 9.295050272127046043 ) ) ;
#12289=VERTEX_POINT ( 'NONE', #7870 ) ;
#12293=CARTESIAN_POINT ( 'NONE',  ( 0.000000000000000000, -7.395377635281828788, 13.57481594606304398 ) ) ;
#12294=CARTESIAN_POINT ( 'NONE',  ( 51.90409344636400846, 36.00000000000000000, 1.137167824541468031 ) ) ;
#12296=CARTESIAN_POINT ( 'NONE',  ( 116.4251840539369596, 34.79882812716787299, 5.622872871577880183 ) ) ;
#12298=DIRECTION ( 'NONE',  ( 1.156482317317871478E-16, 0.000000000000000000, 1.000000000000000000 ) ) ;
#12299=CARTESIAN_POINT ( 'NONE',  ( 189.5550856135277229, 36.63437500108393152, -13.14518615778179900 ) ) ;
#12300=EDGE_LOOP ( 'NONE', ( #6188, #17978, #10811, #5051 ) ) ;
#12302=ORIENTED_EDGE ( 'NONE', *, *, #16630, .T. ) ;
#12306=CARTESIAN_POINT ( 'NONE',  ( 104.4587341249999639, 83.93750000136560629, -1.442382525525748735E-14 ) ) ;
#12315=CARTESIAN_POINT ( 'NONE',  ( 99.99999999999995737, 84.25000000000000000, 4.999999999999990230 ) ) ;
#12320=CARTESIAN_POINT ( 'NONE',  ( 139.2950502721270425, 38.86679687608393863, -9.295050272127046043 ) ) ;
#12321=CARTESIAN_POINT ( 'NONE',  ( 65.00000000000000000, 35.59257812608393579, -13.14518615778179544 ) ) ;
#12324=CARTESIAN_POINT ( 'NONE',  ( -18.00000000000000355, 78.00000000000000000, 13.00000000000000178 ) ) ;
#12325=CARTESIAN_POINT ( 'NONE',  ( 9.295050272127046043, 35.49335937608393010, -9.295050272127046043 ) ) ;
#12328=CARTESIAN_POINT ( 'NONE',  ( 142.0772764098356333, 36.00000000000000000, -6.197985357349214297 ) ) ;
#12330=CARTESIAN_POINT ( 'NONE',  ( 120.4011555911795455, 40.10703124999999147, -9.598844408820458085 ) ) ;
#12331=ORIENTED_EDGE ( 'NONE', *, *, #16454, .T. ) ;
#12332=DIRECTION ( 'NONE',  ( 1.000000000000000000, 0.000000000000000000, 0.000000000000000000 ) ) ;
#12333=CARTESIAN_POINT ( 'NONE',  ( -9.295050272127046043, 37.27929687608393294, -9.295050272127046043 ) ) ;
#12334=CARTESIAN_POINT ( 'NONE',  ( 136.8311344573049553, 36.00000000000000000, 11.35217666745991671 ) ) ;
#12337=CARTESIAN_POINT ( 'NONE',  ( 134.1572863549629062, 35.99999999999997868, -12.92256159328817411 ) ) ;
#12338=LINE ( 'NONE', #10195, #28190 ) ;
#12347=CARTESIAN_POINT ( 'NONE',  ( 98.15313185440925281, 84.50000000136562051, -4.458734125000016313 ) ) ;
#12348=CARTESIAN_POINT ( 'NONE',  ( 78.14518615778179367, 38.81718750108393579, -5.444914386472297529 ) ) ;
#12354=CARTESIAN_POINT ( 'NONE',  ( 120.4011555911795455, 40.90078124999999432, -9.598844408820458085 ) ) ;
#12358=CARTESIAN_POINT ( 'NONE',  ( 96.84719886470459471, 80.31250000136559208, -3.152801135295383084 ) ) ;
#12359=CARTESIAN_POINT ( 'NONE',  ( 120.7049497278729575, 38.86679687608393863, -9.295050272127046043 ) ) ;
#12360=CARTESIAN_POINT ( 'NONE',  ( 65.00000000000000000, 38.51953125216787299, -13.57481594606304576 ) ) ;
#12362=CARTESIAN_POINT ( 'NONE',  ( -9.598844408820458085, 34.65000000216787868, -9.598844408820458085 ) ) ;
#12363=ORIENTED_EDGE ( 'NONE', *, *, #12606, .T. ) ;
#12367=CARTESIAN_POINT ( 'NONE',  ( 185.7049497278729575, 36.68398437608392726, 9.295050272127047819 ) ) ;
#12368=( BOUNDED_SURFACE ( )  B_SPLINE_SURFACE ( 1, 2, ( 
 ( #11166, #17454, #9192, #17597, #15451, #11309, #2369, #10891, #26303, #4501, #19883, #20031, #13443, #11027, #19738, #22170, #6766, #24164, #2647, #511, #18462, #25145, #14300, #13874, #18315, #799, #16448, #26882, #27305, #22742, #11877, #9891, #16315, #7762, #5068, #24586, #5635, #23018, #27024, #9752, #3489, #16164, #12153, #7469, #20879, #1365, #10026, #13732, #27169, #5210, #20459, #24871, #5354, #3208, #7328, #15876, #9612, #9468, #18735, #7623, #27433, #22455, #1084, #20600, #25015, #5493, #14162, #3348, #2922, #22881, #22600, #11592, #12018, #20312, #20741, #18170, #16016, #1226, #941, #18602, #24730, #3069, #11734, #14019, #1917, #12431, #27715, #7897, #6049, #12566, #21020, #8453, #25700, #23157, #14714, #14849, #10583, #14992, #23709, #19003, #16867, #18864, #21294, #12714, #19148, #25565, #27992, #27853, #8310, #17140, #17000, #12296, #23432, #10720, #8177, #16591, #21437, #4185, #23570, #3906, #4051, #21151, #1777, #3632, #6316, #14442, #19291, #10442, #10296, #25285, #25841, #6182, #12846, #1500, #21575, #27576, #8034, #2050, #19427, #5771, #3772, #25431, #10154, #5914, #16732, #14579, #1637, #23298, #28127, #26268, #4603, #12982, #477, #17713, #15126, #6730, #6874, #2614, #7009, #15705, #10992, #8872, #10854, #13262, #4749, #11132, #17564, #19998, #19847, #333, #9160, #9020, #4324, #15416, #2756, #19705, #8592, #13409, #24407, #15558, #190, #24267, #13124 ),
 ( #22136, #21859, #24131, #11277, #6588, #17282, #2334, #21719, #21995, #17852, #2471, #15270, #11419, #4467, #26415, #23988, #26555, #4894, #13558, #22281, #25984, #6454, #23847, #2193, #19566, #50, #8731, #17424, #26122, #3032, #5176, #18284, #11559, #20712, #619, #11701, #24977, #7435, #20275, #24838, #9723, #13840, #16130, #1051, #26990, #22565, #7585, #3178, #7295, #5460, #910, #14129, #5321, #13701, #20426, #18425, #24554, #9580, #13980, #15984, #22418, #5035, #16278, #2889, #22708, #11988, #762, #9293, #11848, #22850, #20570, #3317, #18135, #1194, #20139, #17990, #26700, #27133, #9435, #7149, #26848, #15844, #24698, #10966, #164, #4577, #25812, #2589, #6560, #19821, #26387, #28100, #17397, #10824, #13091, #8564, #22110, #27961, #26095, #8991, #2309, #17254, #19678, #21969, #22, #8846, #13237, #21832, #8704, #305, #6698, #4296, #6842, #15240, #15532, #17536, #2019, #23960, #2446, #12820, #4439, #26240, #12954, #21544, #4160, #17681, #10688, #15385, #13382, #19395, #8418, #24099, #24240, #11107, #4722, #15097, #19261, #17107, #6286, #14963, #23818, #23683, #25955, #6428, #21687, #2162, #19540, #4868, #24671, #26963, #3002, #22252, #20397, #2729, #6984, #5010, #22823, #19968, #11820, #18396, #13675, #22681, #447, #2862, #3151, #7554, #16101, #24807, #11530, #20543, #5290, #20113, #9554, #15679, #11676, #11251, #590, #1025, #15819, #9696, #27103, #24380, #22391 ) ),
 .UNSPECIFIED., .F., .F., .F. ) 
 B_SPLINE_SURFACE_WITH_KNOTS ( ( 2, 2 ),
 ( 3, 2, 2, 2, 2, 2, 2, 2, 2, 2, 2, 2, 2, 2, 2, 2, 2, 2, 2, 2, 2, 2, 2, 2, 2, 2, 2, 2, 2, 2, 2, 2, 2, 2, 2, 2, 2, 2, 2, 2, 2, 2, 2, 2, 2, 2, 2, 2, 2, 2, 2, 2, 2, 2, 2, 2, 2, 2, 2, 2, 2, 2, 2, 2, 2, 2, 2, 2, 2, 2, 2, 2, 2, 2, 2, 2, 2, 2, 2, 2, 2, 2, 2, 2, 2, 2, 2, 2, 2, 2, 2, 3 ),
 ( 0.000000000000000000, 1.000000000000000000 ),
 ( 0.000000000000000000, 0.01041666666666666609, 0.02083333333333333218, 0.03125000000000000000, 0.04166666666666666435, 0.05208333333333333565, 0.06250000000000000000, 0.07291666666666667129, 0.08333333333333332871, 0.09375000000000000000, 0.1041666666666666713, 0.1145833333333333287, 0.1250000000000000000, 0.1354166666666666574, 0.1458333333333333426, 0.1562500000000000000, 0.1666666666666666574, 0.1770833333333333426, 0.1875000000000000000, 0.1979166666666666574, 0.2083333333333333426, 0.2187500000000000000, 0.2291666666666666574, 0.2395833333333333426, 0.2500000000000000000, 0.2604166666666666852, 0.2708333333333333148, 0.2812500000000000000, 0.2916666666666666852, 0.3020833333333333148, 0.3125000000000000000, 0.3229166666666666852, 0.3333333333333333148, 0.3437500000000000000, 0.3541666666666666852, 0.3645833333333333148, 0.3750000000000000000, 0.3854166666666666852, 0.3958333333333333148, 0.4062500000000000000, 0.4166666666666666852, 0.4270833333333333148, 0.4375000000000000000, 0.4479166666666666852, 0.4583333333333333148, 0.4687500000000000000, 0.4791666666666666852, 0.4895833333333333148, 0.5000000000000000000, 0.5104166666666666297, 0.5208333333333333703, 0.5312500000000000000, 0.5416666666666666297, 0.5520833333333333703, 0.5625000000000000000, 0.5729166666666666297, 0.5833333333333333703, 0.5937500000000000000, 0.6041666666666666297, 0.6145833333333333703, 0.6250000000000000000, 0.6354166666666666297, 0.6458333333333333703, 0.6562500000000000000, 0.6666666666666666297, 0.6770833333333333703, 0.6875000000000000000, 0.6979166666666666297, 0.7083333333333333703, 0.7187500000000000000, 0.7291666666666666297, 0.7395833333333333703, 0.7500000000000000000, 0.7604166666666666297, 0.7708333333333333703, 0.7812500000000000000, 0.7916666666666666297, 0.8020833333333333703, 0.8125000000000000000, 0.8229166666666666297, 0.8333333333333333703, 0.8437500000000000000, 0.8541666666666666297, 0.8645833333333333703, 0.8750000000000000000, 0.8854166666666666297, 0.8958333333333333703, 0.9062500000000000000, 0.9166666666666666297, 0.9270833333333333703, 0.9375000000000000000, 0.9448586970929392370 ),
 .UNSPECIFIED. ) 
 GEOMETRIC_REPRESENTATION_ITEM ( )  RATIONAL_B_SPLINE_SURFACE ( (
 ( 1.000000000000000000, 0.9238795325112867385, 1.000000000000000000, 0.9238795325112867385, 1.000000000000000000, 0.9238795325112867385, 1.000000000000000000, 0.9238795325112867385, 1.000000000000000000, 0.9238795325112867385, 1.000000000000000000, 0.9238795325112867385, 1.000000000000000000, 0.9238795325112867385, 1.000000000000000000, 0.9238795325112867385, 1.000000000000000000, 0.9238795325112867385, 1.000000000000000000, 0.9238795325112867385, 1.000000000000000000, 0.9238795325112867385, 1.000000000000000000, 0.9238795325112867385, 1.000000000000000000, 0.9238795325112867385, 1.000000000000000000, 0.9238795325112867385, 1.000000000000000000, 0.9238795325112867385, 1.000000000000000000, 0.9238795325112867385, 1.000000000000000000, 0.9238795325112867385, 1.000000000000000000, 0.9238795325112867385, 1.000000000000000000, 0.9238795325112867385, 1.000000000000000000, 0.9238795325112867385, 1.000000000000000000, 0.9238795325112867385, 1.000000000000000000, 0.9238795325112867385, 1.000000000000000000, 0.9238795325112867385, 1.000000000000000000, 0.9238795325112867385, 1.000000000000000000, 0.9238795325112867385, 1.000000000000000000, 0.9238795325112867385, 1.000000000000000000, 0.9238795325112867385, 1.000000000000000000, 0.9238795325112867385, 1.000000000000000000, 0.9238795325112867385, 1.000000000000000000, 0.9238795325112867385, 1.000000000000000000, 0.9238795325112867385, 1.000000000000000000, 0.9238795325112867385, 1.000000000000000000, 0.9238795325112867385, 1.000000000000000000, 0.9238795325112867385, 1.000000000000000000, 0.9238795325112867385, 1.000000000000000000, 0.9238795325112867385, 1.000000000000000000, 0.9238795325112867385, 1.000000000000000000, 0.9238795325112867385, 1.000000000000000000, 0.9238795325112867385, 1.000000000000000000, 0.9238795325112867385, 1.000000000000000000, 0.9238795325112867385, 1.000000000000000000, 0.9238795325112867385, 1.000000000000000000, 0.9238795325112867385, 1.000000000000000000, 0.9238795325112867385, 1.000000000000000000, 0.9238795325112867385, 1.000000000000000000, 0.9238795325112867385, 1.000000000000000000, 0.9238795325112867385, 1.000000000000000000, 0.9238795325112867385, 1.000000000000000000, 0.9238795325112867385, 1.000000000000000000, 0.9238795325112867385, 1.000000000000000000, 0.9238795325112867385, 1.000000000000000000, 0.9238795325112867385, 1.000000000000000000, 0.9238795325112867385, 1.000000000000000000, 0.9238795325112867385, 1.000000000000000000, 0.9238795325112867385, 1.000000000000000000, 0.9238795325112867385, 1.000000000000000000, 0.9238795325112867385, 1.000000000000000000, 0.9238795325112867385, 1.000000000000000000, 0.9238795325112867385, 1.000000000000000000, 0.9238795325112867385, 1.000000000000000000, 0.9238795325112867385, 1.000000000000000000, 0.9238795325112867385, 1.000000000000000000, 0.9238795325112867385, 1.000000000000000000, 0.9238795325112867385, 1.000000000000000000, 0.9238795325112867385, 1.000000000000000000, 0.9238795325112867385, 1.000000000000000000, 0.9238795325112867385, 1.000000000000000000, 0.9238795325112867385, 1.000000000000000000, 0.9238795325112867385, 1.000000000000000000, 0.9238795325112867385, 1.000000000000000000, 0.9238795325112867385, 1.000000000000000000, 0.9238795325112867385, 1.000000000000000000, 0.9238795325112867385, 1.000000000000000000, 0.9238795325112867385, 1.000000000000000000, 0.9238795325112867385, 1.000000000000000000, 0.9238795325112867385, 1.000000000000000000, 0.9238795325112867385, 1.000000000000000000, 0.9238795325112867385, 1.000000000000000000, 0.9238795325112867385, 1.000000000000000000, 0.9238795325112867385, 1.000000000000000000, 0.9238795325112867385, 1.000000000000000000, 0.9238795325112867385, 1.000000000000000000, 0.9238795325112867385, 1.000000000000000000, 0.9238795325112867385, 1.000000000000000000, 0.9238795325112867385, 1.000000000000000000, 0.9238795325112867385, 1.000000000000000000, 0.9238795325112867385, 1.000000000000000000, 0.9238795325112867385, 1.000000000000000000, 0.9238795325112867385, 1.000000000000000000, 0.9238795325112867385, 1.000000000000000000, 0.9462258435690522607, 0.9684275710300105366),
 ( 1.000000000000000000, 0.9238795325112867385, 1.000000000000000000, 0.9238795325112867385, 1.000000000000000000, 0.9238795325112867385, 1.000000000000000000, 0.9238795325112867385, 1.000000000000000000, 0.9238795325112867385, 1.000000000000000000, 0.9238795325112867385, 1.000000000000000000, 0.9238795325112867385, 1.000000000000000000, 0.9238795325112867385, 1.000000000000000000, 0.9238795325112867385, 1.000000000000000000, 0.9238795325112867385, 1.000000000000000000, 0.9238795325112867385, 1.000000000000000000, 0.9238795325112867385, 1.000000000000000000, 0.9238795325112867385, 1.000000000000000000, 0.9238795325112867385, 1.000000000000000000, 0.9238795325112867385, 1.000000000000000000, 0.9238795325112867385, 1.000000000000000000, 0.9238795325112867385, 1.000000000000000000, 0.9238795325112867385, 1.000000000000000000, 0.9238795325112867385, 1.000000000000000000, 0.9238795325112867385, 1.000000000000000000, 0.9238795325112867385, 1.000000000000000000, 0.9238795325112867385, 1.000000000000000000, 0.9238795325112867385, 1.000000000000000000, 0.9238795325112867385, 1.000000000000000000, 0.9238795325112867385, 1.000000000000000000, 0.9238795325112867385, 1.000000000000000000, 0.9238795325112867385, 1.000000000000000000, 0.9238795325112867385, 1.000000000000000000, 0.9238795325112867385, 1.000000000000000000, 0.9238795325112867385, 1.000000000000000000, 0.9238795325112867385, 1.000000000000000000, 0.9238795325112867385, 1.000000000000000000, 0.9238795325112867385, 1.000000000000000000, 0.9238795325112867385, 1.000000000000000000, 0.9238795325112867385, 1.000000000000000000, 0.9238795325112867385, 1.000000000000000000, 0.9238795325112867385, 1.000000000000000000, 0.9238795325112867385, 1.000000000000000000, 0.9238795325112867385, 1.000000000000000000, 0.9238795325112867385, 1.000000000000000000, 0.9238795325112867385, 1.000000000000000000, 0.9238795325112867385, 1.000000000000000000, 0.9238795325112867385, 1.000000000000000000, 0.9238795325112867385, 1.000000000000000000, 0.9238795325112867385, 1.000000000000000000, 0.9238795325112867385, 1.000000000000000000, 0.9238795325112867385, 1.000000000000000000, 0.9238795325112867385, 1.000000000000000000, 0.9238795325112867385, 1.000000000000000000, 0.9238795325112867385, 1.000000000000000000, 0.9238795325112867385, 1.000000000000000000, 0.9238795325112867385, 1.000000000000000000, 0.9238795325112867385, 1.000000000000000000, 0.9238795325112867385, 1.000000000000000000, 0.9238795325112867385, 1.000000000000000000, 0.9238795325112867385, 1.000000000000000000, 0.9238795325112867385, 1.000000000000000000, 0.9238795325112867385, 1.000000000000000000, 0.9238795325112867385, 1.000000000000000000, 0.9238795325112867385, 1.000000000000000000, 0.9238795325112867385, 1.000000000000000000, 0.9238795325112867385, 1.000000000000000000, 0.9238795325112867385, 1.000000000000000000, 0.9238795325112867385, 1.000000000000000000, 0.9238795325112867385, 1.000000000000000000, 0.9238795325112867385, 1.000000000000000000, 0.9238795325112867385, 1.000000000000000000, 0.9238795325112867385, 1.000000000000000000, 0.9238795325112867385, 1.000000000000000000, 0.9238795325112867385, 1.000000000000000000, 0.9238795325112867385, 1.000000000000000000, 0.9238795325112867385, 1.000000000000000000, 0.9238795325112867385, 1.000000000000000000, 0.9238795325112867385, 1.000000000000000000, 0.9238795325112867385, 1.000000000000000000, 0.9238795325112867385, 1.000000000000000000, 0.9238795325112867385, 1.000000000000000000, 0.9238795325112867385, 1.000000000000000000, 0.9238795325112867385, 1.000000000000000000, 0.9238795325112867385, 1.000000000000000000, 0.9238795325112867385, 1.000000000000000000, 0.9238795325112867385, 1.000000000000000000, 0.9238795325112867385, 1.000000000000000000, 0.9238795325112867385, 1.000000000000000000, 0.9238795325112867385, 1.000000000000000000, 0.9238795325112867385, 1.000000000000000000, 0.9238795325112867385, 1.000000000000000000, 0.9238795325112867385, 1.000000000000000000, 0.9238795325112867385, 1.000000000000000000, 0.9238795325112867385, 1.000000000000000000, 0.9462258435690522607, 0.9684275710300105366) ) ) 
 REPRESENTATION_ITEM ( '' )  SURFACE ( )  );
#12370=CARTESIAN_POINT ( 'NONE',  ( 143.1451861577818363, 38.61875000108392442, -5.444914386472297529 ) ) ;
#12371=CARTESIAN_POINT ( 'NONE',  ( 13.14518615778179900, 32.46718750108393436, -5.444914386472297529 ) ) ;
#12376=CARTESIAN_POINT ( 'NONE',  ( 185.4011555911795313, 39.31328124999999574, -9.598844408820458085 ) ) ;
#12377=CARTESIAN_POINT ( 'NONE',  ( 65.00000000000000000, 39.61093749999999147, 13.57481594606304576 ) ) ;
#12379=CARTESIAN_POINT ( 'NONE',  ( 65.00000000000000000, 37.57695312608392868, 13.14518615778179544 ) ) ;
#12385=CARTESIAN_POINT ( 'NONE',  ( 124.3771271284221740, 39.26367187500000000, -13.57481594606310260 ) ) ;
#12386=CARTESIAN_POINT ( 'NONE',  ( 13.57481594606304931, 38.96601562499999005, 5.622872871577869525 ) ) ;
#12389=ORIENTED_EDGE ( 'NONE', *, *, #27810, .F. ) ;
#12390=VECTOR ( 'NONE', #11360, 1000.000000000000000 ) ;
#12396=CARTESIAN_POINT ( 'NONE',  ( 181.4251840539369596, 40.30546875216787583, 0.000000000000000000 ) ) ;
#12399=CARTESIAN_POINT ( 'NONE',  ( 130.0000000000000000, 38.17226562608394147, -13.14518615778179544 ) ) ;
#12400=CARTESIAN_POINT ( 'NONE',  ( 5.444914386472302859, 32.07031250108393294, 13.14518615778179189 ) ) ;
#12402=CARTESIAN_POINT ( 'NONE',  ( 65.00000000000000000, 37.22968749999999716, 13.57481594606304576 ) ) ;
#12410=EDGE_CURVE ( 'NONE', #21487, #27401, #20574, .T. ) ;
#12411=CARTESIAN_POINT ( 'NONE',  ( 104.4587341249999639, 84.18750000136560629, -1.442382525525748735E-14 ) ) ;
#12413=CARTESIAN_POINT ( 'NONE',  ( -13.14518615778179900, 39.11484375108394573, -5.444914386472297529 ) ) ;
#12414=CARTESIAN_POINT ( 'NONE',  ( 74.18017581364799184, 55.00000000000000000, 14.99999999999997868 ) ) ;
#12420=CYLINDRICAL_SURFACE ( 'NONE', #9089, 13.57481594606304398 ) ;
#12422=CARTESIAN_POINT ( 'NONE',  ( 130.0000000000000000, 39.71015625216787015, 13.57481594606304576 ) ) ;
#12424=CARTESIAN_POINT ( 'NONE',  ( 65.00000000000000000, 39.75976562608394005, -13.14518615778179544 ) ) ;
#12428=CARTESIAN_POINT ( 'NONE',  ( 78.57481594606305464, 37.37851562499999858, 5.622872871577868636 ) ) ;
#12429=CARTESIAN_POINT ( 'NONE',  ( 124.3771271284220319, 37.97382812499999716, 13.57481594606295161 ) ) ;
#12431=CARTESIAN_POINT ( 'NONE',  ( 135.6228728715778686, 36.08867187716787583, -13.57481594606304753 ) ) ;
#12433=CARTESIAN_POINT ( 'NONE',  ( 204.2950502721270425, 36.48554687608393721, -9.295050272127046043 ) ) ;
#12435=FACE_OUTER_BOUND ( 'NONE', #18045, .T. ) ;
#12437=EDGE_CURVE ( 'NONE', #13724, #10805, #16843, .T. ) ;
#12438=LINE ( 'NONE', #12163, #21994 ) ;
#12439=CARTESIAN_POINT ( 'NONE',  ( -20.00000000000000355, 55.00000000000000000, -14.99999999999999822 ) ) ;
#12440=CYLINDRICAL_SURFACE ( 'NONE', #28192, 5.000000000000000888 ) ;
#12442=CARTESIAN_POINT ( 'NONE',  ( 12.53142549111993098, 36.00000000000000711, -5.200562670743043903 ) ) ;
#12443=DIRECTION ( 'NONE',  ( -0.000000000000000000, 1.000000000000000000, -0.000000000000000000 ) ) ;
#12445=ADVANCED_FACE ( 'NONE', ( #11993 ), #7731, .F. ) ;
#12446=ORIENTED_EDGE ( 'NONE', *, *, #27435, .T. ) ;
#12451=CARTESIAN_POINT ( 'NONE',  ( 136.9444263933115167, 31.55306875057403104, -11.16113171639042356 ) ) ;
#12452=CARTESIAN_POINT ( 'NONE',  ( 55.70494972787295751, 38.27148437608393294, 9.295050272127047819 ) ) ;
#12454=CARTESIAN_POINT ( 'NONE',  ( 201.9444263933115167, 31.55306875057403104, -11.16113171639042356 ) ) ;
#12455=CARTESIAN_POINT ( 'NONE',  ( 56.87469608220845174, 36.00000000000000000, 10.34220695173551441 ) ) ;
#12456=CARTESIAN_POINT ( 'NONE',  ( -13.14518615778179544, 34.20351562608393436, 0.000000000000000000 ) ) ;
#12457=CARTESIAN_POINT ( 'NONE',  ( 0.000000000000000000, 50.00000000000000000, 13.57481594606304398 ) ) ;
#12460=DIRECTION ( 'NONE',  ( 0.000000000000000000, 0.000000000000000000, 1.000000000000000000 ) ) ;
#12461=CARTESIAN_POINT ( 'NONE',  ( 5.444914386472297529, 37.13046875108393152, -13.14518615778179900 ) ) ;
#12462=CARTESIAN_POINT ( 'NONE',  ( 195.0000000000000000, -7.395377635281828788, -2.255140518769849538E-14 ) ) ;
#12467=CARTESIAN_POINT ( 'NONE',  ( 185.4011555911795313, 39.41250000216787441, -9.598844408820458085 ) ) ;
#12476=CARTESIAN_POINT ( 'NONE',  ( 98.15313185440925281, 81.25000000136560629, -4.458734125000016313 ) ) ;
#12477=CARTESIAN_POINT ( 'NONE',  ( 51.85481384221820633, 39.16445312608393436, 0.000000000000000000 ) ) ;
#12483=CARTESIAN_POINT ( 'NONE',  ( 143.1451861577818079, 32.36796875108393579, 5.444914386472293977 ) ) ;
#12484=EDGE_CURVE ( 'NONE', #20385, #9261, #3124, .T. ) ;
#12488=CARTESIAN_POINT ( 'NONE',  ( 103.1528011352953342, 80.81250000136559208, 3.152801135295355106 ) ) ;
#12490=CARTESIAN_POINT ( 'NONE',  ( 78.57481594606304043, 37.57695312716787583, -5.622872871577873077 ) ) ;
#12491=VECTOR ( 'NONE', #25455, 999.9999999999998863 ) ;
#12493=CARTESIAN_POINT ( 'NONE',  ( -5.622872871577873077, 35.69179687716786731, 13.57481594606304753 ) ) ;
#12494=VERTEX_POINT ( 'NONE', #15099 ) ;
#12496=ORIENTED_EDGE ( 'NONE', *, *, #24272, .T. ) ;
#12497=CARTESIAN_POINT ( 'NONE',  ( 204.2950502721270425, 36.28710937608393294, -9.295050272127046043 ) ) ;
#12498=CARTESIAN_POINT ( 'NONE',  ( -20.00000000000000000, 80.00000000000000000, 10.00000000000000000 ) ) ;
#12499=CARTESIAN_POINT ( 'NONE',  ( 139.2950502721270425, 38.46992187608393010, 9.295050272127046043 ) ) ;
#12503=DIRECTION ( 'NONE',  ( 0.000000000000000000, 0.000000000000000000, 1.000000000000000000 ) ) ;
#12505=CARTESIAN_POINT ( 'NONE',  ( 208.5748159460630688, 36.63437499999999858, -1.662435489736055892E-15 ) ) ;
#12509=CARTESIAN_POINT ( 'NONE',  ( 78.14518615778179367, 40.20625000108393010, -5.444914386472297529 ) ) ;
#12510=CIRCLE ( 'NONE', #26655, 5.000000000000000888 ) ;
#12514=CARTESIAN_POINT ( 'NONE',  ( 130.0000000000000000, 39.61093749999999147, 13.57481594606304576 ) ) ;
#12515=CARTESIAN_POINT ( 'NONE',  ( -5.622872871577873077, 39.26367187499999289, -13.57481594606304753 ) ) ;
#12517=CARTESIAN_POINT ( 'NONE',  ( 99.99999999999995737, 81.93750000136559208, 4.458734124999988779 ) ) ;
#12518=CIRCLE ( 'NONE', #20740, 5.000000000000000888 ) ;
#12521=ORIENTED_EDGE ( 'NONE', *, *, #11267, .T. ) ;
#12522=CARTESIAN_POINT ( 'NONE',  ( 204.5988444088204687, 37.42812500216787441, 9.598844408820456309 ) ) ;
#12525=CARTESIAN_POINT ( 'NONE',  ( 99.99999999999995737, 78.00000000000000000, -1.387778780781445676E-14 ) ) ;
#12531=CARTESIAN_POINT ( 'NONE',  ( 189.3771271284221314, 38.56914062716788294, -13.57481594606304753 ) ) ;
#12533=DIRECTION ( 'NONE',  ( 0.000000000000000000, 0.000000000000000000, 1.000000000000000000 ) ) ;
#12534=CARTESIAN_POINT ( 'NONE',  ( 196.5054921815576563, 53.60078691996476152, 14.99999999999994671 ) ) ;
#12535=CARTESIAN_POINT ( 'NONE',  ( 2.414731522848535132E-15, 36.18789062608393436, 13.14518615778179544 ) ) ;
#12536=CARTESIAN_POINT ( 'NONE',  ( -13.14518615778179189, 39.21406250108392300, 5.444914386472304635 ) ) ;
#12538=CARTESIAN_POINT ( 'NONE',  ( 51.42518405393695957, 39.36289062499999858, -5.622872871577873077 ) ) ;
#12540=CARTESIAN_POINT ( 'NONE',  ( 5.622872871577928144, 38.46992187716787726, -13.57481594606299247 ) ) ;
#12545=DIRECTION ( 'NONE',  ( 0.000000000000000000, 0.000000000000000000, -1.000000000000000000 ) ) ;
#12547=CARTESIAN_POINT ( 'NONE',  ( -9.295050272127044266, 38.46992187608393721, 9.295050272127047819 ) ) ;
#12548=CARTESIAN_POINT ( 'NONE',  ( 73.39221529163837943, 54.99999999999997158, 14.99999999999997158 ) ) ;
#12549=VERTEX_POINT ( 'NONE', #28102 ) ;
#12551=CIRCLE ( 'NONE', #299, 13.57481594606304398 ) ;
#12558=ORIENTED_EDGE ( 'NONE', *, *, #5141, .F. ) ;
#12559=CARTESIAN_POINT ( 'NONE',  ( 55.70494972787295751, 37.67617187608393436, 9.295050272127047819 ) ) ;
#12561=PLANE ( 'NONE',  #17581 ) ;
#12562=EDGE_LOOP ( 'NONE', ( #26114, #5542, #17197, #11380, #5060 ) ) ;
#12566=CARTESIAN_POINT ( 'NONE',  ( 143.5748159460630404, 35.89023437716787868, 5.622872871577869525 ) ) ;
#12569=CARTESIAN_POINT ( 'NONE',  ( 51.85481384221820633, 39.95820312608393010, 0.000000000000000000 ) ) ;
#12571=CARTESIAN_POINT ( 'NONE',  ( 189.5550856135277229, 37.42812500108394147, -13.14518615778179900 ) ) ;
#12572=ORIENTED_EDGE ( 'NONE', *, *, #23954, .F. ) ;
#12573=VERTEX_POINT ( 'NONE', #16973 ) ;
#12577=CARTESIAN_POINT ( 'NONE',  ( 99.99999999999995737, 85.00000000000000000, -5.000000000000018652 ) ) ;
#12581=DIRECTION ( 'NONE',  ( 0.000000000000000000, -1.000000000000000000, 0.000000000000000000 ) ) ;
#12582=CARTESIAN_POINT ( 'NONE',  ( 4.859977269581191806, 36.00000000000002132, 12.29462155906313292 ) ) ;
#12584=DIRECTION ( 'NONE',  ( -0.000000000000000000, 1.000000000000000000, -0.000000000000000000 ) ) ;
#12585=VERTEX_POINT ( 'NONE', #10690 ) ;
#12592=CARTESIAN_POINT ( 'NONE',  ( 143.1451861577818079, 40.40468750108393436, -5.444914386472297529 ) ) ;
#12593=CARTESIAN_POINT ( 'NONE',  ( 51.85481384221819923, 38.12265625108393152, -5.444914386472297529 ) ) ;
#12594=CARTESIAN_POINT ( 'NONE',  ( 208.1451861577817795, 40.30546875108393579, 5.444914386472293977 ) ) ;
#12596=CARTESIAN_POINT ( 'NONE',  ( 51.90409344636400846, 36.00000000000000000, 1.137167824541468031 ) ) ;
#12597=CARTESIAN_POINT ( 'NONE',  ( 13.14518615778179900, 37.03125000108393294, -5.444914386472297529 ) ) ;
#12598=CARTESIAN_POINT ( 'NONE',  ( 193.7288612287583476, 36.00000000000000711, -13.43002483374373135 ) ) ;
#12601=CARTESIAN_POINT ( 'NONE',  ( 116.4251840539369596, 40.15664062499999432, -5.622872871577872189 ) ) ;
#12603=CARTESIAN_POINT ( 'NONE',  ( -9.295050272127046043, 38.86679687608393863, -9.295050272127046043 ) ) ;
#12604=CARTESIAN_POINT ( 'NONE',  ( 1.501019124304962427, 53.60014735326989666, 15.00000000000000000 ) ) ;
#12606=EDGE_CURVE ( 'NONE', #3171, #4458, #25337, .T. ) ;
#12609=CARTESIAN_POINT ( 'NONE',  ( 181.9040934463640156, 36.00000000000000000, 1.137167824541468031 ) ) ;
#12612=CARTESIAN_POINT ( 'NONE',  ( 116.4251840539369596, 40.99999999999999289, 0.000000000000000000 ) ) ;
#12616=ADVANCED_FACE ( 'NONE', ( #23404 ), #6155, .T. ) ;
#12619=CARTESIAN_POINT ( 'NONE',  ( 103.1528011352953342, 80.06250000136559208, -3.152801135295383084 ) ) ;
#12620=CARTESIAN_POINT ( 'NONE',  ( 74.29505027212704249, 39.46210937608393721, 9.295050272127046043 ) ) ;
#12622=CARTESIAN_POINT ( 'NONE',  ( 9.295050272127046043, 40.25585937608393294, -9.295050272127046043 ) ) ;
#12625=CARTESIAN_POINT ( 'NONE',  ( 139.5988444088204403, 39.11484374999999858, -9.598844408820458085 ) ) ;
#12627=CARTESIAN_POINT ( 'NONE',  ( 116.8548138422182063, 31.97109375108393436, -5.444914386472297529 ) ) ;
#12631=CARTESIAN_POINT ( 'NONE',  ( 99.99999999999995737, 80.68750000136559208, 4.458734124999988779 ) ) ;
#12632=CARTESIAN_POINT ( 'NONE',  ( 130.0000000000000000, 39.95820312608393010, 13.14518615778179544 ) ) ;
#12633=CARTESIAN_POINT ( 'NONE',  ( 74.59884440882045453, 36.03906250216787299, -9.598844408820458085 ) ) ;
#12635=CARTESIAN_POINT ( 'NONE',  ( -13.57481594606304576, 35.59257812716788294, 5.622872871577880183 ) ) ;
#12639=DIRECTION ( 'NONE',  ( 0.000000000000000000, -1.000000000000000000, 0.000000000000000000 ) ) ;
#12642=CARTESIAN_POINT ( 'NONE',  ( 189.5550856135277229, 35.93984375108392726, 13.14518615778179722 ) ) ;
#12645=CARTESIAN_POINT ( 'NONE',  ( 130.0000000000000000, 39.16445312608392726, 13.14518615778179544 ) ) ;
#12646=LINE ( 'NONE', #16805, #14140 ) ;
#12647=LINE ( 'NONE', #13200, #25444 ) ;
#12649=DIRECTION ( 'NONE',  ( -0.000000000000000000, 1.000000000000000000, -0.000000000000000000 ) ) ;
#12650=B_SPLINE_CURVE_WITH_KNOTS ( 'NONE', 3,
 ( #22538, #18543, #14246, #3006, #20688, #737, #15822, #7703, #26677, #5581, #24528, #22968, #12097, #593, #17968, #11678, #25640, #3716, #10522, #16539, #14524, #1301, #12233, #1584, #27385 ),
 .UNSPECIFIED., .F., .F.,
 ( 4, 2, 2, 2, 2, 2, 2, 1, 2, 2, 2, 2, 4 ),
 ( 0.000000000000000000, 0.001301161269048871838, 0.002602322538097743675, 0.005204645076195476075, 0.007806967614293208041, 0.01040929015239094001, 0.01171045142143980686, 0.01301161269048867371, 0.01431277395953754229, 0.01561393522858640914, 0.01821625776668406999, 0.01951741903573289694, 0.02081858030478172389 ),
 .UNSPECIFIED. ) ;
#12652=CARTESIAN_POINT ( 'NONE',  ( 185.4011555911795597, 38.71796874999999716, 9.598844408820459861 ) ) ;
#12656=CARTESIAN_POINT ( 'NONE',  ( 51.85481384221820633, 38.96601562608393721, 0.000000000000000000 ) ) ;
#12658=PLANE ( 'NONE',  #25046 ) ;
#12660=CARTESIAN_POINT ( 'NONE',  ( 116.4251840539369596, 39.36289062499999858, -5.622872871577872189 ) ) ;
#12661=CARTESIAN_POINT ( 'NONE',  ( -13.57481594606304753, 40.95039062499999005, -5.622872871577873077 ) ) ;
#12666=CARTESIAN_POINT ( 'NONE',  ( 99.99999999999995737, 83.43750000136560629, -4.458734125000016313 ) ) ;
#12667=AXIS2_PLACEMENT_3D ( 'NONE', #1126, #21056, #1262 ) ;
#12671=CARTESIAN_POINT ( 'NONE',  ( 70.44491438647230552, 36.23750000108393721, 13.14518615778179189 ) ) ;
#12676=CARTESIAN_POINT ( 'NONE',  ( 97.92893218813452449, 81.93750000273118417, -5.000000000000043521 ) ) ;
#12678=CARTESIAN_POINT ( 'NONE',  ( 208.5748159460630120, 36.78320312716786589, -5.622872871577873077 ) ) ;
#12680=DIRECTION ( 'NONE',  ( -0.8660254037844407060, 0.4999999999999963363, 0.000000000000000000 ) ) ;
#12681=CARTESIAN_POINT ( 'NONE',  ( 200.3237909639438215, 54.47170356488064868, 14.99999999999994671 ) ) ;
#12682=CARTESIAN_POINT ( 'NONE',  ( 130.0000000000000000, 38.96601562608393721, -13.14518615778179544 ) ) ;
#12683=CARTESIAN_POINT ( 'NONE',  ( -9.295050272127044266, 37.67617187608393436, 9.295050272127047819 ) ) ;
#12684=ORIENTED_EDGE ( 'NONE', *, *, #14192, .T. ) ;
#12685=CARTESIAN_POINT ( 'NONE',  ( 78.57481594606305464, 36.63437499999999858, -1.662435489736055892E-15 ) ) ;
#12687=CIRCLE ( 'NONE', #19543, 5.000000000000004441 ) ;
#12689=CARTESIAN_POINT ( 'NONE',  ( 2.493653234604083739E-15, 36.43593749999999432, 13.57481594606304576 ) ) ;
#12695=CARTESIAN_POINT ( 'NONE',  ( -13.14518615778179544, 39.95820312608393010, 0.000000000000000000 ) ) ;
#12696=DIRECTION ( 'NONE',  ( -0.000000000000000000, 1.000000000000000000, -0.000000000000000000 ) ) ;
#12701=CARTESIAN_POINT ( 'NONE',  ( 99.99999999999995737, 83.37500000273119838, 4.999999999999990230 ) ) ;
#12702=CARTESIAN_POINT ( 'NONE',  ( -5.622872871577890841, 40.35507812499999147, 13.57481594606302444 ) ) ;
#12703=CARTESIAN_POINT ( 'NONE',  ( 195.0000000000000000, 39.56132812608393579, -13.14518615778179544 ) ) ;
#12705=CARTESIAN_POINT ( 'NONE',  ( 59.55508561352770158, 39.01562500108394005, -13.14518615778179722 ) ) ;
#12709=ORIENTED_EDGE ( 'NONE', *, *, #5162, .T. ) ;
#12711=CARTESIAN_POINT ( 'NONE',  ( -1.814355354584118674, 51.46618445021835697, -14.99999999999999467 ) ) ;
#12712=CARTESIAN_POINT ( 'NONE',  ( 97.92893218813455292, 80.93750000273118417, -5.000000000000053291 ) ) ;
#12714=CARTESIAN_POINT ( 'NONE',  ( 143.5748159460630404, 35.19570312716788152, -5.622872871577873077 ) ) ;
#12716=CARTESIAN_POINT ( 'NONE',  ( 181.8548138422181921, 35.14609375108393152, -5.444914386472297529 ) ) ;
#12721=CARTESIAN_POINT ( 'NONE',  ( 55.70494972787295751, 39.85898437608393152, 9.295050272127047819 ) ) ;
#12722=CARTESIAN_POINT ( 'NONE',  ( 99.99999999999995737, 80.68750000136559208, 4.458734124999988779 ) ) ;
#12724=VECTOR ( 'NONE', #564, 1000.000000000000000 ) ;
#12729=CARTESIAN_POINT ( 'NONE',  ( 181.8548138422182205, 39.95820312608393010, 0.000000000000000000 ) ) ;
#12731=ORIENTED_EDGE ( 'NONE', *, *, #22243, .F. ) ;
#12735=CARTESIAN_POINT ( 'NONE',  ( 143.1451861577818079, 36.33671875108394289, 5.444914386472293977 ) ) ;
#12736=CARTESIAN_POINT ( 'NONE',  ( 59.55508561352770158, 36.73359375108393010, 13.14518615778179722 ) ) ;
#12737=CARTESIAN_POINT ( 'NONE',  ( 195.0000000000000000, 40.55351562608393579, -13.14518615778179544 ) ) ;
#12738=( BOUNDED_CURVE ( )  B_SPLINE_CURVE ( 2, ( #9572, #26983, #1187, #27399, #9854, #27948, #1735, #28088, #2007 ),
 .UNSPECIFIED., .F., .T. ) 
 B_SPLINE_CURVE_WITH_KNOTS ( ( 3, 2, 2, 2, 3 ),
 ( 0.3958333333333331483, 0.4062499999999999445, 0.4166666666666667407, 0.4270833333333335369, 0.4375000000000003331 ),
 .UNSPECIFIED. ) 
 CURVE ( )  GEOMETRIC_REPRESENTATION_ITEM ( )  RATIONAL_B_SPLINE_CURVE ( ( 1.000000000000001110, 0.9238795325112855172, 1.000000000000000000, 0.9238795325112867385, 1.000000000000000000, 0.9238795325112867385, 1.000000000000000000, 0.9238795325112842960, 1.000000000000002442 ) ) 
 REPRESENTATION_ITEM ( '' )  );
#12740=CARTESIAN_POINT ( 'NONE',  ( -13.14518615778179544, 35.79101562608393294, 0.000000000000000000 ) ) ;
#12741=CARTESIAN_POINT ( 'NONE',  ( 127.7238531554433791, 51.46995505939418791, -15.00000000000033751 ) ) ;
#12745=CARTESIAN_POINT ( 'NONE',  ( 13.14518615778179900, 37.72578125108393721, 5.444914386472293977 ) ) ;
#12746=DIRECTION ( 'NONE',  ( -0.000000000000000000, -0.000000000000000000, -1.000000000000000000 ) ) ;
#12759=CARTESIAN_POINT ( 'NONE',  ( 104.4587341249999639, 81.93750000136559208, -1.442382525525748735E-14 ) ) ;
#12760=CARTESIAN_POINT ( 'NONE',  ( 78.14518615778179367, 37.92421875108392726, 5.444914386472293977 ) ) ;
#12762=CARTESIAN_POINT ( 'NONE',  ( 9.295050272127047819, 40.05742187608392868, 9.295050272127046043 ) ) ;
#12764=ADVANCED_FACE ( 'NONE', ( #9556 ), #13535, .F. ) ;
#12768=CARTESIAN_POINT ( 'NONE',  ( 130.0000000000000000, 39.61093749999999147, 13.57481594606304576 ) ) ;
#12769=EDGE_LOOP ( 'NONE', ( #9336, #16301, #20834, #26587 ) ) ;
#12771=ADVANCED_FACE ( 'NONE', ( #2448 ), #24382, .T. ) ;
#12773=CARTESIAN_POINT ( 'NONE',  ( 103.1528011352953342, 80.06250000136559208, -3.152801135295383084 ) ) ;
#12775=CARTESIAN_POINT ( 'NONE',  ( 139.2950502721270425, 37.87460937608393152, -9.295050272127046043 ) ) ;
#12776=CARTESIAN_POINT ( 'NONE',  ( 70.62287287157786864, 36.08867187716787583, -13.57481594606304753 ) ) ;
#12778=CARTESIAN_POINT ( 'NONE',  ( -9.598844408820454532, 36.43593750216787441, 9.598844408820459861 ) ) ;
#12782=CARTESIAN_POINT ( 'NONE',  ( 204.2950502721270425, 38.46992187608393010, 9.295050272127046043 ) ) ;
#12783=CARTESIAN_POINT ( 'NONE',  ( 65.00000000000000000, 39.21406249999999716, -13.57481594606304576 ) ) ;
#12784=CARTESIAN_POINT ( 'NONE',  ( 116.8548138422182205, 38.96601562608393721, 0.000000000000000000 ) ) ;
#12786=CYLINDRICAL_SURFACE ( 'NONE', #6315, 13.57481594606304398 ) ;
#12791=CARTESIAN_POINT ( 'NONE',  ( 185.4011555911795313, 36.93203124999999432, -9.598844408820458085 ) ) ;
#12795=CARTESIAN_POINT ( 'NONE',  ( 55.70494972787295751, 37.47773437608393010, 9.295050272127047819 ) ) ;
#12798=CARTESIAN_POINT ( 'NONE',  ( -13.57481594606304576, 40.25585937499999289, 5.622872871577880183 ) ) ;
#12799=CARTESIAN_POINT ( 'NONE',  ( 143.1451861577818079, 40.30546875108393579, 5.444914386472293977 ) ) ;
#12801=CARTESIAN_POINT ( 'NONE',  ( 99.99999999999995737, 84.25000000000000000, 4.999999999999990230 ) ) ;
#12803=ORIENTED_EDGE ( 'NONE', *, *, #11558, .F. ) ;
#12806=CARTESIAN_POINT ( 'NONE',  ( 55.70494972787295751, 33.70742187608393436, 9.295050272127047819 ) ) ;
#12808=CARTESIAN_POINT ( 'NONE',  ( 128.4989808756949969, 53.60014735326987534, -14.99999999999999822 ) ) ;
#12810=VERTEX_POINT ( 'NONE', #7124 ) ;
#12813=CARTESIAN_POINT ( 'NONE',  ( 208.5748159460630120, 37.47773437716787726, 5.622872871577869525 ) ) ;
#12818=CARTESIAN_POINT ( 'NONE',  ( 124.5550856135277087, 40.10703125108393152, 13.14518615778179722 ) ) ;
#12819=CARTESIAN_POINT ( 'NONE',  ( 13.14518615778179544, 38.76757812608393294, -1.609821015232357215E-15 ) ) ;
#12820=CARTESIAN_POINT ( 'NONE',  ( 143.1451861577818079, 34.65000000108393152, -5.444914386472297529 ) ) ;
#12821=CARTESIAN_POINT ( 'NONE',  ( 78.57481594606304043, 36.58476562499999574, 5.622872871577869525 ) ) ;
#12828=CARTESIAN_POINT ( 'NONE',  ( 214.9999999999999716, 55.00000000000000000, -10.00000000000000000 ) ) ;
#12838=CARTESIAN_POINT ( 'NONE',  ( 204.2950502721270425, 38.66835937608393436, -9.295050272127046043 ) ) ;
#12840=CYLINDRICAL_SURFACE ( 'NONE', #145, 11.57481594606304398 ) ;
#12842=CARTESIAN_POINT ( 'NONE',  ( 64.28023940389081758, 53.51499872091923038, -15.00000000000000000 ) ) ;
#12843=VERTEX_POINT ( 'NONE', #15821 ) ;
#12846=CARTESIAN_POINT ( 'NONE',  ( 130.0000000000000000, 33.75703125216787726, -13.57481594606304576 ) ) ;
#12848=CARTESIAN_POINT ( 'NONE',  ( 78.14518615778179367, 40.35507812608393863, -1.609821015232357215E-15 ) ) ;
#12850=CARTESIAN_POINT ( 'NONE',  ( 195.0000000000000000, 34.20351562608394147, -13.14518615778179544 ) ) ;
#12856=CARTESIAN_POINT ( 'NONE',  ( 104.4587341249999639, 80.93750000136559208, -1.442382525525748735E-14 ) ) ;
#12857=CARTESIAN_POINT ( 'NONE',  ( 185.7049497278729575, 39.85898437608393152, 9.295050272127047819 ) ) ;
#12858=CARTESIAN_POINT ( 'NONE',  ( 135.6228728715778971, 39.75976562716787299, 13.57481594606306174 ) ) ;
#12860=CARTESIAN_POINT ( 'NONE',  ( 214.9999999999999716, 55.00000000000000000, -10.00000000000000000 ) ) ;
#12863=ORIENTED_EDGE ( 'NONE', *, *, #2573, .F. ) ;
#12867=CARTESIAN_POINT ( 'NONE',  ( 124.5550856135277087, 35.04687500108393294, -13.14518615778179900 ) ) ;
#12868=CARTESIAN_POINT ( 'NONE',  ( 51.85481384221820633, 34.20351562608393436, 0.000000000000000000 ) ) ;
#12869=CARTESIAN_POINT ( 'NONE',  ( 181.8548138422181921, 37.62656250108393863, 5.444914386472304635 ) ) ;
#12871=CARTESIAN_POINT ( 'NONE',  ( 13.14518615778179900, 36.93203125108394147, 5.444914386472293977 ) ) ;
#12872=CARTESIAN_POINT ( 'NONE',  ( 138.7726092461284679, 50.37415326812335792, -15.00000000000000000 ) ) ;
#12877=CARTESIAN_POINT ( 'NONE',  ( -9.295050272127046043, 38.07304687608393579, -9.295050272127046043 ) ) ;
#12878=CARTESIAN_POINT ( 'NONE',  ( 5.317351577475893265, 54.47013368152371982, 15.00000000000000533 ) ) ;
#12881=VECTOR ( 'NONE', #3530, 1000.000000000000000 ) ;
#12887=CARTESIAN_POINT ( 'NONE',  ( 122.3637589320068884, 54.91786508990715276, 14.99999999999996625 ) ) ;
#12890=CARTESIAN_POINT ( 'NONE',  ( 103.1528011352953342, 81.06250000136559208, 3.152801135295355106 ) ) ;
#12891=CARTESIAN_POINT ( 'NONE',  ( 51.85481384221820633, 34.45156250108394147, 5.444914386472304635 ) ) ;
#12893=CARTESIAN_POINT ( 'NONE',  ( 5.444914386472297529, 39.51171875108393294, -13.14518615778179722 ) ) ;
#12898=CARTESIAN_POINT ( 'NONE',  ( 116.8548138422182063, 32.07031250108393294, 5.444914386472304635 ) ) ;
#12899=EDGE_LOOP ( 'NONE', ( #24726, #18322, #14360, #27684 ) ) ;
#12904=CARTESIAN_POINT ( 'NONE',  ( 135.4449143864723055, 35.24531250108393010, 13.14518615778179189 ) ) ;
#12905=CARTESIAN_POINT ( 'NONE',  ( 51.42518405393695957, 37.92421875216787441, 0.000000000000000000 ) ) ;
#12907=CARTESIAN_POINT ( 'NONE',  ( 5.622872871577871301, 36.08867187716787583, -13.57481594606304753 ) ) ;
#12910=VECTOR ( 'NONE', #22126, 1000.000000000000000 ) ;
#12911=CARTESIAN_POINT ( 'NONE',  ( 204.2950502721270425, 37.87460937608393152, -9.295050272127046043 ) ) ;
#12916=DIRECTION ( 'NONE',  ( 0.000000000000000000, 0.000000000000000000, 1.000000000000000000 ) ) ;
#12919=LINE ( 'NONE', #10234, #22561 ) ;
#12922=CARTESIAN_POINT ( 'NONE',  ( 208.5748159460630120, 34.30273437500000000, -5.622872871577873077 ) ) ;
#12925=CARTESIAN_POINT ( 'NONE',  ( 55.70494972787295751, 37.27929687608393294, -9.295050272127046043 ) ) ;
#12930=CARTESIAN_POINT ( 'NONE',  ( -13.57481594606304576, 37.03124999999999289, 0.000000000000000000 ) ) ;
#12932=ORIENTED_EDGE ( 'NONE', *, *, #6660, .F. ) ;
#12933=CARTESIAN_POINT ( 'NONE',  ( 104.4587341249999781, 80.12500000136560629, 1.846868145590721655 ) ) ;
#12934=AXIS2_PLACEMENT_3D ( 'NONE', #8266, #16954, #5626 ) ;
#12938=CARTESIAN_POINT ( 'NONE',  ( 51.85481384221820633, 34.40195312608393152, 0.000000000000000000 ) ) ;
#12940=CARTESIAN_POINT ( 'NONE',  ( 130.8421075954646540, 53.50112910130381749, -15.00000000000000000 ) ) ;
#12945=UNCERTAINTY_MEASURE_WITH_UNIT (LENGTH_MEASURE( 1.000000000000000082E-05 ), #13881, 'distance_accuracy_value', 'NONE');
#12946=CARTESIAN_POINT ( 'NONE',  ( 189.3771271284221314, 38.07304687716787583, 13.57481594606304753 ) ) ;
#12950=CARTESIAN_POINT ( 'NONE',  ( 191.8853022544570592, 53.90847045361017109, 14.99999999999995026 ) ) ;
#12951=CARTESIAN_POINT ( 'NONE',  ( 139.2950502721270425, 37.27929687608394005, -9.295050272127046043 ) ) ;
#12952=CARTESIAN_POINT ( 'NONE',  ( 5.444914386472297529, 38.12265625108393152, -13.14518615778179900 ) ) ;
#12954=CARTESIAN_POINT ( 'NONE',  ( 139.2950502721270425, 34.50117187608393010, 9.295050272127046043 ) ) ;
#12955=CARTESIAN_POINT ( 'NONE',  ( 78.57481594606304043, 33.40976562499999858, 5.622872871577869525 ) ) ;
#12959=CARTESIAN_POINT ( 'NONE',  ( 65.00000000000000000, -7.395377635281828788, -7.517135062566165128E-15 ) ) ;
#12962=CARTESIAN_POINT ( 'NONE',  ( 116.8548138422182205, 40.65273437608393436, 0.000000000000000000 ) ) ;
#12963=AXIS2_PLACEMENT_3D ( 'NONE', #7277, #894, #18117 ) ;
#12969=ORIENTED_EDGE ( 'NONE', *, *, #27913, .F. ) ;
#12972=CARTESIAN_POINT ( 'NONE',  ( 181.4251840539369596, 36.23749999999999005, 0.000000000000000000 ) ) ;
#12973=CARTESIAN_POINT ( 'NONE',  ( 200.4449143864723055, 37.62656250108393863, 13.14518615778179189 ) ) ;
#12982=CARTESIAN_POINT ( 'NONE',  ( 143.5748159460630404, 32.81445312716787299, -5.622872871577873077 ) ) ;
#12985=CARTESIAN_POINT ( 'NONE',  ( 208.1451861577818079, 35.59257812608393579, -1.609821015232357215E-15 ) ) ;
#12988=VERTEX_POINT ( 'NONE', #26102 ) ;
#12992=CARTESIAN_POINT ( 'NONE',  ( 104.4587341249999781, 80.00000000136560629, -1.846868145590750521 ) ) ;
#12993=CARTESIAN_POINT ( 'NONE',  ( 189.5550856135277229, 38.81718750108393579, -13.14518615778179722 ) ) ;
#12995=CARTESIAN_POINT ( 'NONE',  ( 187.3637589319962160, 54.91786508990981730, 14.99999999999995026 ) ) ;
#12997=CARTESIAN_POINT ( 'NONE',  ( 99.99999999999995737, 85.00000000000000000, -1.387778780781445676E-14 ) ) ;
#12998=CARTESIAN_POINT ( 'NONE',  ( 195.0000000000000000, -7.395377635281828788, -2.255140518769849538E-14 ) ) ;
#13004=CARTESIAN_POINT ( 'NONE',  ( 135.4449143864723055, 37.82500000108392868, 13.14518615778179189 ) ) ;
#13005=CARTESIAN_POINT ( 'NONE',  ( 78.14518615778179367, 32.21914062608393436, -1.609821015232357215E-15 ) ) ;
#13006=CARTESIAN_POINT ( 'NONE',  ( 189.5550856135277229, 37.72578125108395142, 13.14518615778179722 ) ) ;
#13009=( BOUNDED_CURVE ( )  B_SPLINE_CURVE ( 2, ( #10166, #18875, #2485, #23723, #24004, #24282, #11145, #6744, #26429, #13278, #19580, #6889, #2350, #6467, #12857, #6602, #28139, #17437, #15001, #64, #11291, #26136, #15286, #23859, #20012, #19441, #8606, #10870, #19861, #4763, #8746, #4481, #8466, #17154, #13137, #12993, #19718, #17294, #21873, #203, #25996, #11006, #15141, #8888, #9035, #348, #4337, #17578, #17727, #13423, #26284, #22008, #15429, #15574, #24143, #21733, #4620, #22149, #2630, #25856, #2207, #6327, #4198, #21586, #10732, #2062, #5333, #20582, #16290, #20440, #1065, #24992, #5472, #13998, #22723, #11434, #9450, #3189, #22294, #18149, #15996, #11573, #24713, #27149, #26863, #18006, #7309, #3047, #634, #11860, #3328, #5190, #13853 ),
 .UNSPECIFIED., .F., .T. ) 
 B_SPLINE_CURVE_WITH_KNOTS ( ( 3, 2, 2, 2, 2, 2, 2, 2, 2, 2, 2, 2, 2, 2, 2, 2, 2, 2, 2, 2, 2, 2, 2, 2, 2, 2, 2, 2, 2, 2, 2, 2, 2, 2, 2, 2, 2, 2, 2, 2, 2, 2, 2, 2, 2, 2, 3 ),
 ( 0.000000000000000000, 0.01041666666666666609, 0.02083333333333333218, 0.03125000000000000000, 0.04166666666666666435, 0.05208333333333333565, 0.06250000000000000000, 0.07291666666666667129, 0.08333333333333332871, 0.09374999999999998612, 0.1041666666666666713, 0.1145833333333333287, 0.1250000000000000000, 0.1354166666666666574, 0.1458333333333333426, 0.1562500000000000000, 0.1666666666666666574, 0.1770833333333333426, 0.1874999999999999722, 0.1979166666666666574, 0.2083333333333333426, 0.2187500000000000000, 0.2291666666666666574, 0.2395833333333333426, 0.2500000000000000000, 0.2604166666666666852, 0.2708333333333333148, 0.2812500000000000000, 0.2916666666666666852, 0.3020833333333333148, 0.3125000000000000000, 0.3229166666666666852, 0.3333333333333333148, 0.3437500000000000000, 0.3541666666666666852, 0.3645833333333333148, 0.3749999999999999445, 0.3854166666666666852, 0.3958333333333333148, 0.4062500000000000000, 0.4166666666666666852, 0.4270833333333333148, 0.4375000000000000000, 0.4479166666666666852, 0.4583333333333333148, 0.4687500000000000000, 0.4779971559588570562 ),
 .UNSPECIFIED. ) 
 CURVE ( )  GEOMETRIC_REPRESENTATION_ITEM ( )  RATIONAL_B_SPLINE_CURVE ( ( 1.000000000000000000, 0.9238795325112867385, 1.000000000000000000, 0.9238795325112867385, 1.000000000000000000, 0.9238795325112867385, 1.000000000000000000, 0.9238795325112867385, 1.000000000000000000, 0.9238795325112867385, 1.000000000000000000, 0.9238795325112867385, 1.000000000000000000, 0.9238795325112867385, 1.000000000000000000, 0.9238795325112867385, 1.000000000000000000, 0.9238795325112867385, 1.000000000000000000, 0.9238795325112867385, 1.000000000000000000, 0.9238795325112867385, 1.000000000000000000, 0.9238795325112867385, 1.000000000000000000, 0.9238795325112867385, 1.000000000000000000, 0.9238795325112867385, 1.000000000000000000, 0.9238795325112867385, 1.000000000000000000, 0.9238795325112867385, 1.000000000000000000, 0.9238795325112867385, 1.000000000000000000, 0.9238795325112867385, 1.000000000000000000, 0.9238795325112867385, 1.000000000000000000, 0.9238795325112867385, 1.000000000000000000, 0.9238795325112867385, 1.000000000000000000, 0.9238795325112867385, 1.000000000000000000, 0.9238795325112867385, 1.000000000000000000, 0.9238795325112867385, 1.000000000000000000, 0.9238795325112867385, 1.000000000000000000, 0.9238795325112867385, 1.000000000000000000, 0.9238795325112867385, 1.000000000000000000, 0.9238795325112867385, 1.000000000000000000, 0.9238795325112867385, 1.000000000000000000, 0.9238795325112867385, 1.000000000000000000, 0.9238795325112867385, 1.000000000000000000, 0.9238795325112867385, 1.000000000000000000, 0.9238795325112867385, 1.000000000000000000, 0.9238795325112867385, 1.000000000000000000, 0.9238795325112867385, 1.000000000000000000, 0.9238795325112867385, 1.000000000000000000, 0.9238795325112867385, 1.000000000000000000, 0.9238795325112867385, 1.000000000000000000, 0.9238795325112867385, 1.000000000000000000, 0.9238795325112867385, 1.000000000000000000, 0.9238795325112867385, 1.000000000000000000, 0.9238795325112867385, 1.000000000000000000, 0.9238795325112867385, 1.000000000000000000, 0.9238795325112867385, 1.000000000000000000, 0.9238795325112867385, 1.000000000000000000, 0.9324258078851931364, 0.9848264816800285093 ) ) 
 REPRESENTATION_ITEM ( '' )  );
#13010=CARTESIAN_POINT ( 'NONE',  ( 129.6713997234275269, 53.49358765998905341, -15.00000000000000000 ) ) ;
#13011=AXIS2_PLACEMENT_3D ( 'NONE', #21538, #27822, #12533 ) ;
#13013=CARTESIAN_POINT ( 'NONE',  ( 214.9999999999999716, 55.00000000000000000, 9.999999999999946709 ) ) ;
#13015=CARTESIAN_POINT ( 'NONE',  ( -9.295050272127044266, 35.09648437608392868, 9.295050272127047819 ) ) ;
#13020=CARTESIAN_POINT ( 'NONE',  ( 55.81982418635199394, 55.00000000000000711, 14.99999999999998224 ) ) ;
#13026=CARTESIAN_POINT ( 'NONE',  ( 128.3974668693900298, 53.60343507247939954, 14.99999999999996447 ) ) ;
#13029=CARTESIAN_POINT ( 'NONE',  ( 98.15313185440925281, 79.87500000136559208, 4.458734124999987891 ) ) ;
#13030=CARTESIAN_POINT ( 'NONE',  ( 55.70494972787295751, 34.50117187608393721, 9.295050272127047819 ) ) ;
#13032=DIRECTION ( 'NONE',  ( -0.000000000000000000, 1.000000000000000000, -0.000000000000000000 ) ) ;
#13033=AXIS2_PLACEMENT_3D ( 'NONE', #13386, #19974, #26244 ) ;
#13034=CARTESIAN_POINT ( 'NONE',  ( 104.9999999999999716, 80.56250000273119838, 2.071067811865462627 ) ) ;
#13037=CARTESIAN_POINT ( 'NONE',  ( 120.4011555911795455, 36.93203124999999432, -9.598844408820458085 ) ) ;
#13043=CARTESIAN_POINT ( 'NONE',  ( 143.1451861577818079, 36.13828125108393863, 5.444914386472293977 ) ) ;
#13045=CARTESIAN_POINT ( 'NONE',  ( 51.42518405393695957, 34.00507812716787015, 5.622872871577880183 ) ) ;
#13047=CARTESIAN_POINT ( 'NONE',  ( -5.622872871577873077, 31.42539062716787157, -13.57481594606304753 ) ) ;
#13049=CARTESIAN_POINT ( 'NONE',  ( 96.46446609406721961, 84.87500000000000000, -3.535533905932755072 ) ) ;
#13050=CARTESIAN_POINT ( 'NONE',  ( 181.8548138422182205, 34.20351562608393436, 0.000000000000000000 ) ) ;
#13052=CARTESIAN_POINT ( 'NONE',  ( 78.57481594606305464, 38.96601562499999005, 5.622872871577868636 ) ) ;
#13053=CARTESIAN_POINT ( 'NONE',  ( 104.9999999999999716, 81.56250000000002842, -2.071067811865491937 ) ) ;
#13054=CARTESIAN_POINT ( 'NONE',  ( 130.0000000000000000, -7.395377635281828788, -1.503427012513233026E-14 ) ) ;
#13055=CARTESIAN_POINT ( 'NONE',  ( 204.5988444088204687, 36.53515624999999289, 9.598844408820456309 ) ) ;
#13057=DIRECTION ( 'NONE',  ( -0.000000000000000000, 1.000000000000000000, -0.000000000000000000 ) ) ;
#13060=CARTESIAN_POINT ( 'NONE',  ( 185.4011555911795313, 36.13828124999999147, -9.598844408820458085 ) ) ;
#13061=CARTESIAN_POINT ( 'NONE',  ( 51.42518405393695957, 40.20624999999999005, 0.000000000000000000 ) ) ;
#13063=CARTESIAN_POINT ( 'NONE',  ( 74.29505027212704249, 36.08867187608392868, 9.295050272127046043 ) ) ;
#13069=CARTESIAN_POINT ( 'NONE',  ( -9.598844408820458085, 37.72578124999999005, -9.598844408820458085 ) ) ;
#13070=CARTESIAN_POINT ( 'NONE',  ( 130.0000000000000000, 37.77539062608393294, 13.14518615778179544 ) ) ;
#13071=ORIENTED_EDGE ( 'NONE', *, *, #1327, .F. ) ;
#13073=CARTESIAN_POINT ( 'NONE',  ( 98.15313185440925281, 80.50000000136560629, -4.458734125000016313 ) ) ;
#13076=CARTESIAN_POINT ( 'NONE',  ( 55.92190807730121094, 36.00000000000001421, -9.794392408849049048 ) ) ;
#13079=CARTESIAN_POINT ( 'NONE',  ( 59.55508561352770158, 35.84062500108394289, -13.14518615778179900 ) ) ;
#13081=CARTESIAN_POINT ( 'NONE',  ( 135.6228728715777549, 38.96601562716787015, 13.57481594606318076 ) ) ;
#13086=CARTESIAN_POINT ( 'NONE',  ( 200.6228728715778686, 38.96601562716787015, 13.57481594606304576 ) ) ;
#13088=LINE ( 'NONE', #15236, #1729 ) ;
#13089=CARTESIAN_POINT ( 'NONE',  ( 143.1451861577818079, 36.38632812608393863, -1.609821015232357215E-15 ) ) ;
#13090=CARTESIAN_POINT ( 'NONE',  ( -13.14518615778179189, 38.42031250108393436, 5.444914386472304635 ) ) ;
#13091=CARTESIAN_POINT ( 'NONE',  ( 120.7049497278729575, 35.89023437608393152, 9.295050272127047819 ) ) ;
#13092=CARTESIAN_POINT ( 'NONE',  ( 51.42518405393695957, 34.69960937499999432, 5.622872871577880183 ) ) ;
#13101=( BOUNDED_CURVE ( )  B_SPLINE_CURVE ( 2, ( #3768, #12429, #27711, #16865, #25563, #14711, #6586, #8590, #188 ),
 .UNSPECIFIED., .F., .F. ) 
 B_SPLINE_CURVE_WITH_KNOTS ( ( 3, 2, 2, 2, 3 ),
 ( 0.3125000000000002220, 0.3229166666666668517, 0.3333333333333334259, 0.3437500000000000555, 0.3541666666666666852 ),
 .UNSPECIFIED. ) 
 CURVE ( )  GEOMETRIC_REPRESENTATION_ITEM ( )  RATIONAL_B_SPLINE_CURVE ( ( 0.9999999999999983347, 0.9238795325112884038, 1.000000000000000000, 0.9238795325112867385, 1.000000000000000000, 0.9238795325112867385, 1.000000000000000000, 0.9238795325112867385, 1.000000000000000000 ) ) 
 REPRESENTATION_ITEM ( '' )  );
#13104=CARTESIAN_POINT ( 'NONE',  ( 5.444914386472297529, 35.74140625108393721, -13.14518615778179900 ) ) ;
#13108=FACE_OUTER_BOUND ( 'NONE', #14499, .T. ) ;
#13110=CARTESIAN_POINT ( 'NONE',  ( -8.312177448680279460E-16, 38.51953125216787299, -13.57481594606304576 ) ) ;
#13112=CARTESIAN_POINT ( 'NONE',  ( 208.1451861577817795, 40.10703125108393152, 5.444914386472293977 ) ) ;
#13113=ORIENTED_EDGE ( 'NONE', *, *, #24870, .T. ) ;
#13115=EDGE_CURVE ( 'NONE', #6189, #26410, #3214, .T. ) ;
#13116=CARTESIAN_POINT ( 'NONE',  ( 65.00000000000000000, -7.395377635281828788, -7.517135062566165128E-15 ) ) ;
#13123=ADVANCED_FACE ( 'NONE', ( #23932, #8393 ), #4268, .T. ) ;
#13124=CARTESIAN_POINT ( 'NONE',  ( 137.1713913950166557, 31.30502190640808990, -11.52591746582321974 ) ) ;
#13125=CARTESIAN_POINT ( 'NONE',  ( -5.444914386472299306, 40.10703125108393152, 13.14518615778179722 ) ) ;
#13128=CARTESIAN_POINT ( 'NONE',  ( 78.14518615778179367, 37.13046875108393863, 5.444914386472293977 ) ) ;
#13130=CARTESIAN_POINT ( 'NONE',  ( 204.2950502721270425, 35.69179687608394147, -9.295050272127046043 ) ) ;
#13131=VERTEX_POINT ( 'NONE', #14935 ) ;
#13132=ORIENTED_EDGE ( 'NONE', *, *, #14355, .T. ) ;
#13135=EDGE_CURVE ( 'NONE', #2438, #19624, #26409, .T. ) ;
#13136=CARTESIAN_POINT ( 'NONE',  ( 101.8468681455907046, 81.12500000136560629, -4.458734125000016313 ) ) ;
#13137=CARTESIAN_POINT ( 'NONE',  ( 185.7049497278729575, 38.86679687608393863, -9.295050272127046043 ) ) ;
#13139=CARTESIAN_POINT ( 'NONE',  ( 190.0749732163493206, 49.99999999893116609, 12.67776588292511519 ) ) ;
#13141=CIRCLE ( 'NONE', #11804, 4.999999999999997335 ) ;
#13142=CARTESIAN_POINT ( 'NONE',  ( -15.00000000000000355, 50.00000000000000000, -14.99999999999999822 ) ) ;
#13144=ORIENTED_EDGE ( 'NONE', *, *, #11012, .T. ) ;
#13145=ADVANCED_FACE ( 'NONE', ( #4132 ), #12658, .T. ) ;
#13149=CARTESIAN_POINT ( 'NONE',  ( 116.8548138422182205, 35.98945312608393721, 0.000000000000000000 ) ) ;
#13150=CARTESIAN_POINT ( 'NONE',  ( 51.85481384221819923, 34.15390625108393863, -5.444914386472297529 ) ) ;
#13152=CARTESIAN_POINT ( 'NONE',  ( 200.4449143864723055, 37.03125000108393294, 13.14518615778179189 ) ) ;
#13155=CARTESIAN_POINT ( 'NONE',  ( 2.414731522848535132E-15, 32.81445312608393294, 13.14518615778179544 ) ) ;
#13156=CARTESIAN_POINT ( 'NONE',  ( 181.9040934463640156, 36.00000000000000000, 1.137167824541468031 ) ) ;
#13157=FACE_OUTER_BOUND ( 'NONE', #13896, .T. ) ;
#13158=CARTESIAN_POINT ( 'NONE',  ( 78.57481594606305464, 40.55351562499999574, 5.622872871577868636 ) ) ;
#13160=CARTESIAN_POINT ( 'NONE',  ( -1.605271876576585877, 53.60388944777322706, 14.99999999999999645 ) ) ;
#13162=CARTESIAN_POINT ( 'NONE',  ( 57.36375893200157350, 54.91786508990982441, 14.99999999999998046 ) ) ;
#13168=CARTESIAN_POINT ( 'NONE',  ( 121.5976842187730966, 54.99999999484811752, 14.99999999999996625 ) ) ;
#13171=CARTESIAN_POINT ( 'NONE',  ( 104.4587341249999639, 82.18750000136559208, -1.442382525525748735E-14 ) ) ;
#13172=CARTESIAN_POINT ( 'NONE',  ( 51.85481384221820633, 36.83281250108393579, 5.444914386472304635 ) ) ;
#13174=CARTESIAN_POINT ( 'NONE',  ( 13.14518615778179722, 36.93203125108394147, 5.444914386472293977 ) ) ;
#13176=CARTESIAN_POINT ( 'NONE',  ( 120.4011555911795455, 36.13828124999999147, -9.598844408820458085 ) ) ;
#13178=CARTESIAN_POINT ( 'NONE',  ( 135.6228728715778686, 35.98945312499999716, -13.57481594606304753 ) ) ;
#13179=EDGE_CURVE ( 'NONE', #4960, #16430, #20224, .T. ) ;
#13185=CARTESIAN_POINT ( 'NONE',  ( 139.2950502721270425, 36.08867187608392868, 9.295050272127046043 ) ) ;
#13186=CARTESIAN_POINT ( 'NONE',  ( 70.62287287157788285, 33.40976562716787157, 13.57481594606304576 ) ) ;
#13187=AXIS2_PLACEMENT_3D ( 'NONE', #8256, #21516, #25784 ) ;
#13190=CARTESIAN_POINT ( 'NONE',  ( -8.312177448680279460E-16, 31.37578125216787583, -13.57481594606304576 ) ) ;
#13194=CARTESIAN_POINT ( 'NONE',  ( 195.0000000000000000, 33.60820312608392868, 13.14518615778179544 ) ) ;
#13196=B_SPLINE_CURVE_WITH_KNOTS ( 'NONE', 3,
 ( #12152, #9751, #23017, #6046, #18461, #12017, #21150, #3206, #5491, #8033, #25564, #16590, #1636, #1363, #7761, #18600, #3487, #10153 ),
 .UNSPECIFIED., .F., .F.,
 ( 4, 2, 2, 2, 2, 2, 2, 2, 4 ),
 ( 0.000000000000000000, 0.004618502246277095095, 0.006927753369415642209, 0.009237004492554190191, 0.01039163005412350495, 0.01154625561569281970, 0.01385550673883144401, 0.01616475786197007006, 0.01847400898510869610 ),
 .UNSPECIFIED. ) ;
#13198=CARTESIAN_POINT ( 'NONE',  ( 185.4011555911795313, 40.10703124999999147, -9.598844408820458085 ) ) ;
#13200=CARTESIAN_POINT ( 'NONE',  ( 95.27063293749995410, 79.28125000204838102, -1.387778780781445676E-14 ) ) ;
#13201=CARTESIAN_POINT ( 'NONE',  ( 136.0790800205188020, 54.65154858643460756, 14.99999999999996092 ) ) ;
#13203=FACE_OUTER_BOUND ( 'NONE', #15914, .T. ) ;
#13206=CARTESIAN_POINT ( 'NONE',  ( 204.5988444088204403, 35.93984374999999432, -9.598844408820458085 ) ) ;
#13208=CARTESIAN_POINT ( 'NONE',  ( 130.0000000000000000, 36.43593749999999432, 13.57481594606304576 ) ) ;
#13209=CARTESIAN_POINT ( 'NONE',  ( 65.00000000000000000, 34.00507812608393721, -13.14518615778179544 ) ) ;
#13212=DIRECTION ( 'NONE',  ( 1.000000000000000000, 0.000000000000000000, -2.385244779468110248E-16 ) ) ;
#13213=CARTESIAN_POINT ( 'NONE',  ( -5.622872871577873077, 37.18007812500000853, 13.57481594606304753 ) ) ;
#13214=CARTESIAN_POINT ( 'NONE',  ( 120.7049497278729575, 39.06523437608392868, -9.295050272127046043 ) ) ;
#13216=VERTEX_POINT ( 'NONE', #2973 ) ;
#13217=CARTESIAN_POINT ( 'NONE',  ( 97.92893218813451028, 83.81250000000001421, -5.000000000000018652 ) ) ;
#13219=CARTESIAN_POINT ( 'NONE',  ( 104.9999999999999574, 83.68750000273119838, -2.071067811865491937 ) ) ;
#13221=CARTESIAN_POINT ( 'NONE',  ( 66.46433772032058585, 36.00000000000002842, -13.46163418879030438 ) ) ;
#13223=CARTESIAN_POINT ( 'NONE',  ( 59.37712712842213136, 40.35507812499998437, 13.57481594606304753 ) ) ;
#13230=CARTESIAN_POINT ( 'NONE',  ( 185.4011555911795597, 35.64218750216787868, 9.598844408820459861 ) ) ;
#13234=CARTESIAN_POINT ( 'NONE',  ( 139.2950502721270425, 37.87460937608393863, 9.295050272127046043 ) ) ;
#13235=CARTESIAN_POINT ( 'NONE',  ( -13.14518615778179900, 35.93984375108393436, -5.444914386472297529 ) ) ;
#13237=CARTESIAN_POINT ( 'NONE',  ( 139.2950502721270425, 35.29492187608393294, 9.295050272127046043 ) ) ;
#13238=CARTESIAN_POINT ( 'NONE',  ( 74.59884440882045453, 34.15390624999999858, 9.598844408820456309 ) ) ;
#13241=CARTESIAN_POINT ( 'NONE',  ( 181.4251840539369596, 36.98164062499999005, -5.622872871577872189 ) ) ;
#13244=CARTESIAN_POINT ( 'NONE',  ( 2.493653234604083739E-15, 38.91640625216786731, 13.57481594606304576 ) ) ;
#13247=CARTESIAN_POINT ( 'NONE',  ( -9.295050272127044266, 35.29492187608393294, 9.295050272127047819 ) ) ;
#13253=CARTESIAN_POINT ( 'NONE',  ( 181.8548138422181921, 38.22187500108393010, 5.444914386472304635 ) ) ;
#13256=CARTESIAN_POINT ( 'NONE',  ( 204.1801758136479918, 55.00000000000000000, -15.00000000000000000 ) ) ;
#13262=CARTESIAN_POINT ( 'NONE',  ( 124.3771271284221314, 32.21914062716787441, -13.57481594606304753 ) ) ;
#13263=CARTESIAN_POINT ( 'NONE',  ( 9.295050272127047819, 40.25585937608393294, 9.295050272127046043 ) ) ;
#13266=CARTESIAN_POINT ( 'NONE',  ( 70.44491438647230552, 37.32890625108393579, -13.14518615778179900 ) ) ;
#13268=CARTESIAN_POINT ( 'NONE',  ( 74.18017581364799184, 55.00000000000000000, -15.00000000000000000 ) ) ;
#13269=CARTESIAN_POINT ( 'NONE',  ( 195.0000000000000000, 33.40976562608393863, -13.14518615778179544 ) ) ;
#13270=ADVANCED_FACE ( 'NONE', ( #9938 ), #7673, .F. ) ;
#13272=ORIENTED_EDGE ( 'NONE', *, *, #26943, .T. ) ;
#13277=CARTESIAN_POINT ( 'NONE',  ( 101.8468681455907046, 79.75000000136560629, 4.458734124999987891 ) ) ;
#13278=CARTESIAN_POINT ( 'NONE',  ( 208.1451861577818079, 40.10703125108393152, 5.444914386472293977 ) ) ;
#13280=CARTESIAN_POINT ( 'NONE',  ( 185.8198241863519797, 50.00000000000000000, 9.999999999999948486 ) ) ;
#13282=DIRECTION ( 'NONE',  ( -1.156482317317871478E-16, -0.000000000000000000, -1.000000000000000000 ) ) ;
#13290=CARTESIAN_POINT ( 'NONE',  ( 143.1451861577818079, 37.92421875108392726, 5.444914386472293977 ) ) ;
#13291=CARTESIAN_POINT ( 'NONE',  ( 55.70494972787295751, 34.10429687608393579, -9.295050272127046043 ) ) ;
#13292=VECTOR ( 'NONE', #5116, 1000.000000000000000 ) ;
#13293=CARTESIAN_POINT ( 'NONE',  ( 200.4449143864723055, 35.74140625108393721, -13.14518615778179900 ) ) ;
#13294=ORIENTED_EDGE ( 'NONE', *, *, #2215, .F. ) ;
#13295=CARTESIAN_POINT ( 'NONE',  ( 95.54126587499996504, 79.56250000136559208, -1.387778780781445676E-14 ) ) ;
#13296=CARTESIAN_POINT ( 'NONE',  ( 13.14518615778179900, 32.96328125108393436, 5.444914386472293977 ) ) ;
#13298=CARTESIAN_POINT ( 'NONE',  ( 125.1415007095402530, 49.99999999891476676, -12.70434618648937963 ) ) ;
#13299=DIRECTION ( 'NONE',  ( 1.000000000000000000, 0.000000000000000000, -1.156482317317871478E-16 ) ) ;
#13300=CARTESIAN_POINT ( 'NONE',  ( 195.0000000000000000, 50.00000000000000000, -2.255140518769849538E-14 ) ) ;
#13302=CARTESIAN_POINT ( 'NONE',  ( 199.1572863549628210, 35.99999999999999289, -12.92256159328821141 ) ) ;
#13305=CARTESIAN_POINT ( 'NONE',  ( 56.24166560764628997, 50.00000000000000000, 10.38725784494103799 ) ) ;
#13307=( LENGTH_UNIT ( ) NAMED_UNIT ( * ) SI_UNIT ( .MILLI., .METRE. ) );
#13317=CARTESIAN_POINT ( 'NONE',  ( 95.54126587499996504, 80.68750000136559208, -1.387778780781445676E-14 ) ) ;
#13318=CARTESIAN_POINT ( 'NONE',  ( 65.00000000000000000, 33.80664062608393294, 13.14518615778179544 ) ) ;
#13319=( BOUNDED_SURFACE ( )  B_SPLINE_SURFACE ( 1, 2, ( 
 ( #9331, #14022, #11880, #15880, #18174, #22318, #20604, #9473, #659, #26887, #13595, #16021, #24734, #26740, #5214, #15598, #24304, #13878, #13447, #3074, #4788, #22174, #20035, #515, #7043, #14303, #10445, #7626, #25289, #6053, #10029, #16872, #27173, #16318, #5917, #23021, #14717, #23160, #27719, #7765, #25569, #25148, #1368, #12021, #8180, #9894, #10299, #5774, #3636, #21155, #27579, #19006, #25018, #14584, #3775, #22885, #3910, #3494, #16735, #27309, #8038, #14445, #14166, #1641, #25434, #5638, #23435, #12571, #27437, #21298, #1780, #3351, #18605, #5497, #20883, #20745, #1230, #16595, #18739, #16452, #12156, #7901, #23302, #12299, #21024, #1504, #12433, #10158, #18869, #22001, #10860, #2476, #23996, #195, #19153, #25705, #4188, #4328, #23851, #6736, #8456, #21865, #13130, #23714, #12985, #27855, #17001, #17569, #4054, #19711, #8736, #6185, #17429, #12716, #17144, #14855, #2340, #4472, #8598, #17287, #6319, #8314, #1920, #10587, #21578, #10997, #15421, #19432, #2198, #14995, #8877, #25989, #12850, #19572, #27995, #21725, #15130, #2054, #6458, #26274, #24135, #10723, #23573, #57, #4611, #26128, #6594, #21441, #13269, #28131, #19295, #25845, #15276, #15852, #9166, #11283, #3428, #26707, #5580, #5043, #627, #20822, #17859, #9026, #17999, #24561, #20147, #23100, #20282, #15711, #9968, #7015, #1300, #25228, #2764, #13415, #20004, #12096, #9442, #485, #13707, #9302, #11428 ),
 ( #18681, #6879, #4903, #11137, #19852, #2620, #7156, #17719, #22427, #14383, #26420, #26563, #27383, #339, #22141, #16395, #5717, #2896, #7842, #11565, #24413, #15566, #25093, #768, #13565, #24274, #14245, #4755, #18142, #22288, #22966, #26855, #7702, #16536, #12376, #19364, #27655, #20959, #27519, #14653, #25924, #8388, #3845, #17074, #21234, #10236, #12652, #10378, #8533, #27793, #8115, #28067, #21094, #19227, #14931, #10100, #25371, #1990, #19085, #10656, #1583, #18812, #15067, #8250, #4126, #17219, #18946, #1717, #23372, #25638, #16810, #6398, #12231, #3575, #1442, #7975, #25508, #16674, #27928, #23237, #16938, #5852, #12791, #5987, #14522, #21377, #3714, #6121, #12505, #25779, #6257, #23651, #21510, #14787, #23510, #3989, #1855, #10520, #13060, #19508, #17794, #9099, #13206, #21940, #10935, #7089, #6529, #15208, #26204, #6953, #11357, #24068, #6811, #19645, #26496, #2417, #128, #15499, #4406, #270, #19788, #17503, #11076, #2697, #13498, #6667, #2129, #8956, #22218, #17645, #24211, #4262, #15648, #8813, #23785, #12922, #26352, #4690, #21797, #23927, #24346, #20080, #15352, #558, #21654, #10794, #2556, #4544, #9240, #13350, #4837, #2276, #17932, #22079, #11216, #8673, #26642, #19933, #17209, #415, #17365, #26061, #16216, #27213, #24492, #22790, #20649, #11500, #20787, #20364, #5401, #15922, #24917, #3118, #2832, #9801, #14070, #22501, #12062, #1268, #16068, #7668, #9932 ) ),
 .UNSPECIFIED., .F., .F., .F. ) 
 B_SPLINE_SURFACE_WITH_KNOTS ( ( 2, 2 ),
 ( 3, 2, 2, 2, 2, 2, 2, 2, 2, 2, 2, 2, 2, 2, 2, 2, 2, 2, 2, 2, 2, 2, 2, 2, 2, 2, 2, 2, 2, 2, 2, 2, 2, 2, 2, 2, 2, 2, 2, 2, 2, 2, 2, 2, 2, 2, 2, 2, 2, 2, 2, 2, 2, 2, 2, 2, 2, 2, 2, 2, 2, 2, 2, 2, 2, 2, 2, 2, 2, 2, 2, 2, 2, 2, 2, 2, 2, 2, 2, 2, 2, 2, 2, 2, 2, 2, 2, 2, 2, 2, 2, 3 ),
 ( 0.000000000000000000, 1.000000000000000000 ),
 ( 0.000000000000000000, 0.01041666666666666609, 0.02083333333333333218, 0.03125000000000000000, 0.04166666666666666435, 0.05208333333333333565, 0.06250000000000000000, 0.07291666666666667129, 0.08333333333333332871, 0.09375000000000000000, 0.1041666666666666713, 0.1145833333333333287, 0.1250000000000000000, 0.1354166666666666574, 0.1458333333333333426, 0.1562500000000000000, 0.1666666666666666574, 0.1770833333333333426, 0.1875000000000000000, 0.1979166666666666574, 0.2083333333333333426, 0.2187500000000000000, 0.2291666666666666574, 0.2395833333333333426, 0.2500000000000000000, 0.2604166666666666852, 0.2708333333333333148, 0.2812500000000000000, 0.2916666666666666852, 0.3020833333333333148, 0.3125000000000000000, 0.3229166666666666852, 0.3333333333333333148, 0.3437500000000000000, 0.3541666666666666852, 0.3645833333333333148, 0.3750000000000000000, 0.3854166666666666852, 0.3958333333333333148, 0.4062500000000000000, 0.4166666666666666852, 0.4270833333333333148, 0.4375000000000000000, 0.4479166666666666852, 0.4583333333333333148, 0.4687500000000000000, 0.4791666666666666852, 0.4895833333333333148, 0.5000000000000000000, 0.5104166666666666297, 0.5208333333333333703, 0.5312500000000000000, 0.5416666666666666297, 0.5520833333333333703, 0.5625000000000000000, 0.5729166666666666297, 0.5833333333333333703, 0.5937500000000000000, 0.6041666666666666297, 0.6145833333333333703, 0.6250000000000000000, 0.6354166666666666297, 0.6458333333333333703, 0.6562500000000000000, 0.6666666666666666297, 0.6770833333333333703, 0.6875000000000000000, 0.6979166666666666297, 0.7083333333333333703, 0.7187500000000000000, 0.7291666666666666297, 0.7395833333333333703, 0.7500000000000000000, 0.7604166666666666297, 0.7708333333333333703, 0.7812500000000000000, 0.7916666666666666297, 0.8020833333333333703, 0.8125000000000000000, 0.8229166666666666297, 0.8333333333333333703, 0.8437500000000000000, 0.8541666666666666297, 0.8645833333333333703, 0.8750000000000000000, 0.8854166666666666297, 0.8958333333333333703, 0.9062500000000000000, 0.9166666666666666297, 0.9270833333333333703, 0.9375000000000000000, 0.9448586968893691873 ),
 .UNSPECIFIED. ) 
 GEOMETRIC_REPRESENTATION_ITEM ( )  RATIONAL_B_SPLINE_SURFACE ( (
 ( 1.000000000000000000, 0.9238795325112867385, 1.000000000000000000, 0.9238795325112867385, 1.000000000000000000, 0.9238795325112867385, 1.000000000000000000, 0.9238795325112867385, 1.000000000000000000, 0.9238795325112867385, 1.000000000000000000, 0.9238795325112867385, 1.000000000000000000, 0.9238795325112867385, 1.000000000000000000, 0.9238795325112867385, 1.000000000000000000, 0.9238795325112867385, 1.000000000000000000, 0.9238795325112867385, 1.000000000000000000, 0.9238795325112867385, 1.000000000000000000, 0.9238795325112867385, 1.000000000000000000, 0.9238795325112867385, 1.000000000000000000, 0.9238795325112867385, 1.000000000000000000, 0.9238795325112867385, 1.000000000000000000, 0.9238795325112867385, 1.000000000000000000, 0.9238795325112867385, 1.000000000000000000, 0.9238795325112867385, 1.000000000000000000, 0.9238795325112867385, 1.000000000000000000, 0.9238795325112867385, 1.000000000000000000, 0.9238795325112867385, 1.000000000000000000, 0.9238795325112867385, 1.000000000000000000, 0.9238795325112867385, 1.000000000000000000, 0.9238795325112867385, 1.000000000000000000, 0.9238795325112867385, 1.000000000000000000, 0.9238795325112867385, 1.000000000000000000, 0.9238795325112867385, 1.000000000000000000, 0.9238795325112867385, 1.000000000000000000, 0.9238795325112867385, 1.000000000000000000, 0.9238795325112867385, 1.000000000000000000, 0.9238795325112867385, 1.000000000000000000, 0.9238795325112867385, 1.000000000000000000, 0.9238795325112867385, 1.000000000000000000, 0.9238795325112867385, 1.000000000000000000, 0.9238795325112867385, 1.000000000000000000, 0.9238795325112867385, 1.000000000000000000, 0.9238795325112867385, 1.000000000000000000, 0.9238795325112867385, 1.000000000000000000, 0.9238795325112867385, 1.000000000000000000, 0.9238795325112867385, 1.000000000000000000, 0.9238795325112867385, 1.000000000000000000, 0.9238795325112867385, 1.000000000000000000, 0.9238795325112867385, 1.000000000000000000, 0.9238795325112867385, 1.000000000000000000, 0.9238795325112867385, 1.000000000000000000, 0.9238795325112867385, 1.000000000000000000, 0.9238795325112867385, 1.000000000000000000, 0.9238795325112867385, 1.000000000000000000, 0.9238795325112867385, 1.000000000000000000, 0.9238795325112867385, 1.000000000000000000, 0.9238795325112867385, 1.000000000000000000, 0.9238795325112867385, 1.000000000000000000, 0.9238795325112867385, 1.000000000000000000, 0.9238795325112867385, 1.000000000000000000, 0.9238795325112867385, 1.000000000000000000, 0.9238795325112867385, 1.000000000000000000, 0.9238795325112867385, 1.000000000000000000, 0.9238795325112867385, 1.000000000000000000, 0.9238795325112867385, 1.000000000000000000, 0.9238795325112867385, 1.000000000000000000, 0.9238795325112867385, 1.000000000000000000, 0.9238795325112867385, 1.000000000000000000, 0.9238795325112867385, 1.000000000000000000, 0.9238795325112867385, 1.000000000000000000, 0.9238795325112867385, 1.000000000000000000, 0.9238795325112867385, 1.000000000000000000, 0.9238795325112867385, 1.000000000000000000, 0.9238795325112867385, 1.000000000000000000, 0.9238795325112867385, 1.000000000000000000, 0.9238795325112867385, 1.000000000000000000, 0.9238795325112867385, 1.000000000000000000, 0.9238795325112867385, 1.000000000000000000, 0.9238795325112867385, 1.000000000000000000, 0.9238795325112867385, 1.000000000000000000, 0.9238795325112867385, 1.000000000000000000, 0.9238795325112867385, 1.000000000000000000, 0.9238795325112867385, 1.000000000000000000, 0.9238795325112867385, 1.000000000000000000, 0.9238795325112867385, 1.000000000000000000, 0.9238795325112867385, 1.000000000000000000, 0.9238795325112867385, 1.000000000000000000, 0.9238795325112867385, 1.000000000000000000, 0.9238795325112867385, 1.000000000000000000, 0.9238795325112867385, 1.000000000000000000, 0.9238795325112867385, 1.000000000000000000, 0.9238795325112867385, 1.000000000000000000, 0.9238795325112867385, 1.000000000000000000, 0.9238795325112867385, 1.000000000000000000, 0.9238795325112867385, 1.000000000000000000, 0.9238795325112867385, 1.000000000000000000, 0.9462258450566536361, 0.9684275698016389100),
 ( 1.000000000000000000, 0.9238795325112867385, 1.000000000000000000, 0.9238795325112867385, 1.000000000000000000, 0.9238795325112867385, 1.000000000000000000, 0.9238795325112867385, 1.000000000000000000, 0.9238795325112867385, 1.000000000000000000, 0.9238795325112867385, 1.000000000000000000, 0.9238795325112867385, 1.000000000000000000, 0.9238795325112867385, 1.000000000000000000, 0.9238795325112867385, 1.000000000000000000, 0.9238795325112867385, 1.000000000000000000, 0.9238795325112867385, 1.000000000000000000, 0.9238795325112867385, 1.000000000000000000, 0.9238795325112867385, 1.000000000000000000, 0.9238795325112867385, 1.000000000000000000, 0.9238795325112867385, 1.000000000000000000, 0.9238795325112867385, 1.000000000000000000, 0.9238795325112867385, 1.000000000000000000, 0.9238795325112867385, 1.000000000000000000, 0.9238795325112867385, 1.000000000000000000, 0.9238795325112867385, 1.000000000000000000, 0.9238795325112867385, 1.000000000000000000, 0.9238795325112867385, 1.000000000000000000, 0.9238795325112867385, 1.000000000000000000, 0.9238795325112867385, 1.000000000000000000, 0.9238795325112867385, 1.000000000000000000, 0.9238795325112867385, 1.000000000000000000, 0.9238795325112867385, 1.000000000000000000, 0.9238795325112867385, 1.000000000000000000, 0.9238795325112867385, 1.000000000000000000, 0.9238795325112867385, 1.000000000000000000, 0.9238795325112867385, 1.000000000000000000, 0.9238795325112867385, 1.000000000000000000, 0.9238795325112867385, 1.000000000000000000, 0.9238795325112867385, 1.000000000000000000, 0.9238795325112867385, 1.000000000000000000, 0.9238795325112867385, 1.000000000000000000, 0.9238795325112867385, 1.000000000000000000, 0.9238795325112867385, 1.000000000000000000, 0.9238795325112867385, 1.000000000000000000, 0.9238795325112867385, 1.000000000000000000, 0.9238795325112867385, 1.000000000000000000, 0.9238795325112867385, 1.000000000000000000, 0.9238795325112867385, 1.000000000000000000, 0.9238795325112867385, 1.000000000000000000, 0.9238795325112867385, 1.000000000000000000, 0.9238795325112867385, 1.000000000000000000, 0.9238795325112867385, 1.000000000000000000, 0.9238795325112867385, 1.000000000000000000, 0.9238795325112867385, 1.000000000000000000, 0.9238795325112867385, 1.000000000000000000, 0.9238795325112867385, 1.000000000000000000, 0.9238795325112867385, 1.000000000000000000, 0.9238795325112867385, 1.000000000000000000, 0.9238795325112867385, 1.000000000000000000, 0.9238795325112867385, 1.000000000000000000, 0.9238795325112867385, 1.000000000000000000, 0.9238795325112867385, 1.000000000000000000, 0.9238795325112867385, 1.000000000000000000, 0.9238795325112867385, 1.000000000000000000, 0.9238795325112867385, 1.000000000000000000, 0.9238795325112867385, 1.000000000000000000, 0.9238795325112867385, 1.000000000000000000, 0.9238795325112867385, 1.000000000000000000, 0.9238795325112867385, 1.000000000000000000, 0.9238795325112867385, 1.000000000000000000, 0.9238795325112867385, 1.000000000000000000, 0.9238795325112867385, 1.000000000000000000, 0.9238795325112867385, 1.000000000000000000, 0.9238795325112867385, 1.000000000000000000, 0.9238795325112867385, 1.000000000000000000, 0.9238795325112867385, 1.000000000000000000, 0.9238795325112867385, 1.000000000000000000, 0.9238795325112867385, 1.000000000000000000, 0.9238795325112867385, 1.000000000000000000, 0.9238795325112867385, 1.000000000000000000, 0.9238795325112867385, 1.000000000000000000, 0.9238795325112867385, 1.000000000000000000, 0.9238795325112867385, 1.000000000000000000, 0.9238795325112867385, 1.000000000000000000, 0.9238795325112867385, 1.000000000000000000, 0.9238795325112867385, 1.000000000000000000, 0.9238795325112867385, 1.000000000000000000, 0.9238795325112867385, 1.000000000000000000, 0.9238795325112867385, 1.000000000000000000, 0.9238795325112867385, 1.000000000000000000, 0.9238795325112867385, 1.000000000000000000, 0.9238795325112867385, 1.000000000000000000, 0.9238795325112867385, 1.000000000000000000, 0.9238795325112867385, 1.000000000000000000, 0.9238795325112867385, 1.000000000000000000, 0.9462258450566536361, 0.9684275698016389100) ) ) 
 REPRESENTATION_ITEM ( '' )  SURFACE ( )  );
#13321=CARTESIAN_POINT ( 'NONE',  ( -13.14518615778179544, 38.17226562608393436, 0.000000000000000000 ) ) ;
#13325=CARTESIAN_POINT ( 'NONE',  ( 124.3771271284221314, 38.76757812500000000, 13.57481594606304753 ) ) ;
#13326=ORIENTED_EDGE ( 'NONE', *, *, #18902, .T. ) ;
#13329=DIRECTION ( 'NONE',  ( 0.000000000000000000, 0.000000000000000000, -1.000000000000000000 ) ) ;
#13333=CARTESIAN_POINT ( 'NONE',  ( 116.8548138422182063, 36.63437500108393152, 5.444914386472304635 ) ) ;
#13334=CARTESIAN_POINT ( 'NONE',  ( 74.59884440882045453, 35.04687500216787299, 9.598844408820456309 ) ) ;
#13335=ORIENTED_EDGE ( 'NONE', *, *, #26203, .T. ) ;
#13337=CARTESIAN_POINT ( 'NONE',  ( -8.312177448680279460E-16, 33.75703125216787726, -13.57481594606304576 ) ) ;
#13340=CARTESIAN_POINT ( 'NONE',  ( 181.8548138422181921, 35.84062500108394289, 5.444914386472304635 ) ) ;
#13341=CARTESIAN_POINT ( 'NONE',  ( 116.4251840539369596, 40.99999999999999289, 0.000000000000000000 ) ) ;
#13343=CYLINDRICAL_SURFACE ( 'NONE', #22819, 13.57481594606304398 ) ;
#13350=CARTESIAN_POINT ( 'NONE',  ( 200.6228728715778686, 33.60820312499998863, -13.57481594606304753 ) ) ;
#13351=EDGE_CURVE ( 'NONE', #27982, #12810, #13928, .T. ) ;
#13354=CARTESIAN_POINT ( 'NONE',  ( 51.85481384221819923, 34.94765625108392726, -5.444914386472297529 ) ) ;
#13357=ORIENTED_EDGE ( 'NONE', *, *, #16988, .T. ) ;
#13359=CARTESIAN_POINT ( 'NONE',  ( 5.622872871577878406, 34.89804687499999147, 13.57481594606304576 ) ) ;
#13360=CARTESIAN_POINT ( 'NONE',  ( 116.8548138422182063, 37.52734375108393294, -5.444914386472297529 ) ) ;
#13362=CARTESIAN_POINT ( 'NONE',  ( 104.4587341249999639, 80.18750000136559208, -1.442382525525748735E-14 ) ) ;
#13363=DIRECTION ( 'NONE',  ( 0.000000000000000000, 1.000000000000000000, 0.000000000000000000 ) ) ;
#13364=CARTESIAN_POINT ( 'NONE',  ( 104.9999999999999574, 81.56250000273119838, 2.071067811865462627 ) ) ;
#13366=CARTESIAN_POINT ( 'NONE',  ( 0.000000000000000000, -7.395377635281828788, 0.000000000000000000 ) ) ;
#13368=CARTESIAN_POINT ( 'NONE',  ( 78.57481594606304043, 39.75976562499999289, 5.622872871577869525 ) ) ;
#13369=ORIENTED_EDGE ( 'NONE', *, *, #16314, .F. ) ;
#13375=CARTESIAN_POINT ( 'NONE',  ( 208.5748159460630688, 35.93984375216787441, -1.662435489736055892E-15 ) ) ;
#13379=CARTESIAN_POINT ( 'NONE',  ( 195.0000000000000000, 38.51953125216787299, -13.57481594606304576 ) ) ;
#13381=CARTESIAN_POINT ( 'NONE',  ( 5.444914386472297529, 34.15390625108393863, -13.14518615778179900 ) ) ;
#13382=CARTESIAN_POINT ( 'NONE',  ( 116.8548138422182205, 34.20351562608393436, 0.000000000000000000 ) ) ;
#13383=CARTESIAN_POINT ( 'NONE',  ( 55.40115559117954547, 36.13828124999999147, -9.598844408820458085 ) ) ;
#13384=DIRECTION ( 'NONE',  ( 7.228014483236696740E-18, -0.000000000000000000, 1.000000000000000000 ) ) ;
#13386=CARTESIAN_POINT ( 'NONE',  ( -7.228014483236695816E-17, 75.00000000000000000, -9.999999999999998224 ) ) ;
#13391=CARTESIAN_POINT ( 'NONE',  ( 104.9999999999999716, 83.68750000273119838, -2.071067811865491937 ) ) ;
#13393=CARTESIAN_POINT ( 'NONE',  ( -5.444914386472297529, 35.84062500108394289, -13.14518615778179900 ) ) ;
#13398=LINE ( 'NONE', #2325, #12910 ) ;
#13399=EDGE_CURVE ( 'NONE', #15490, #291, #25339, .T. ) ;
#13400=CARTESIAN_POINT ( 'NONE',  ( 181.8548138422181921, 34.94765625108392726, -5.444914386472297529 ) ) ;
#13403=CARTESIAN_POINT ( 'NONE',  ( 59.68264842252411029, 54.47013368152370560, -15.00000000000000000 ) ) ;
#13409=CARTESIAN_POINT ( 'NONE',  ( 116.4251840539369454, 31.52460937716787370, -5.622872871577873077 ) ) ;
#13410=CYLINDRICAL_SURFACE ( 'NONE', #4347, 13.57481594606304398 ) ;
#13412=AXIS2_PLACEMENT_3D ( 'NONE', #19419, #4042, #28120 ) ;
#13413=CARTESIAN_POINT ( 'NONE',  ( 74.29505027212704249, 38.86679687608393863, -9.295050272127046043 ) ) ;
#13414=CARTESIAN_POINT ( 'NONE',  ( 58.91405578400244281, 54.65299103241780188, -15.00000000000000178 ) ) ;
#13415=CARTESIAN_POINT ( 'NONE',  ( 181.8548138422181921, 32.07031250108393294, 5.444914386472304635 ) ) ;
#13416=DIRECTION ( 'NONE',  ( 1.000000000000000000, 0.000000000000000000, -3.469446951953613696E-16 ) ) ;
#13418=VERTEX_POINT ( 'NONE', #18370 ) ;
#13421=CARTESIAN_POINT ( 'NONE',  ( 70.90850774719304184, 36.04503594658366694, 12.68159279706107334 ) ) ;
#13423=CARTESIAN_POINT ( 'NONE',  ( 181.8548138422182205, 38.12265625108393863, -5.444914386472297529 ) ) ;
#13426=AXIS2_PLACEMENT_3D ( 'NONE', #5898, #12277, #25683 ) ;
#13428=CARTESIAN_POINT ( 'NONE',  ( 208.1451861577818079, 39.51171875108393294, 5.444914386472293977 ) ) ;
#13433=AXIS2_PLACEMENT_3D ( 'NONE', #7418, #7565, #16259 ) ;
#13435=CARTESIAN_POINT ( 'NONE',  ( 139.2950502721270425, 32.51679687608393721, -9.295050272127046043 ) ) ;
#13436=CARTESIAN_POINT ( 'NONE',  ( 65.00000000000000000, 34.79882812608393294, -13.14518615778179544 ) ) ;
#13437=CARTESIAN_POINT ( 'NONE',  ( 195.0000000000000000, 36.58476562608393579, -13.14518615778179544 ) ) ;
#13443=CARTESIAN_POINT ( 'NONE',  ( 130.0000000000000000, 39.71015625216787015, 13.57481594606304576 ) ) ;
#13447=CARTESIAN_POINT ( 'NONE',  ( 185.7049497278729575, 39.85898437608393152, -9.295050272127046043 ) ) ;
#13448=ORIENTED_EDGE ( 'NONE', *, *, #7944, .F. ) ;
#13451=ORIENTED_EDGE ( 'NONE', *, *, #27456, .F. ) ;
#13454=CARTESIAN_POINT ( 'NONE',  ( 128.9858691739322865, 51.45790058219387220, 14.99999999999793765 ) ) ;
#13456=CARTESIAN_POINT ( 'NONE',  ( -5.622872871577816234, 38.56914062716787583, -13.57481594606310260 ) ) ;
#13457=CARTESIAN_POINT ( 'NONE',  ( 95.54126587499995082, 81.75000000136560629, 1.846868145590724986 ) ) ;
#13458=CARTESIAN_POINT ( 'NONE',  ( 74.29505027212704249, 36.48554687608393721, -9.295050272127046043 ) ) ;
#13460=CARTESIAN_POINT ( 'NONE',  ( 181.4251840539369596, 37.82499999999999574, 0.000000000000000000 ) ) ;
#13461=CARTESIAN_POINT ( 'NONE',  ( 9.295050272127047819, 39.26367187608393294, 9.295050272127046043 ) ) ;
#13462=DIRECTION ( 'NONE',  ( 0.000000000000000000, 0.000000000000000000, 1.000000000000000000 ) ) ;
#13463=DIRECTION ( 'NONE',  ( 0.000000000000000000, -1.000000000000000000, 0.000000000000000000 ) ) ;
#13464=CARTESIAN_POINT ( 'NONE',  ( 104.9999999999999716, 82.43750000000002842, 2.071067811865462627 ) ) ;
#13465=CARTESIAN_POINT ( 'NONE',  ( 135.6228728715778686, 36.78320312499999289, -13.57481594606304753 ) ) ;
#13466=ORIENTED_EDGE ( 'NONE', *, *, #8261, .F. ) ;
#13471=VECTOR ( 'NONE', #23678, 1000.000000000000000 ) ;
#13473=CARTESIAN_POINT ( 'NONE',  ( 139.2950502721270425, 33.90585937608393152, -9.295050272127046043 ) ) ;
#13475=CARTESIAN_POINT ( 'NONE',  ( 55.40115559117954547, 33.26093750216787726, 9.598844408820459861 ) ) ;
#13479=CARTESIAN_POINT ( 'NONE',  ( 13.57481594606304753, 32.02070312716787015, -5.622872871577873077 ) ) ;
#13484=CARTESIAN_POINT ( 'NONE',  ( 204.2950502721270425, 33.11210937608393579, -9.295050272127046043 ) ) ;
#13486=CARTESIAN_POINT ( 'NONE',  ( 203.7548989532324413, 50.00000000000000000, 10.39041163856606964 ) ) ;
#13488=CARTESIAN_POINT ( 'NONE',  ( 130.0000000000000000, 36.38632812608393152, -13.14518615778179544 ) ) ;
#13492=CARTESIAN_POINT ( 'NONE',  ( 200.6228728715777834, 36.48554687499999716, 13.57481594606309194 ) ) ;
#13495=AXIS2_PLACEMENT_3D ( 'NONE', #22540, #7705, #1303 ) ;
#13498=CARTESIAN_POINT ( 'NONE',  ( 195.0000000000000000, 34.84843749999999574, 13.57481594606304576 ) ) ;
#13500=CARTESIAN_POINT ( 'NONE',  ( 13.57481594606304753, 36.68398437500000142, -5.622872871577873966 ) ) ;
#13502=CARTESIAN_POINT ( 'NONE',  ( 55.70494972787295751, 36.48554687608393721, -9.295050272127046043 ) ) ;
#13505=VERTEX_POINT ( 'NONE', #4235 ) ;
#13507=CARTESIAN_POINT ( 'NONE',  ( -13.57481594606304753, 36.98164062499999005, -5.622872871577873077 ) ) ;
#13508=CARTESIAN_POINT ( 'NONE',  ( 143.1451861577818079, 38.71796875108393721, 5.444914386472293977 ) ) ;
#13511=CARTESIAN_POINT ( 'NONE',  ( 103.5355339059327093, 80.62500000000000000, -3.535533905932755072 ) ) ;
#13513=CARTESIAN_POINT ( 'NONE',  ( 94.99999999999995737, 80.18750000273121259, 2.071067811865466624 ) ) ;
#13515=CARTESIAN_POINT ( 'NONE',  ( 62.10793747869670511, 36.00000000000000000, -13.15766692561476958 ) ) ;
#13518=CARTESIAN_POINT ( 'NONE',  ( 51.85481384221820633, 32.07031250108393294, 5.444914386472304635 ) ) ;
#13522=ADVANCED_FACE ( 'NONE', ( #19199 ), #4376, .T. ) ;
#13524=ORIENTED_EDGE ( 'NONE', *, *, #11918, .T. ) ;
#13526=CARTESIAN_POINT ( 'NONE',  ( 204.5988444088204403, 34.45156250216787441, -9.598844408820458085 ) ) ;
#13530=CARTESIAN_POINT ( 'NONE',  ( 195.0000000000000000, 39.71015625216787015, 13.57481594606304576 ) ) ;
#13531=CARTESIAN_POINT ( 'NONE',  ( -9.295050272127044266, 33.70742187608393436, 9.295050272127047819 ) ) ;
#13533=CARTESIAN_POINT ( 'NONE',  ( 55.40115559117954547, 34.74921874999999716, 9.598844408820459861 ) ) ;
#13535=PLANE ( 'NONE',  #7768 ) ;
#13537=DIRECTION ( 'NONE',  ( 0.000000000000000000, 0.000000000000000000, -1.000000000000000000 ) ) ;
#13540=DIRECTION ( 'NONE',  ( 0.000000000000000000, 0.000000000000000000, -1.000000000000000000 ) ) ;
#13543=CARTESIAN_POINT ( 'NONE',  ( -8.049105076161786076E-16, 37.37851562608393863, -13.14518615778179544 ) ) ;
#13549=CARTESIAN_POINT ( 'NONE',  ( 181.8548138422182205, 35.79101562608393294, 0.000000000000000000 ) ) ;
#13550=EDGE_LOOP ( 'NONE', ( #805, #6008 ) ) ;
#13557=AXIS2_PLACEMENT_3D ( 'NONE', #20367, #9524, #11502 ) ;
#13558=CARTESIAN_POINT ( 'NONE',  ( 120.7049497278729575, 39.66054687608393436, -9.295050272127046043 ) ) ;
#13559=DIRECTION ( 'NONE',  ( -0.000000000000000000, 1.000000000000000000, -0.000000000000000000 ) ) ;
#13560=CARTESIAN_POINT ( 'NONE',  ( 2.414731522848535132E-15, 35.19570312608392726, 13.14518615778179544 ) ) ;
#13562=CARTESIAN_POINT ( 'NONE',  ( 55.70494972787295751, 38.46992187608393721, 9.295050272127047819 ) ) ;
#13563=CARTESIAN_POINT ( 'NONE',  ( 68.11469774553764012, 53.90847045361286405, -15.00000000000000000 ) ) ;
#13565=CARTESIAN_POINT ( 'NONE',  ( 208.5748159460630688, 39.80937499999999574, -1.662435489736055892E-15 ) ) ;
#13566=CARTESIAN_POINT ( 'NONE',  ( 72.06563498876006690, 36.00000000000002842, 11.21307450592250987 ) ) ;
#13569=CARTESIAN_POINT ( 'NONE',  ( 51.85481384221820633, 36.53515625108393294, -5.444914386472297529 ) ) ;
#13571=DIRECTION ( 'NONE',  ( -0.000000000000000000, -1.000000000000000000, -0.000000000000000000 ) ) ;
#13575=CARTESIAN_POINT ( 'NONE',  ( 189.5550856135277229, 38.51953125108393294, 13.14518615778179722 ) ) ;
#13577=AXIS2_PLACEMENT_3D ( 'NONE', #26324, #4661, #18479 ) ;
#13581=VECTOR ( 'NONE', #4121, 1000.000000000000000 ) ;
#13583=ORIENTED_EDGE ( 'NONE', *, *, #21548, .T. ) ;
#13584=CARTESIAN_POINT ( 'NONE',  ( 120.7049497278729575, 34.30273437608393294, -9.295050272127046043 ) ) ;
#13585=CARTESIAN_POINT ( 'NONE',  ( 78.14518615778179367, 40.35507812608393863, -1.609821015232357215E-15 ) ) ;
#13586=CARTESIAN_POINT ( 'NONE',  ( 185.7049497278729575, 35.09648437608393579, -9.295050272127046043 ) ) ;
#13589=CARTESIAN_POINT ( 'NONE',  ( 9.295050272127046043, 32.31835937608393294, -9.295050272127046043 ) ) ;
#13591=DIRECTION ( 'NONE',  ( 0.000000000000000000, 0.000000000000000000, 1.000000000000000000 ) ) ;
#13595=CARTESIAN_POINT ( 'NONE',  ( 204.2950502721270425, 40.25585937608393294, 9.295050272127046043 ) ) ;
#13596=ADVANCED_FACE ( 'NONE', ( #10908 ), #23346, .T. ) ;
#13599=ORIENTED_EDGE ( 'NONE', *, *, #20104, .F. ) ;
#13602=CARTESIAN_POINT ( 'NONE',  ( 134.5048870863210766, 51.44650206076644139, 15.00000000000063416 ) ) ;
#13606=CARTESIAN_POINT ( 'NONE',  ( 78.57481594606305464, 37.52734375216787299, -1.662435489736055892E-15 ) ) ;
#13608=DIRECTION ( 'NONE',  ( 0.000000000000000000, 0.000000000000000000, 1.000000000000000000 ) ) ;
#13609=CARTESIAN_POINT ( 'NONE',  ( 13.14518615778179544, 36.98164062608393010, -1.609821015232357215E-15 ) ) ;
#13611=CARTESIAN_POINT ( 'NONE',  ( -8.772609246135315786, 50.37415326814002725, 15.00000000000326317 ) ) ;
#13613=CARTESIAN_POINT ( 'NONE',  ( 130.0000000000000000, 37.62656249999999858, -13.57481594606304576 ) ) ;
#13614=EDGE_LOOP ( 'NONE', ( #27856, #13721, #6573, #1913 ) ) ;
#13620=CARTESIAN_POINT ( 'NONE',  ( 143.1451861577818079, 32.21914062608393436, -1.609821015232357215E-15 ) ) ;
#13621=CARTESIAN_POINT ( 'NONE',  ( 74.59884440882045453, 31.87187500216787228, 9.598844408820456309 ) ) ;
#13622=EDGE_LOOP ( 'NONE', ( #303, #24263, #26956, #11447, #4474, #23542, #7995, #13856, #7964, #1534 ) ) ;
#13623=CARTESIAN_POINT ( 'NONE',  ( 51.42518405393695957, 37.18007812716787441, 5.622872871577880183 ) ) ;
#13624=CARTESIAN_POINT ( 'NONE',  ( 2.493653234604083739E-15, 34.15390625216787157, 13.57481594606304576 ) ) ;
#13626=CARTESIAN_POINT ( 'NONE',  ( 51.42518405393695957, 37.87460937499999147, 5.622872871577880183 ) ) ;
#13627=CYLINDRICAL_SURFACE ( 'NONE', #25820, 5.000000000000000888 ) ;
#13629=CARTESIAN_POINT ( 'NONE',  ( 200.4449143864723055, 34.74921875108394431, -13.14518615778179900 ) ) ;
#13630=DIRECTION ( 'NONE',  ( 0.000000000000000000, -1.000000000000000000, 0.000000000000000000 ) ) ;
#13632=VECTOR ( 'NONE', #13958, 1000.000000000000000 ) ;
#13642=EDGE_CURVE ( 'NONE', #12810, #4709, #5118, .T. ) ;
#13645=CARTESIAN_POINT ( 'NONE',  ( 13.57481594606304576, 36.63437499999999858, -1.662435489736055892E-15 ) ) ;
#13646=CARTESIAN_POINT ( 'NONE',  ( 98.15313185440925281, 82.25000000136559208, -4.458734125000016313 ) ) ;
#13647=CARTESIAN_POINT ( 'NONE',  ( 70.44491438647230552, 34.45156250108393436, 13.14518615778179189 ) ) ;
#13648=EDGE_CURVE ( 'NONE', #18589, #10173, #15834, .T. ) ;
#13652=CARTESIAN_POINT ( 'NONE',  ( -13.57481594606304576, 33.06249999999999289, 0.000000000000000000 ) ) ;
#13653=CARTESIAN_POINT ( 'NONE',  ( 130.0000000000000000, 38.17226562608394147, -13.14518615778179544 ) ) ;
#13654=EDGE_LOOP ( 'NONE', ( #6579, #16496, #7691, #25448 ) ) ;
#13655=CARTESIAN_POINT ( 'NONE',  ( 104.9999999999999716, 81.50000000000000000, -1.449011120738813565E-14 ) ) ;
#13657=CARTESIAN_POINT ( 'NONE',  ( 102.0710678118654329, 83.81250000273119838, -5.000000000000018652 ) ) ;
#13659=CYLINDRICAL_SURFACE ( 'NONE', #27455, 13.57481594606304398 ) ;
#13662=CARTESIAN_POINT ( 'NONE',  ( 65.00000000000000000, 32.61601562608393579, -13.14518615778179544 ) ) ;
#13666=VERTEX_POINT ( 'NONE', #9628 ) ;
#13669=CARTESIAN_POINT ( 'NONE',  ( 204.5988444088204687, 35.84062500216786873, 9.598844408820456309 ) ) ;
#13673=CARTESIAN_POINT ( 'NONE',  ( 95.27063293749995410, 84.28125000204839523, -1.387778780781445676E-14 ) ) ;
#13674=CARTESIAN_POINT ( 'NONE',  ( -13.14518615778179544, 33.60820312608393579, 0.000000000000000000 ) ) ;
#13675=CARTESIAN_POINT ( 'NONE',  ( 116.8548138422182205, 32.61601562608393579, 0.000000000000000000 ) ) ;
#13676=CARTESIAN_POINT ( 'NONE',  ( 74.59884440882045453, 32.76484374999999716, -9.598844408820458085 ) ) ;
#13680=CARTESIAN_POINT ( 'NONE',  ( 208.4541126562309330, 35.99999999999997158, 0.6772748633551743946 ) ) ;
#13686=CARTESIAN_POINT ( 'NONE',  ( -13.14518615778179900, 34.35234375108393579, -5.444914386472297529 ) ) ;
#13687=EDGE_CURVE ( 'NONE', #25435, #28031, #19501, .T. ) ;
#13688=ORIENTED_EDGE ( 'NONE', *, *, #14517, .T. ) ;
#13689=CARTESIAN_POINT ( 'NONE',  ( 130.0000000000000000, 36.83281249999999574, -13.57481594606304576 ) ) ;
#13690=LINE ( 'NONE', #13827, #18862 ) ;
#13691=CARTESIAN_POINT ( 'NONE',  ( -13.57481594606304576, 36.23749999999999005, 0.000000000000000000 ) ) ;
#13693=CARTESIAN_POINT ( 'NONE',  ( 208.1451861577817795, 37.03125000108393294, -5.444914386472297529 ) ) ;
#13694=ORIENTED_EDGE ( 'NONE', *, *, #24287, .T. ) ;
#13695=CARTESIAN_POINT ( 'NONE',  ( 193.1124712741235783, 53.66306546785489218, -14.99999999999999645 ) ) ;
#13700=FACE_OUTER_BOUND ( 'NONE', #25790, .T. ) ;
#13701=CARTESIAN_POINT ( 'NONE',  ( 135.4449143864723055, 37.92421875108392726, -13.14518615778179900 ) ) ;
#13702=LINE ( 'NONE', #4895, #27573 ) ;
#13703=CARTESIAN_POINT ( 'NONE',  ( 2.414731522848535132E-15, 36.78320312608393294, 13.14518615778179544 ) ) ;
#13705=CARTESIAN_POINT ( 'NONE',  ( 64.67139972343294119, 53.49358765998906051, -15.00000000000000000 ) ) ;
#13707=CARTESIAN_POINT ( 'NONE',  ( 195.0000000000000000, 31.82226562608393650, -13.14518615778179544 ) ) ;
#13709=ORIENTED_EDGE ( 'NONE', *, *, #18597, .F. ) ;
#13712=CARTESIAN_POINT ( 'NONE',  ( 74.29505027212704249, 38.46992187608393010, 9.295050272127046043 ) ) ;
#13719=CARTESIAN_POINT ( 'NONE',  ( 204.2950502721270425, 39.46210937608393721, 9.295050272127046043 ) ) ;
#13721=ORIENTED_EDGE ( 'NONE', *, *, #3383, .F. ) ;
#13724=VERTEX_POINT ( 'NONE', #16181 ) ;
#13725=CARTESIAN_POINT ( 'NONE',  ( 124.5550856135277087, 32.96328125108393436, 13.14518615778179722 ) ) ;
#13726=CARTESIAN_POINT ( 'NONE',  ( 51.85481384221820633, 31.87187500108393223, 5.444914386472304635 ) ) ;
#13727=CARTESIAN_POINT ( 'NONE',  ( 195.0000000000000000, 32.61601562608393579, -13.14518615778179544 ) ) ;
#13732=CARTESIAN_POINT ( 'NONE',  ( 116.4251840539369596, 37.97382812716787726, 5.622872871577880183 ) ) ;
#13736=CARTESIAN_POINT ( 'NONE',  ( 68.63649624680374473, 51.46815297079189833, 14.99999999999998401 ) ) ;
#13739=VERTEX_POINT ( 'NONE', #16606 ) ;
#13742=CARTESIAN_POINT ( 'NONE',  ( 136.8735082435767083, 51.14166184781144864, 15.00000000000258638 ) ) ;
#13745=CARTESIAN_POINT ( 'NONE',  ( 78.14518615778179367, 32.46718750108393436, -5.444914386472297529 ) ) ;
#13748=CARTESIAN_POINT ( 'NONE',  ( -9.295050272127044266, 38.27148437608393294, 9.295050272127047819 ) ) ;
#13749=LINE ( 'NONE', #25029, #3013 ) ;
#13751=DIRECTION ( 'NONE',  ( 0.000000000000000000, 0.000000000000000000, -1.000000000000000000 ) ) ;
#13752=CARTESIAN_POINT ( 'NONE',  ( 124.3771271284221314, 34.00507812499999716, 13.57481594606304753 ) ) ;
#13754=FACE_BOUND ( 'NONE', #10567, .T. ) ;
#13758=CARTESIAN_POINT ( 'NONE',  ( 143.1451861577818079, 34.65000000108393152, -5.444914386472297529 ) ) ;
#13760=CARTESIAN_POINT ( 'NONE',  ( 78.14518615778179367, 40.20625000108393010, -5.444914386472297529 ) ) ;
#13761=EDGE_CURVE ( 'NONE', #16261, #21367, #20435, .T. ) ;
#13762=CARTESIAN_POINT ( 'NONE',  ( 65.00000000000000000, 52.00000000000000711, -7.517135062566165128E-15 ) ) ;
#13763=CARTESIAN_POINT ( 'NONE',  ( 13.14518615778179900, 37.72578125108393721, 5.444914386472293977 ) ) ;
#13767=CARTESIAN_POINT ( 'NONE',  ( -5.444914386472297529, 40.40468750108393436, -13.14518615778179900 ) ) ;
#13768=FACE_OUTER_BOUND ( 'NONE', #18178, .T. ) ;
#13782=CARTESIAN_POINT ( 'NONE',  ( 95.54126587499996504, 82.43750000136559208, -1.387778780781445676E-14 ) ) ;
#13783=CARTESIAN_POINT ( 'NONE',  ( 55.70494972787295751, 31.72304687608393081, -9.295050272127046043 ) ) ;
#13789=CARTESIAN_POINT ( 'NONE',  ( 7.171391216998965312, 31.99955315621561525, -11.52591757658528948 ) ) ;
#13790=CARTESIAN_POINT ( 'NONE',  ( 135.4449143864723055, 35.74140625108393721, -13.14518615778179900 ) ) ;
#13791=ORIENTED_EDGE ( 'NONE', *, *, #27439, .F. ) ;
#13792=CARTESIAN_POINT ( 'NONE',  ( 102.0710678118654329, 81.31250000000000000, 4.999999999999989342 ) ) ;
#13794=CARTESIAN_POINT ( 'NONE',  ( 96.46446609406721961, 80.00000000273119838, -3.535533905932755072 ) ) ;
#13796=CARTESIAN_POINT ( 'NONE',  ( 78.57481594606305464, 39.11484375216787157, -1.662435489736055892E-15 ) ) ;
#13798=CARTESIAN_POINT ( 'NONE',  ( 70.44491438647230552, 32.56640625108394005, -13.14518615778179900 ) ) ;
#13799=CARTESIAN_POINT ( 'NONE',  ( 59.55508561352770158, 36.13828125108393152, 13.14518615778179722 ) ) ;
#13800=ORIENTED_EDGE ( 'NONE', *, *, #3260, .T. ) ;
#13801=CARTESIAN_POINT ( 'NONE',  ( 130.0000000000000000, -7.395377635281828788, -1.503427012513233026E-14 ) ) ;
#13803=EDGE_CURVE ( 'NONE', #5516, #19665, #23344, .T. ) ;
#13806=CARTESIAN_POINT ( 'NONE',  ( 195.0000000000000000, 33.36015625216786873, 13.57481594606304576 ) ) ;
#13807=ORIENTED_EDGE ( 'NONE', *, *, #22040, .T. ) ;
#13811=CARTESIAN_POINT ( 'NONE',  ( -9.295050272127046043, 36.68398437608393436, -9.295050272127046043 ) ) ;
#13820=DIRECTION ( 'NONE',  ( 0.000000000000000000, 0.000000000000000000, 1.000000000000000000 ) ) ;
#13822=CARTESIAN_POINT ( 'NONE',  ( 195.0000000000000000, 50.00000000000000000, -2.255140518769849538E-14 ) ) ;
#13823=CARTESIAN_POINT ( 'NONE',  ( -8.049105076161786076E-16, 31.82226562608393650, -13.14518615778179544 ) ) ;
#13827=CARTESIAN_POINT ( 'NONE',  ( -9.396418828207704684E-17, 78.00000000000000000, -12.99999999999999822 ) ) ;
#13829=CARTESIAN_POINT ( 'NONE',  ( 185.7049497278729575, 37.27929687608393294, -9.295050272127046043 ) ) ;
#13830=ORIENTED_EDGE ( 'NONE', *, *, #16950, .T. ) ;
#13832=CARTESIAN_POINT ( 'NONE',  ( 201.1165602397168186, 54.66944451632673463, -15.00000000000000178 ) ) ;
#13838=CYLINDRICAL_SURFACE ( 'NONE', #25786, 13.57481594606304398 ) ;
#13839=EDGE_CURVE ( 'NONE', #18823, #18668, #3783, .T. ) ;
#13840=CARTESIAN_POINT ( 'NONE',  ( 143.1451861577818079, 38.51953125108393294, 5.444914386472293977 ) ) ;
#13841=CARTESIAN_POINT ( 'NONE',  ( -13.14518615778179189, 36.83281250108393579, 5.444914386472304635 ) ) ;
#13842=CARTESIAN_POINT ( 'NONE',  ( 5.444914386472297529, 36.33671875108394289, -13.14518615778179900 ) ) ;
#13843=AXIS2_PLACEMENT_3D ( 'NONE', #12009, #4142, #22733 ) ;
#13845=CARTESIAN_POINT ( 'NONE',  ( -13.57481594606304753, 36.28710937716787299, -5.622872871577872189 ) ) ;
#13848=CARTESIAN_POINT ( 'NONE',  ( 77.66784425494549282, 35.99999999999997868, 4.396229039744254941 ) ) ;
#13851=CARTESIAN_POINT ( 'NONE',  ( 65.00000000000000000, 38.37070312608393152, 13.14518615778179544 ) ) ;
#13853=CARTESIAN_POINT ( 'NONE',  ( 196.1371678245420753, 35.99999999999999289, 13.09590655363592582 ) ) ;
#13854=ORIENTED_EDGE ( 'NONE', *, *, #7706, .T. ) ;
#13856=ORIENTED_EDGE ( 'NONE', *, *, #24116, .F. ) ;
#13859=CARTESIAN_POINT ( 'NONE',  ( 181.8548138422182205, 36.83281250108393579, 5.444914386472304635 ) ) ;
#13861=ORIENTED_EDGE ( 'NONE', *, *, #21226, .F. ) ;
#13866=CARTESIAN_POINT ( 'NONE',  ( 139.2950502721270425, 34.69960937608393436, 9.295050272127046043 ) ) ;
#13867=CARTESIAN_POINT ( 'NONE',  ( 78.14518615778180788, 40.40468750108393436, -5.444914386472297529 ) ) ;
#13868=CARTESIAN_POINT ( 'NONE',  ( 181.8548138422182205, 33.60820312608393579, 0.000000000000000000 ) ) ;
#13869=VERTEX_POINT ( 'NONE', #6470 ) ;
#13871=CARTESIAN_POINT ( 'NONE',  ( -0.8765262653614457333, 51.45968077934941221, -14.99999999999999289 ) ) ;
#13872=LINE ( 'NONE', #9326, #19972 ) ;
#13874=CARTESIAN_POINT ( 'NONE',  ( 143.5748159460630404, 39.16445312716788152, -5.622872871577873077 ) ) ;
#13876=CYLINDRICAL_SURFACE ( 'NONE', #26996, 13.57481594606304398 ) ;
#13878=CARTESIAN_POINT ( 'NONE',  ( 181.8548138422181921, 39.90859375108394147, -5.444914386472297529 ) ) ;
#13879=CIRCLE ( 'NONE', #13426, 13.57481594606304398 ) ;
#13881=( LENGTH_UNIT ( ) NAMED_UNIT ( * ) SI_UNIT ( .MILLI., .METRE. ) );
#13886=CARTESIAN_POINT ( 'NONE',  ( 133.8030543732469653, 54.09082899096448926, 14.99999999999996447 ) ) ;
#13887=CARTESIAN_POINT ( 'NONE',  ( -7.068365687998699798, 35.99999999999997158, 11.09140360074105658 ) ) ;
#13888=CARTESIAN_POINT ( 'NONE',  ( 51.85481384221820633, 32.86406250108393579, 5.444914386472304635 ) ) ;
#13889=DIRECTION ( 'NONE',  ( 1.156482317317871478E-16, 0.000000000000000000, 1.000000000000000000 ) ) ;
#13890=DIRECTION ( 'NONE',  ( -1.000000000000000000, 0.000000000000000000, 0.000000000000000000 ) ) ;
#13892=CYLINDRICAL_SURFACE ( 'NONE', #20303, 13.57481594606304398 ) ;
#13893=CARTESIAN_POINT ( 'NONE',  ( -8.758334392354218068, 50.00000000000000000, 10.38725784494356930 ) ) ;
#13894=CARTESIAN_POINT ( 'NONE',  ( 143.5748159460630688, 40.65273437499999432, -5.622872871577873966 ) ) ;
#13895=CARTESIAN_POINT ( 'NONE',  ( 130.0000000000000000, 35.64218749999999147, 13.57481594606304576 ) ) ;
#13896=EDGE_LOOP ( 'NONE', ( #17959, #6972, #13709, #1795 ) ) ;
#13897=ORIENTED_EDGE ( 'NONE', *, *, #11067, .F. ) ;
#13898=DIRECTION ( 'NONE',  ( 1.000000000000000000, 0.000000000000000000, -1.156482317317871725E-16 ) ) ;
#13902=CARTESIAN_POINT ( 'NONE',  ( 124.5550856135277087, 32.46718750108393436, -13.14518615778179900 ) ) ;
#13903=CARTESIAN_POINT ( 'NONE',  ( 55.70494972787295751, 39.66054687608393436, -9.295050272127046043 ) ) ;
#13904=CARTESIAN_POINT ( 'NONE',  ( 102.0710678118654897, 80.68750000000002842, -4.999999999999968914 ) ) ;
#13905=CARTESIAN_POINT ( 'NONE',  ( -13.14518615778179189, 39.01562500108393294, 5.444914386472304635 ) ) ;
#13910=CARTESIAN_POINT ( 'NONE',  ( 185.7049497278729575, 32.71523437608393436, 9.295050272127047819 ) ) ;
#13915=CARTESIAN_POINT ( 'NONE',  ( 132.0072970100684984, 35.99999999999997158, -13.40042260803736696 ) ) ;
#13916=CARTESIAN_POINT ( 'NONE',  ( 124.3771271284222877, 36.18789062716787441, -13.57481594606318254 ) ) ;
#13924=CARTESIAN_POINT ( 'NONE',  ( 99.99999999999995737, 83.18750000136560629, -4.458734125000016313 ) ) ;
#13925=CARTESIAN_POINT ( 'NONE',  ( 51.85481384221820633, 40.75195312608393294, 0.000000000000000000 ) ) ;
#13928=LINE ( 'NONE', #18786, #9574 ) ;
#13929=AXIS2_PLACEMENT_3D ( 'NONE', #7734, #16284, #27550 ) ;
#13931=CARTESIAN_POINT ( 'NONE',  ( -13.57481594606304753, 33.80664062500000000, -5.622872871577873077 ) ) ;
#13932=CARTESIAN_POINT ( 'NONE',  ( 120.7049497278729575, 33.70742187608393436, 9.295050272127047819 ) ) ;
#13933=VERTEX_POINT ( 'NONE', #8048 ) ;
#13936=CARTESIAN_POINT ( 'NONE',  ( 94.99999999999995737, 80.12500000273119838, -1.387778780781445676E-14 ) ) ;
#13939=CARTESIAN_POINT ( 'NONE',  ( 70.62287287157786864, 39.26367187716787299, -13.57481594606304753 ) ) ;
#13941=CARTESIAN_POINT ( 'NONE',  ( 200.4449143864723055, 40.20625000108394431, 13.14518615778179189 ) ) ;
#13942=CARTESIAN_POINT ( 'NONE',  ( 9.598844408820456309, 38.42031250216787441, -9.598844408820458085 ) ) ;
#13943=ORIENTED_EDGE ( 'NONE', *, *, #19889, .F. ) ;
#13944=CARTESIAN_POINT ( 'NONE',  ( 183.8544531269043887, 35.99999999999999289, -7.260818043106919362 ) ) ;
#13946=EDGE_LOOP ( 'NONE', ( #24613, #3203, #8315, #26982 ) ) ;
#13948=CARTESIAN_POINT ( 'NONE',  ( 189.5550856135277229, 39.61093750108393152, -13.14518615778179900 ) ) ;
#13953=CARTESIAN_POINT ( 'NONE',  ( 9.295050272127047819, 33.11210937608393579, 9.295050272127046043 ) ) ;
#13958=DIRECTION ( 'NONE',  ( -0.000000000000000000, -1.000000000000000000, -0.000000000000000000 ) ) ;
#13960=CARTESIAN_POINT ( 'NONE',  ( 185.8198241863519513, 55.00000000000000000, -15.00000000000000000 ) ) ;
#13965=DIRECTION ( 'NONE',  ( 0.000000000000000000, 0.000000000000000000, -1.000000000000000000 ) ) ;
#13967=CARTESIAN_POINT ( 'NONE',  ( 9.295050272127047819, 33.90585937608393863, 9.295050272127046043 ) ) ;
#13971=CARTESIAN_POINT ( 'NONE',  ( 189.5550856135277229, 35.14609375108393152, 13.14518615778179722 ) ) ;
#13972=ORIENTED_EDGE ( 'NONE', *, *, #3586, .T. ) ;
#13975=ORIENTED_EDGE ( 'NONE', *, *, #21526, .T. ) ;
#13978=CARTESIAN_POINT ( 'NONE',  ( 181.4251840539369596, 38.76757812716787299, 5.622872871577880183 ) ) ;
#13979=DIRECTION ( 'NONE',  ( -0.000000000000000000, 1.000000000000000000, -0.000000000000000000 ) ) ;
#13980=CARTESIAN_POINT ( 'NONE',  ( 139.2950502721270425, 37.67617187608393436, 9.295050272127046043 ) ) ;
#13981=CARTESIAN_POINT ( 'NONE',  ( 5.444914386472302859, 37.82500000108392868, 13.14518615778179189 ) ) ;
#13982=CARTESIAN_POINT ( 'NONE',  ( -13.14518615778179189, 34.25312500108393010, 5.444914386472304635 ) ) ;
#13986=VECTOR ( 'NONE', #7143, 1000.000000000000000 ) ;
#13987=CARTESIAN_POINT ( 'NONE',  ( 69.06258354057162308, 50.00000000116031629, -12.98908657125264554 ) ) ;
#13989=ORIENTED_EDGE ( 'NONE', *, *, #1814, .T. ) ;
#13990=CARTESIAN_POINT ( 'NONE',  ( 65.00000000000000000, 50.00000000000000000, -7.517135062566165128E-15 ) ) ;
#13993=ADVANCED_FACE ( 'NONE', ( #6062 ), #6329, .T. ) ;
#13994=CARTESIAN_POINT ( 'NONE',  ( 51.85481384221821344, 36.63437500108393863, 5.444914386472304635 ) ) ;
#13998=CARTESIAN_POINT ( 'NONE',  ( 208.1451861577818079, 36.93203125108394147, 5.444914386472293977 ) ) ;
#14001=( BOUNDED_CURVE ( )  B_SPLINE_CURVE ( 2, ( #27624, #14490, #16777, #14623, #23341, #21202, #10344, #19051, #27760 ),
 .UNSPECIFIED., .F., .F. ) 
 B_SPLINE_CURVE_WITH_KNOTS ( ( 3, 2, 2, 2, 3 ),
 ( 0.3958333333333331483, 0.4062499999999999445, 0.4166666666666667407, 0.4270833333333335369, 0.4375000000000003331 ),
 .UNSPECIFIED. ) 
 CURVE ( )  GEOMETRIC_REPRESENTATION_ITEM ( )  RATIONAL_B_SPLINE_CURVE ( ( 1.000000000000001110, 0.9238795325112855172, 1.000000000000000000, 0.9238795325112867385, 1.000000000000000000, 0.9238795325112867385, 1.000000000000000000, 0.9238795325112842960, 1.000000000000002442 ) ) 
 REPRESENTATION_ITEM ( '' )  );
#14004=CARTESIAN_POINT ( 'NONE',  ( 200.4449143864723055, 39.41250000108393436, 13.14518615778179189 ) ) ;
#14010=CARTESIAN_POINT ( 'NONE',  ( 139.1801758136479918, 55.00000000000000000, -15.00000000000000000 ) ) ;
#14013=CARTESIAN_POINT ( 'NONE',  ( 189.5550856135277229, 33.75703125108393721, 13.14518615778179722 ) ) ;
#14016=CARTESIAN_POINT ( 'NONE',  ( 8.772609246137605510, 50.37415326814473104, -14.99999999999999822 ) ) ;
#14017=CARTESIAN_POINT ( 'NONE',  ( 55.70494972787295751, 35.69179687608393436, -9.295050272127046043 ) ) ;
#14019=CARTESIAN_POINT ( 'NONE',  ( 124.3771271284221314, 36.18789062716787441, -13.57481594606304753 ) ) ;
#14020=CARTESIAN_POINT ( 'NONE',  ( 65.00000000000000000, 39.61093749999999147, 13.57481594606304576 ) ) ;
#14022=CARTESIAN_POINT ( 'NONE',  ( 181.8548138422181921, 40.70234375108393721, -5.444914386472297529 ) ) ;
#14023=EDGE_CURVE ( 'NONE', #18276, #5473, #27337, .T. ) ;
#14026=EDGE_LOOP ( 'NONE', ( #6738, #18079, #17091, #24750, #15568, #22022, #27670, #18458, #25149, #11975, #2295, #26333, #18411, #6101, #19529 ) ) ;
#14027=CARTESIAN_POINT ( 'NONE',  ( -13.14917398115171743, 36.00000000000000711, -1.058935892997135975 ) ) ;
#14029=CARTESIAN_POINT ( 'NONE',  ( 208.5748159460630688, 38.27148437500000711, -5.622872871577873966 ) ) ;
#14031=CARTESIAN_POINT ( 'NONE',  ( 65.00000000000000000, -7.395377635281828788, -7.517135062566165128E-15 ) ) ;
#14032=CARTESIAN_POINT ( 'NONE',  ( 78.57481594606305464, 37.57695312716787583, -5.622872871577873966 ) ) ;
#14035=CARTESIAN_POINT ( 'NONE',  ( 2.493653234604083739E-15, 39.71015625216787015, 13.57481594606304576 ) ) ;
#14037=AXIS2_PLACEMENT_3D ( 'NONE', #15642, #24341, #15916 ) ;
#14038=DIRECTION ( 'NONE',  ( -0.000000000000000000, 1.000000000000000000, -0.000000000000000000 ) ) ;
#14039=CARTESIAN_POINT ( 'NONE',  ( -4.062583540577167973, 50.00000000116096288, 12.98908657125208777 ) ) ;
#14040=CARTESIAN_POINT ( 'NONE',  ( 55.40115559117954547, 40.90078124999999432, -9.598844408820458085 ) ) ;
#14041=CARTESIAN_POINT ( 'NONE',  ( 143.5748159460630688, 35.04687499999999289, -1.662435489736055892E-15 ) ) ;
#14043=ORIENTED_EDGE ( 'NONE', *, *, #25412, .F. ) ;
#14045=SHAPE_REPRESENTATION ( 'Vacuum Distribution Tubing Harness', ( #26844 ), #12238 ) ;
#14049=CARTESIAN_POINT ( 'NONE',  ( 143.1451861577818079, 34.60039062608392868, -1.609821015232357215E-15 ) ) ;
#14050=CARTESIAN_POINT ( 'NONE',  ( 65.00000000000000000, 39.95820312608393010, 13.14518615778179544 ) ) ;
#14051=EDGE_LOOP ( 'NONE', ( #20783, #19, #16689, #14223 ) ) ;
#14053=CARTESIAN_POINT ( 'NONE',  ( 9.295050272127046043, 39.46210937608393010, -9.295050272127046043 ) ) ;
#14055=DIRECTION ( 'NONE',  ( -0.000000000000000000, 1.000000000000000000, -0.000000000000000000 ) ) ;
#14059=CARTESIAN_POINT ( 'NONE',  ( 103.5355339059327093, 82.75000000273119838, -3.535533905932755072 ) ) ;
#14060=CARTESIAN_POINT ( 'NONE',  ( 143.0420085811497302, 36.00000000000001421, -3.640726557254540197 ) ) ;
#14061=DIRECTION ( 'NONE',  ( -0.000000000000000000, -1.000000000000000000, -0.000000000000000000 ) ) ;
#14063=CARTESIAN_POINT ( 'NONE',  ( 116.8975291782781198, 36.00000000000000000, -1.608626461598027246 ) ) ;
#14070=CARTESIAN_POINT ( 'NONE',  ( 181.4251840539369596, 32.26874999999999716, 0.000000000000000000 ) ) ;
#14073=LINE ( 'NONE', #17934, #22693 ) ;
#14075=CARTESIAN_POINT ( 'NONE',  ( 78.14518615778179367, 32.16953125108393152, 5.444914386472293977 ) ) ;
#14079=DIRECTION ( 'NONE',  ( -0.000000000000000000, 1.000000000000000000, 0.000000000000000000 ) ) ;
#14081=CARTESIAN_POINT ( 'NONE',  ( 135.4449143864723055, 34.94765625108394147, -13.14518615778179900 ) ) ;
#14082=ORIENTED_EDGE ( 'NONE', *, *, #3331, .F. ) ;
#14083=CARTESIAN_POINT ( 'NONE',  ( 104.9999999999999574, 80.56250000000004263, -2.071067811865491937 ) ) ;
#14085=CARTESIAN_POINT ( 'NONE',  ( 200.6228728715778686, 36.88242187716787157, -13.57481594606304753 ) ) ;
#14086=CARTESIAN_POINT ( 'NONE',  ( 103.1528011352953342, 82.06250000136559208, -3.152801135295383084 ) ) ;
#14089=CARTESIAN_POINT ( 'NONE',  ( 65.00000000000000000, 39.71015625216787015, 13.57481594606304576 ) ) ;
#14091=CARTESIAN_POINT ( 'NONE',  ( 189.5550856135277229, 40.10703125108393152, 13.14518615778179722 ) ) ;
#14092=CARTESIAN_POINT ( 'NONE',  ( 5.622872871577871301, 40.05742187716786873, -13.57481594606304753 ) ) ;
#14095=ORIENTED_EDGE ( 'NONE', *, *, #15422, .T. ) ;
#14097=CARTESIAN_POINT ( 'NONE',  ( 200.6228728715778686, 32.61601562716786873, 13.57481594606304576 ) ) ;
#14100=CARTESIAN_POINT ( 'NONE',  ( -5.444914386472297529, 31.87187500108393223, -13.14518615778179900 ) ) ;
#14105=CARTESIAN_POINT ( 'NONE',  ( 74.59884440882045453, 36.83281250216787583, -9.598844408820458085 ) ) ;
#14113=CARTESIAN_POINT ( 'NONE',  ( 13.14518615778179900, 33.16171875108393863, 5.444914386472293977 ) ) ;
#14116=CARTESIAN_POINT ( 'NONE',  ( -9.598844408820458085, 37.72578124999999005, -9.598844408820458085 ) ) ;
#14117=CARTESIAN_POINT ( 'NONE',  ( 181.8548138422181921, 33.45937500108392726, 5.444914386472304635 ) ) ;
#14119=ORIENTED_EDGE ( 'NONE', *, *, #26215, .T. ) ;
#14120=CARTESIAN_POINT ( 'NONE',  ( 192.4704160048314634, 49.99999999938371786, -13.34625891065977932 ) ) ;
#14122=VECTOR ( 'NONE', #3321, 1000.000000000000000 ) ;
#14124=ORIENTED_EDGE ( 'NONE', *, *, #14355, .F. ) ;
#14127=CARTESIAN_POINT ( 'NONE',  ( 11.10484805054756841, 36.02027164848242791, -8.092840767093349541 ) ) ;
#14129=CARTESIAN_POINT ( 'NONE',  ( 124.5550856135277087, 38.02343750108394005, -13.14518615778179900 ) ) ;
#14130=CARTESIAN_POINT ( 'NONE',  ( 9.295050272127046043, 37.27929687608394005, -9.295050272127046043 ) ) ;
#14131=CARTESIAN_POINT ( 'NONE',  ( 5.444914386472297529, 32.36796875108393579, -13.14518615778179900 ) ) ;
#14138=CARTESIAN_POINT ( 'NONE',  ( 96.84719886470459471, 81.81250000136559208, 3.152801135295355994 ) ) ;
#14140=VECTOR ( 'NONE', #27786, 1000.000000000000000 ) ;
#14153=LINE ( 'NONE', #6271, #22090 ) ;
#14156=CARTESIAN_POINT ( 'NONE',  ( 208.1451861577817795, 33.26093750108393721, -5.444914386472297529 ) ) ;
#14159=CARTESIAN_POINT ( 'NONE',  ( 2.169956583107089276, 49.99999999883884527, -13.43548448457782918 ) ) ;
#14162=CARTESIAN_POINT ( 'NONE',  ( 120.4011555911795455, 37.03125000216787299, -9.598844408820458085 ) ) ;
#14166=CARTESIAN_POINT ( 'NONE',  ( 185.7049497278729575, 37.67617187608393436, 9.295050272127047819 ) ) ;
#14171=CARTESIAN_POINT ( 'NONE',  ( -1.271138771240642784, 36.00000000000000000, -13.43002483374384681 ) ) ;
#14172=CARTESIAN_POINT ( 'NONE',  ( 204.5988444088204403, 38.32109374999999574, -9.598844408820458085 ) ) ;
#14173=ADVANCED_FACE ( 'NONE', ( #2352 ), #19670, .T. ) ;
#14174=CARTESIAN_POINT ( 'NONE',  ( 1.137167824540872951, 35.99999999999998579, 13.09590655363602707 ) ) ;
#14175=CARTESIAN_POINT ( 'NONE',  ( 70.44491438647230552, 32.26875000108393721, 13.14518615778179189 ) ) ;
#14180=CARTESIAN_POINT ( 'NONE',  ( 9.180175813648009608, 50.00000000000000000, 9.999999999999980460 ) ) ;
#14181=CARTESIAN_POINT ( 'NONE',  ( 130.0000000000000000, 34.84843749999999574, 13.57481594606304576 ) ) ;
#14183=ORIENTED_EDGE ( 'NONE', *, *, #4113, .F. ) ;
#14184=CARTESIAN_POINT ( 'NONE',  ( 102.0710678118654187, 84.68750000000000000, -5.000000000000015987 ) ) ;
#14188=CARTESIAN_POINT ( 'NONE',  ( 116.8548138422182063, 40.70234375108393721, -5.444914386472297529 ) ) ;
#14189=CARTESIAN_POINT ( 'NONE',  ( 70.62287287157786864, 32.11992187716787583, -13.57481594606304753 ) ) ;
#14190=CARTESIAN_POINT ( 'NONE',  ( 13.57481594606304576, 37.52734375216787299, -1.662435489736055892E-15 ) ) ;
#14191=CARTESIAN_POINT ( 'NONE',  ( -13.14518615778179900, 37.32890625108393579, -5.444914386472297529 ) ) ;
#14192=EDGE_CURVE ( 'NONE', #27535, #19618, #4827, .T. ) ;
#14194=FACE_OUTER_BOUND ( 'NONE', #27324, .T. ) ;
#14196=ORIENTED_EDGE ( 'NONE', *, *, #13135, .T. ) ;
#14197=CARTESIAN_POINT ( 'NONE',  ( 13.14518615778179900, 40.20625000108393010, -5.444914386472297529 ) ) ;
#14198=DIRECTION ( 'NONE',  ( -0.000000000000000000, 1.000000000000000000, -0.000000000000000000 ) ) ;
#14199=CARTESIAN_POINT ( 'NONE',  ( 65.00000000000000000, -7.395377635281828788, -13.57481594606305109 ) ) ;
#14200=EDGE_CURVE ( 'NONE', #28009, #9895, #18094, .T. ) ;
#14214=CARTESIAN_POINT ( 'NONE',  ( 97.92893218813443923, 80.18750000000001421, 4.999999999999927169 ) ) ;
#14215=CARTESIAN_POINT ( 'NONE',  ( 95.54126587499995082, 83.50000000136560629, 1.846868145590724986 ) ) ;
#14216=CARTESIAN_POINT ( 'NONE',  ( 65.00000000000000000, 40.55351562608393579, -13.14518615778179544 ) ) ;
#14220=CARTESIAN_POINT ( 'NONE',  ( -9.598844408820458085, 33.75703124999999005, -9.598844408820458085 ) ) ;
#14222=CARTESIAN_POINT ( 'NONE',  ( 143.1451861577818079, 34.79882812608394005, -1.609821015232357215E-15 ) ) ;
#14223=ORIENTED_EDGE ( 'NONE', *, *, #6047, .F. ) ;
#14224=DIRECTION ( 'NONE',  ( -1.000000000000000000, 0.000000000000000000, 2.385244779468110248E-16 ) ) ;
#14225=CARTESIAN_POINT ( 'NONE',  ( 95.54126587499995082, 83.50000000136560629, 1.846868145590724986 ) ) ;
#14226=CARTESIAN_POINT ( 'NONE',  ( 124.5550856135277087, 38.81718750108393579, -13.14518615778179900 ) ) ;
#14227=CARTESIAN_POINT ( 'NONE',  ( 65.00000000000000000, 39.31328125216787583, -13.57481594606304576 ) ) ;
#14229=CARTESIAN_POINT ( 'NONE',  ( 185.7049497278729575, 40.05742187608393579, 9.295050272127047819 ) ) ;
#14230=CARTESIAN_POINT ( 'NONE',  ( -13.57481594606304753, 39.46210937716787726, -5.622872871577873077 ) ) ;
#14231=ORIENTED_EDGE ( 'NONE', *, *, #5465, .T. ) ;
#14236=CARTESIAN_POINT ( 'NONE',  ( 189.3771271284221314, 31.42539062716787157, -13.57481594606304753 ) ) ;
#14237=FACE_OUTER_BOUND ( 'NONE', #12300, .T. ) ;
#14238=EDGE_CURVE ( 'NONE', #8092, #12157, #6425, .T. ) ;
#14240=CARTESIAN_POINT ( 'NONE',  ( 120.7049497278729575, 40.45429687608393721, -9.295050272127046043 ) ) ;
#14242=FACE_OUTER_BOUND ( 'NONE', #1058, .T. ) ;
#14245=CARTESIAN_POINT ( 'NONE',  ( 204.5988444088204687, 39.71015624999999716, 9.598844408820456309 ) ) ;
#14246=CARTESIAN_POINT ( 'NONE',  ( 117.0005117698093784, 35.99999999999999289, 1.999176114741889165 ) ) ;
#14248=CARTESIAN_POINT ( 'NONE',  ( 55.70494972787295751, 40.45429687608393721, -9.295050272127046043 ) ) ;
#14254=CARTESIAN_POINT ( 'NONE',  ( 9.295050272127046043, 33.31054687608394005, -9.295050272127046043 ) ) ;
#14257=CARTESIAN_POINT ( 'NONE',  ( 103.1528011352953342, 82.06250000136559208, 3.152801135295355106 ) ) ;
#14258=( BOUNDED_CURVE ( )  B_SPLINE_CURVE ( 2, ( #18635, #27339, #14059, #3248, #981, #27474, #26918, #7362, #18351 ),
 .UNSPECIFIED., .F., .T. ) 
 B_SPLINE_CURVE_WITH_KNOTS ( ( 3, 2, 2, 2, 3 ),
 ( 0.2500000000000002220, 0.2750000000000002442, 0.3000000000000002665, 0.3250000000000002887, 0.3500000000000003109 ),
 .UNSPECIFIED. ) 
 CURVE ( )  GEOMETRIC_REPRESENTATION_ITEM ( )  RATIONAL_B_SPLINE_CURVE ( ( 0.9999999999999993339, 0.9238795325112874046, 1.000000000000000000, 0.9238795325112867385, 1.000000000000000000, 0.9238795325112867385, 1.000000000000000000, 0.9238795325112857393, 1.000000000000001110 ) ) 
 REPRESENTATION_ITEM ( '' )  );
#14260=CARTESIAN_POINT ( 'NONE',  ( 200.4449143864723055, 33.95546875108393436, -13.14518615778179900 ) ) ;
#14262=CARTESIAN_POINT ( 'NONE',  ( 188.5871333237481053, 50.00000000108477849, -11.99502265407749668 ) ) ;
#14264=ORIENTED_EDGE ( 'NONE', *, *, #15422, .F. ) ;
#14267=CARTESIAN_POINT ( 'NONE',  ( 181.4251840539369596, 38.71796875216787726, 0.000000000000000000 ) ) ;
#14269=CARTESIAN_POINT ( 'NONE',  ( 13.14518615778179722, 38.81718750108393579, -5.444914386472297529 ) ) ;
#14271=CARTESIAN_POINT ( 'NONE',  ( 5.444914386472302859, 32.86406250108392868, 13.14518615778179189 ) ) ;
#14277=CARTESIAN_POINT ( 'NONE',  ( 96.84719886470459471, 83.81250000136560629, 3.152801135295355994 ) ) ;
#14288=CARTESIAN_POINT ( 'NONE',  ( -9.598844408820458085, 40.10703124999999147, -9.598844408820458085 ) ) ;
#14291=ORIENTED_EDGE ( 'NONE', *, *, #8444, .T. ) ;
#14293=CARTESIAN_POINT ( 'NONE',  ( 51.85481384221820633, 36.73359375108393010, -5.444914386472297529 ) ) ;
#14297=CARTESIAN_POINT ( 'NONE',  ( 65.00000000000000000, 37.22968749999999716, 13.57481594606304576 ) ) ;
#14300=CARTESIAN_POINT ( 'NONE',  ( 139.5988444088204403, 39.21406250216787015, -9.598844408820458085 ) ) ;
#14303=CARTESIAN_POINT ( 'NONE',  ( 208.1451861577817795, 39.51171875108392584, 5.444914386472293977 ) ) ;
#14307=CARTESIAN_POINT ( 'NONE',  ( 9.598844408820456309, 39.90859374999999432, -9.598844408820458085 ) ) ;
#14311=CARTESIAN_POINT ( 'NONE',  ( 9.295050272127047819, 36.08867187608392868, 9.295050272127046043 ) ) ;
#14312=CIRCLE ( 'NONE', #27546, 4.999999999999999112 ) ;
#14313=CARTESIAN_POINT ( 'NONE',  ( 217.9999999999999716, 80.00000000000000000, -13.00000000000000000 ) ) ;
#14315=CARTESIAN_POINT ( 'NONE',  ( 135.6228728715778971, 33.31054687499999289, 13.57481594606304576 ) ) ;
#14316=VERTEX_POINT ( 'NONE', #15837 ) ;
#14318=CARTESIAN_POINT ( 'NONE',  ( 78.57481594606305464, 36.63437499999999858, -1.662435489736055892E-15 ) ) ;
#14323=CARTESIAN_POINT ( 'NONE',  ( 135.4449143864723055, 38.61875000108393152, 13.14518615778179189 ) ) ;
#14324=CARTESIAN_POINT ( 'NONE',  ( 78.14518615778179367, 37.77539062608393294, -1.609821015232357215E-15 ) ) ;
#14325=B_SPLINE_CURVE_WITH_KNOTS ( 'NONE', 3,
 ( #18986, #22998, #25413, #25550, #5471, #18848, #5614, #20860, #18716, #14423, #23139, #3468, #22860, #1342, #3614, #12273, #12548, #12414 ),
 .UNSPECIFIED., .F., .F.,
 ( 4, 2, 2, 2, 2, 2, 2, 2, 4 ),
 ( 0.000000000000000000, 0.004618502246277170556, 0.006927753369415742823, 0.009237004492554316826, 0.01039163005412362291, 0.01154625561569293073, 0.01385550673883149779, 0.01616475786197006659, 0.01847400898510863712 ),
 .UNSPECIFIED. ) ;
#14328=CARTESIAN_POINT ( 'NONE',  ( -9.295050272127046043, 38.86679687608393863, -9.295050272127046043 ) ) ;
#14335=CARTESIAN_POINT ( 'NONE',  ( 139.4320061696339508, 36.00000000000000000, 9.391769196590345814 ) ) ;
#14338=CARTESIAN_POINT ( 'NONE',  ( 126.5797791878282226, 36.00000000000000711, -13.02105590829171256 ) ) ;
#14339=EDGE_CURVE ( 'NONE', #8588, #5516, #2200, .T. ) ;
#14340=CARTESIAN_POINT ( 'NONE',  ( 185.4011555911795597, 39.61093750216787868, 9.598844408820459861 ) ) ;
#14342=CARTESIAN_POINT ( 'NONE',  ( 204.1801758136480203, 50.00000000000000000, -10.00000000000000000 ) ) ;
#14351=CARTESIAN_POINT ( 'NONE',  ( 96.84719886470459471, 83.56250000136560629, -3.152801135295383084 ) ) ;
#14352=CARTESIAN_POINT ( 'NONE',  ( 65.00000000000000000, 40.15664062608393436, 13.14518615778179544 ) ) ;
#14355=EDGE_CURVE ( 'NONE', #20160, #2344, #1433, .T. ) ;
#14359=CARTESIAN_POINT ( 'NONE',  ( 139.2950502721270425, 34.10429687608393579, -9.295050272127046043 ) ) ;
#14360=ORIENTED_EDGE ( 'NONE', *, *, #7090, .F. ) ;
#14364=CARTESIAN_POINT ( 'NONE',  ( 99.99999999999995737, 83.18750000136560629, -4.458734125000016313 ) ) ;
#14365=CARTESIAN_POINT ( 'NONE',  ( 116.8548138422182063, 39.01562500108393294, 5.444914386472304635 ) ) ;
#14366=CARTESIAN_POINT ( 'NONE',  ( 55.40115559117954547, 40.20625000216787726, -9.598844408820458085 ) ) ;
#14367=EDGE_CURVE ( 'NONE', #6540, #19007, #6708, .T. ) ;
#14369=CARTESIAN_POINT ( 'NONE',  ( 5.622872871577871301, 37.67617187716787441, -13.57481594606304753 ) ) ;
#14370=EDGE_LOOP ( 'NONE', ( #21521, #12178, #12159, #22746 ) ) ;
#14372=EDGE_CURVE ( 'NONE', #7460, #27733, #26263, .T. ) ;
#14373=ORIENTED_EDGE ( 'NONE', *, *, #21548, .F. ) ;
#14375=CARTESIAN_POINT ( 'NONE',  ( 189.5550856135277229, 39.11484375108394573, 13.14518615778179722 ) ) ;
#14376=( BOUNDED_CURVE ( )  B_SPLINE_CURVE ( 2, ( #22620, #5229, #14040, #3090, #11757 ),
 .UNSPECIFIED., .F., .F. ) 
 B_SPLINE_CURVE_WITH_KNOTS ( ( 3, 2, 3 ),
 ( 0.000000000000000000, 0.01041666666666679446, 0.02083333333333358892 ),
 .UNSPECIFIED. ) 
 CURVE ( )  GEOMETRIC_REPRESENTATION_ITEM ( )  RATIONAL_B_SPLINE_CURVE ( ( 1.000000000000000000, 0.9238795325112867385, 1.000000000000000000, 0.9238795325112848511, 1.000000000000001776 ) ) 
 REPRESENTATION_ITEM ( '' )  );
#14378=CARTESIAN_POINT ( 'NONE',  ( 130.0000000000000000, 38.76757812608393294, -13.14518615778179544 ) ) ;
#14379=CARTESIAN_POINT ( 'NONE',  ( -13.14518615778179189, 32.07031250108393294, 5.444914386472304635 ) ) ;
#14383=CARTESIAN_POINT ( 'NONE',  ( 208.5748159460630120, 40.55351562499998863, 5.622872871577869525 ) ) ;
#14384=ADVANCED_FACE ( 'NONE', ( #24124 ), #9850, .T. ) ;
#14393=PLANE ( 'NONE',  #22118 ) ;
#14394=CARTESIAN_POINT ( 'NONE',  ( -13.57481594606304576, 40.99999999999999289, 0.000000000000000000 ) ) ;
#14396=CARTESIAN_POINT ( 'NONE',  ( 104.4587341249999781, 84.25000000136559208, -1.846868145590750299 ) ) ;
#14398=ORIENTED_EDGE ( 'NONE', *, *, #2854, .F. ) ;
#14400=EDGE_LOOP ( 'NONE', ( #12274, #6240, #8773, #11440 ) ) ;
#14402=CARTESIAN_POINT ( 'NONE',  ( 188.9140557840131862, 54.65299103241510181, -15.00000000000000000 ) ) ;
#14408=CARTESIAN_POINT ( 'NONE',  ( 51.85481384221820633, 40.55351562608393579, 0.000000000000000000 ) ) ;
#14412=CARTESIAN_POINT ( 'NONE',  ( 116.8548138422182205, 38.37070312608393152, 0.000000000000000000 ) ) ;
#14413=CARTESIAN_POINT ( 'NONE',  ( -8.049105076161786076E-16, 33.21132812608393436, -13.14518615778179544 ) ) ;
#14414=CARTESIAN_POINT ( 'NONE',  ( 78.57481594606304043, 38.96601562499999005, 5.622872871577869525 ) ) ;
#14415=CARTESIAN_POINT ( 'NONE',  ( 65.00000000000000000, 38.02343749999999289, 13.57481594606304576 ) ) ;
#14420=CARTESIAN_POINT ( 'NONE',  ( 95.54126587499996504, 82.75000000136560629, 1.846868145590724986 ) ) ;
#14422=LINE ( 'NONE', #16288, #19951 ) ;
#14423=CARTESIAN_POINT ( 'NONE',  ( 66.50101912430496043, 53.60014735326988955, 14.99999999999997868 ) ) ;
#14427=CARTESIAN_POINT ( 'NONE',  ( 208.1451861577818079, 36.33671875108393579, 5.444914386472293977 ) ) ;
#14429=EDGE_CURVE ( 'NONE', #3560, #27809, #12738, .T. ) ;
#14430=FACE_OUTER_BOUND ( 'NONE', #19132, .T. ) ;
#14433=CARTESIAN_POINT ( 'NONE',  ( 65.00000000000000000, 38.96601562608393721, -13.14518615778179544 ) ) ;
#14435=CARTESIAN_POINT ( 'NONE',  ( 2.493653234604083739E-15, 39.61093749999999147, 13.57481594606304576 ) ) ;
#14437=CARTESIAN_POINT ( 'NONE',  ( 70.62287287157795390, 37.27929687499999289, 13.57481594606297115 ) ) ;
#14438=LINE ( 'NONE', #6045, #22261 ) ;
#14439=LINE ( 'NONE', #23156, #21808 ) ;
#14442=CARTESIAN_POINT ( 'NONE',  ( 124.3771271284221314, 34.10429687716786873, 13.57481594606304753 ) ) ;
#14445=CARTESIAN_POINT ( 'NONE',  ( 189.5550856135277229, 37.72578125108395142, 13.14518615778179722 ) ) ;
#14449=CARTESIAN_POINT ( 'NONE',  ( 5.622872871577780707, 38.37070312499999858, -13.57481594606313990 ) ) ;
#14451=LINE ( 'NONE', #8045, #22627 ) ;
#14452=CARTESIAN_POINT ( 'NONE',  ( 135.6228728715779823, 40.05742187716787583, -13.57481594606294095 ) ) ;
#14454=CARTESIAN_POINT ( 'NONE',  ( 97.92893218813456713, 80.81250000000000000, -5.000000000000067502 ) ) ;
#14455=CARTESIAN_POINT ( 'NONE',  ( 13.45411265623082109, 36.00000000000000000, 0.6772748633563333565 ) ) ;
#14456=CARTESIAN_POINT ( 'NONE',  ( 99.99999999999995737, 82.75000000000000000, -5.000000000000018652 ) ) ;
#14457=CARTESIAN_POINT ( 'NONE',  ( 124.3771271284221314, 32.11992187499999574, -13.57481594606304753 ) ) ;
#14460=CARTESIAN_POINT ( 'NONE',  ( 70.62287287157801074, 36.78320312499999289, -13.57481594606290898 ) ) ;
#14465=CARTESIAN_POINT ( 'NONE',  ( 130.0000000000000000, 39.36289062608393152, 13.14518615778179544 ) ) ;
#14466=CARTESIAN_POINT ( 'NONE',  ( 55.70494972787295751, 35.69179687608393436, -9.295050272127046043 ) ) ;
#14467=B_SPLINE_CURVE_WITH_KNOTS ( 'NONE', 3,
 ( #15712, #15990, #20284, #24705, #11567, #770, #11138, #4904, #9444, #21613, #13566, #2765, #23748, #18143, #26857, #19853, #7303, #5185, #340, #13848, #22573, #3040, #19326, #28030, #8496, #24276, #25887, #20149, #15030, #4224, #11429 ),
 .UNSPECIFIED., .F., .F.,
 ( 4, 2, 2, 2, 2, 2, 2, 2, 2, 2, 1, 2, 2, 2, 2, 4 ),
 ( 0.000000000000000000, 0.001647793485000502694, 0.003295586970001005388, 0.004943380455001507648, 0.005767277197501759212, 0.006591173940002010775, 0.008238967425002545128, 0.009886760910003079481, 0.01318234788000417941, 0.01483014136500472938, 0.01647793485000527761, 0.01812572833500582931, 0.01977352182000637754, 0.02306910879000747400, 0.02471690227500801876, 0.02636469576000856352 ),
 .UNSPECIFIED. ) ;
#14469=CARTESIAN_POINT ( 'NONE',  ( -9.295050272127044266, 34.30273437608393294, 9.295050272127047819 ) ) ;
#14470=DIRECTION ( 'NONE',  ( 0.000000000000000000, 0.000000000000000000, 1.000000000000000000 ) ) ;
#14476=CARTESIAN_POINT ( 'NONE',  ( 200.6228728715778971, 40.45429687500001137, 13.57481594606306174 ) ) ;
#14477=CARTESIAN_POINT ( 'NONE',  ( -13.14518615778179900, 38.12265625108393152, -5.444914386472297529 ) ) ;
#14480=AXIS2_PLACEMENT_3D ( 'NONE', #22479, #534, #2673 ) ;
#14482=DIRECTION ( 'NONE',  ( -0.000000000000000000, -1.000000000000000000, -0.000000000000000000 ) ) ;
#14490=CARTESIAN_POINT ( 'NONE',  ( 189.3771271284221882, 36.48554687716787726, 13.57481594606311504 ) ) ;
#14491=CARTESIAN_POINT ( 'NONE',  ( 101.8468681455906903, 84.37500000136562051, -4.458734125000016313 ) ) ;
#14492=CARTESIAN_POINT ( 'NONE',  ( 51.85481384221820633, 38.37070312608393152, 0.000000000000000000 ) ) ;
#14498=CARTESIAN_POINT ( 'NONE',  ( 139.5988444088204687, 40.50390624999999289, 9.598844408820456309 ) ) ;
#14499=EDGE_LOOP ( 'NONE', ( #25346, #13113, #20338, #20697 ) ) ;
#14500=DIRECTION ( 'NONE',  ( 0.000000000000000000, 0.000000000000000000, 1.000000000000000000 ) ) ;
#14503=CARTESIAN_POINT ( 'NONE',  ( 130.0000000000000000, 40.35507812608393152, -13.14518615778179544 ) ) ;
#14504=CARTESIAN_POINT ( 'NONE',  ( 78.57481594606304043, 36.78320312716786589, -5.622872871577873077 ) ) ;
#14507=CARTESIAN_POINT ( 'NONE',  ( 9.598844408820459861, 35.84062500216786873, 9.598844408820456309 ) ) ;
#14512=CARTESIAN_POINT ( 'NONE',  ( 208.1451861577818079, 40.15664062608393436, -1.609821015232357215E-15 ) ) ;
#14515=CARTESIAN_POINT ( 'NONE',  ( 143.1451861577818363, 36.93203125108394147, 5.444914386472293977 ) ) ;
#14516=CARTESIAN_POINT ( 'NONE',  ( -5.444914386472297529, 33.45937500108394147, -13.14518615778179900 ) ) ;
#14517=EDGE_CURVE ( 'NONE', #18933, #8752, #9000, .T. ) ;
#14518=CARTESIAN_POINT ( 'NONE',  ( -15.00000000000000000, 50.00000000000000000, 10.00000000000000000 ) ) ;
#14519=CARTESIAN_POINT ( 'NONE',  ( -20.00000000000000000, 80.00000000000000000, 13.00000000000000178 ) ) ;
#14522=CARTESIAN_POINT ( 'NONE',  ( 195.0000000000000000, 36.83281249999999574, -13.57481594606304576 ) ) ;
#14524=CARTESIAN_POINT ( 'NONE',  ( 128.9781962812409120, 36.00000000000000711, 13.11239906893445095 ) ) ;
#14526=CARTESIAN_POINT ( 'NONE',  ( 51.85481384221820633, 38.22187500108393010, 5.444914386472304635 ) ) ;
#14530=CARTESIAN_POINT ( 'NONE',  ( 99.99999999999995737, 85.00000000000000000, 2.999999999999990674 ) ) ;
#14533=CARTESIAN_POINT ( 'NONE',  ( 6.944423624769117787, 31.75150628229955529, -11.16113343896966370 ) ) ;
#14536=CARTESIAN_POINT ( 'NONE',  ( 96.84719886470459471, 81.56250000136559208, -3.152801135295383084 ) ) ;
#14539=ORIENTED_EDGE ( 'NONE', *, *, #4744, .F. ) ;
#14541=DIRECTION ( 'NONE',  ( -0.000000000000000000, 1.000000000000000000, 0.000000000000000000 ) ) ;
#14544=ORIENTED_EDGE ( 'NONE', *, *, #1856, .T. ) ;
#14547=CARTESIAN_POINT ( 'NONE',  ( 195.0000000000000000, 38.91640625216786731, 13.57481594606304576 ) ) ;
#14550=CARTESIAN_POINT ( 'NONE',  ( 124.5550856135277087, 39.01562500108394005, -13.14518615778179722 ) ) ;
#14551=CARTESIAN_POINT ( 'NONE',  ( -9.295050272127046043, 32.51679687608393721, -9.295050272127046043 ) ) ;
#14553=EDGE_LOOP ( 'NONE', ( #26985, #23038, #27697 ) ) ;
#14554=CARTESIAN_POINT ( 'NONE',  ( 51.42518405393695957, 36.98164062499999005, -5.622872871577873077 ) ) ;
#14557=CARTESIAN_POINT ( 'NONE',  ( -13.57481594606304753, 37.08085937716787583, -5.622872871577872189 ) ) ;
#14561=CARTESIAN_POINT ( 'NONE',  ( 101.8468681455907046, 82.37500000136563472, -4.458734125000016313 ) ) ;
#14563=CARTESIAN_POINT ( 'NONE',  ( -8.049105076161786076E-16, 39.75976562608394005, -13.14518615778179544 ) ) ;
#14569=CARTESIAN_POINT ( 'NONE',  ( 65.00000000000000000, -7.395377635281828788, 13.57481594606303688 ) ) ;
#14571=ORIENTED_EDGE ( 'NONE', *, *, #17313, .F. ) ;
#14572=CARTESIAN_POINT ( 'NONE',  ( 78.14518615778179367, 37.18007812608393436, -1.609821015232357215E-15 ) ) ;
#14574=CARTESIAN_POINT ( 'NONE',  ( 130.0000000000000000, 36.03906250000000000, -13.57481594606304576 ) ) ;
#14579=CARTESIAN_POINT ( 'NONE',  ( 116.4251840539369454, 33.11210937716786873, -5.622872871577873077 ) ) ;
#14580=( BOUNDED_SURFACE ( )  B_SPLINE_SURFACE ( 3, 2, ( 
 ( #24134, #4610, #13268 ),
 ( #20002, #914, #11136 ),
 ( #15988, #5325, #24559 ),
 ( #11425, #6878, #24844 ),
 ( #16136, #15709, #22423 ),
 ( #15850, #2894, #2619 ),
 ( #13987, #9584, #13563 ),
 ( #17996, #18288, #5041 ),
 ( #19851, #22571, #26561 ),
 ( #338, #9300, #13705 ),
 ( #11282, #3037, #26994 ),
 ( #482, #11707, #22712 ),
 ( #7440, #9025, #26705 ),
 ( #9164, #17717, #26419 ),
 ( #20431, #15563, #17856 ),
 ( #2762, #11563, #7013 ),
 ( #24273, #4754, #13414 ),
 ( #22140, #24411, #766 ),
 ( #20144, #4901, #22286 ),
 ( #9440, #625, #7154 ) ),
 .UNSPECIFIED., .F., .F., .F. ) 
 B_SPLINE_SURFACE_WITH_KNOTS ( ( 4, 2, 2, 2, 2, 2, 2, 2, 2, 4 ),
 ( 3, 3 ),
 ( 0.009073803551359473779, 0.01139250602759182655, 0.01371120850382417933, 0.01602991098005653037, 0.01834861345628888488, 0.01950796469440506387, 0.02066731593252123939, 0.02298601840875359043, 0.02530472088498594146, 0.02762342336121829597 ),
 ( 0.000000000000000000, 1.000000000000000000 ),
 .UNSPECIFIED. ) 
 GEOMETRIC_REPRESENTATION_ITEM ( )  RATIONAL_B_SPLINE_SURFACE ( (
 ( 1.000000000000000000, 0.7071067811865476838, 1.000000000000000000),
 ( 1.000000000000000000, 0.7344871497828565632, 1.000000000000000000),
 ( 1.000000000000000000, 0.7612510203319298174, 1.000000000000000000),
 ( 1.000000000000000000, 0.8116663633843581582, 1.000000000000000000),
 ( 1.000000000000000000, 0.8353358059749911302, 1.000000000000000000),
 ( 1.000000000000000000, 0.8764699612587956157, 1.000000000000000000),
 ( 1.000000000000000000, 0.8939017358718738260, 1.000000000000000000),
 ( 1.000000000000000000, 0.9185314935647551637, 1.000000000000000000),
 ( 1.000000000000000000, 0.9256439951239044950, 1.000000000000000000),
 ( 1.000000000000000000, 0.9261623622476727880, 1.000000000000000000),
 ( 1.000000000000000000, 0.9246301385978410448, 1.000000000000000000),
 ( 1.000000000000000000, 0.9183304321348457755, 1.000000000000000000),
 ( 1.000000000000000000, 0.9135987334167977592, 1.000000000000000000),
 ( 1.000000000000000000, 0.8954110486040547379, 1.000000000000000000),
 ( 1.000000000000000000, 0.8779877431162230739, 1.000000000000000000),
 ( 1.000000000000000000, 0.8366182664711283579, 1.000000000000000000),
 ( 1.000000000000000000, 0.8126941604016590937, 1.000000000000000000),
 ( 1.000000000000000000, 0.7617527316304667506, 1.000000000000000000),
 ( 1.000000000000000000, 0.7347103785792968855, 1.000000000000000000),
 ( 1.000000000000000000, 0.7071067811865466846, 1.000000000000000000) ) ) 
 REPRESENTATION_ITEM ( '' )  SURFACE ( )  );
#14581=DIRECTION ( 'NONE',  ( 0.000000000000000000, 0.000000000000000000, 1.000000000000000000 ) ) ;
#14583=EDGE_CURVE ( 'NONE', #26363, #6724, #8480, .T. ) ;
#14584=CARTESIAN_POINT ( 'NONE',  ( 200.4449143864723055, 38.12265625108393152, -13.14518615778179900 ) ) ;
#14585=ORIENTED_EDGE ( 'NONE', *, *, #9159, .F. ) ;
#14588=CARTESIAN_POINT ( 'NONE',  ( 96.84719886470459471, 84.31250000136560629, -3.152801135295383084 ) ) ;
#14591=CIRCLE ( 'NONE', #19162, 4.999999999999997335 ) ;
#14592=CARTESIAN_POINT ( 'NONE',  ( 99.99999999999995737, 85.00000000000000000, -1.387778780781445676E-14 ) ) ;
#14593=CARTESIAN_POINT ( 'NONE',  ( 7.754123975994470896, 35.99999999999999289, 10.77549638133777421 ) ) ;
#14594=SPHERICAL_SURFACE ( 'NONE', #8586, 5.000000000000000000 ) ;
#14597=PRODUCT_DEFINITION_CONTEXT ( 'detailed design', #25524, 'design' ) ;
#14601=CARTESIAN_POINT ( 'NONE',  ( 124.5550856135277087, 40.10703125108393152, 13.14518615778179722 ) ) ;
#14602=CARTESIAN_POINT ( 'NONE',  ( 78.14518615778179367, 35.34453125108392868, 5.444914386472293977 ) ) ;
#14605=CARTESIAN_POINT ( 'NONE',  ( 5.444914386472297529, 34.74921875108394431, -13.14518615778179900 ) ) ;
#14606=CARTESIAN_POINT ( 'NONE',  ( 51.42518405393695957, 36.23749999999999005, 0.000000000000000000 ) ) ;
#14607=CARTESIAN_POINT ( 'NONE',  ( 193.9781962812411393, 35.99999999999997158, 13.11239906893446516 ) ) ;
#14609=DIRECTION ( 'NONE',  ( 1.000000000000000000, -0.000000000000000000, -7.228014483236696740E-18 ) ) ;
#14610=CARTESIAN_POINT ( 'NONE',  ( 13.14518615778179900, 38.61875000108393152, -5.444914386472297529 ) ) ;
#14611=CARTESIAN_POINT ( 'NONE',  ( 143.4955014123171395, 36.00000000000000000, -0.9550757908099576365 ) ) ;
#14613=DIRECTION ( 'NONE',  ( -0.000000000000000000, 1.000000000000000000, -0.000000000000000000 ) ) ;
#14615=DIRECTION ( 'NONE',  ( 0.000000000000000000, 1.000000000000000000, 0.000000000000000000 ) ) ;
#14618=ORIENTED_EDGE ( 'NONE', *, *, #18246, .T. ) ;
#14623=CARTESIAN_POINT ( 'NONE',  ( 181.4251840539369596, 36.38632812716788578, 5.622872871577880183 ) ) ;
#14624=CARTESIAN_POINT ( 'NONE',  ( 99.99999999999995737, 80.18750000136559208, -4.458734125000016313 ) ) ;
#14625=CARTESIAN_POINT ( 'NONE',  ( 55.70494972787295751, 36.88242187608393152, 9.295050272127047819 ) ) ;
#14631=CARTESIAN_POINT ( 'NONE',  ( 124.5550856135277087, 32.66562500108393863, -13.14518615778179900 ) ) ;
#14636=CARTESIAN_POINT ( 'NONE',  ( 101.8468681455906903, 81.12500000136559208, -4.458734125000016313 ) ) ;
#14637=CARTESIAN_POINT ( 'NONE',  ( 143.1451861577818079, 40.15664062608393436, -1.609821015232357215E-15 ) ) ;
#14638=CARTESIAN_POINT ( 'NONE',  ( 55.40115559117954547, 37.22968750216787726, 9.598844408820459861 ) ) ;
#14640=CARTESIAN_POINT ( 'NONE',  ( 13.57481594606304576, 34.35234375216787583, -1.662435489736055892E-15 ) ) ;
#14641=EDGE_LOOP ( 'NONE', ( #6322, #27013, #6688, #18092 ) ) ;
#14645=CARTESIAN_POINT ( 'NONE',  ( 195.0000000000000000, 36.38632812608393152, -13.14518615778179544 ) ) ;
#14647=CARTESIAN_POINT ( 'NONE',  ( 135.4449143864723339, 37.13046875108393152, -13.14518615778179722 ) ) ;
#14648=CARTESIAN_POINT ( 'NONE',  ( 181.4251840539369596, 37.92421875216787441, 0.000000000000000000 ) ) ;
#14649=CARTESIAN_POINT ( 'NONE',  ( 143.5748159460630688, 37.47773437500001137, -5.622872871577873966 ) ) ;
#14651=CARTESIAN_POINT ( 'NONE',  ( 55.40115559117954547, 37.13046874999999147, 9.598844408820459861 ) ) ;
#14653=CARTESIAN_POINT ( 'NONE',  ( 208.5748159460630120, 39.06523437499998863, -5.622872871577873077 ) ) ;
#14654=CARTESIAN_POINT ( 'NONE',  ( 59.37712712842198926, 39.56132812500000284, 13.57481594606290720 ) ) ;
#14656=CARTESIAN_POINT ( 'NONE',  ( 74.29505027212704249, 38.46992187608393010, 9.295050272127046043 ) ) ;
#14660=DIRECTION ( 'NONE',  ( 0.000000000000000000, 1.000000000000000000, 0.000000000000000000 ) ) ;
#14661=CARTESIAN_POINT ( 'NONE',  ( -13.57481594606304576, 40.20624999999999005, 0.000000000000000000 ) ) ;
#14662=CARTESIAN_POINT ( 'NONE',  ( 130.0000000000000000, 40.15664062608393436, 13.14518615778179544 ) ) ;
#14664=CARTESIAN_POINT ( 'NONE',  ( 98.15313185440925281, 83.87500000136560629, 4.458734124999987891 ) ) ;
#14668=EDGE_CURVE ( 'NONE', #10173, #14872, #19957, .T. ) ;
#14669=ORIENTED_EDGE ( 'NONE', *, *, #25348, .T. ) ;
#14675=CARTESIAN_POINT ( 'NONE',  ( 185.4011555911795313, 37.03125000216787299, -9.598844408820458085 ) ) ;
#14678=CARTESIAN_POINT ( 'NONE',  ( 197.2761468445513060, 51.46995505939148785, 14.99999999999995559 ) ) ;
#14679=CARTESIAN_POINT ( 'NONE',  ( 143.1451861577818079, 37.97382812608393721, -1.609821015232357215E-15 ) ) ;
#14680=CARTESIAN_POINT ( 'NONE',  ( -5.444914386472297529, 31.67343750108393863, -13.14518615778179900 ) ) ;
#14682=CARTESIAN_POINT ( 'NONE',  ( 51.42518405393695957, 36.28710937499999289, 5.622872871577880183 ) ) ;
#14685=CARTESIAN_POINT ( 'NONE',  ( 207.2511908804448240, 36.00000000000000711, 5.405483146087288304 ) ) ;
#14690=CARTESIAN_POINT ( 'NONE',  ( -9.180175813647991845, 50.00000000000000000, -9.999999999999998224 ) ) ;
#14692=CARTESIAN_POINT ( 'NONE',  ( 5.444914386472302859, 38.61875000108393152, 13.14518615778179189 ) ) ;
#14696=( BOUNDED_CURVE ( )  B_SPLINE_CURVE ( 2, ( #4821, #26483, #4964, #13626, #20911, #9785, #25459, #27201, #7653 ),
 .UNSPECIFIED., .F., .F. ) 
 B_SPLINE_CURVE_WITH_KNOTS ( ( 3, 2, 2, 2, 3 ),
 ( 0.3125000000000002220, 0.3229166666666668517, 0.3333333333333334259, 0.3437500000000000555, 0.3541666666666666852 ),
 .UNSPECIFIED. ) 
 CURVE ( )  GEOMETRIC_REPRESENTATION_ITEM ( )  RATIONAL_B_SPLINE_CURVE ( ( 0.9999999999999983347, 0.9238795325112884038, 1.000000000000000000, 0.9238795325112867385, 1.000000000000000000, 0.9238795325112867385, 1.000000000000000000, 0.9238795325112867385, 1.000000000000000000 ) ) 
 REPRESENTATION_ITEM ( '' )  );
#14705=CARTESIAN_POINT ( 'NONE',  ( 70.44491438647229131, 37.32890625108393579, -13.14518615778179722 ) ) ;
#14706=EDGE_CURVE ( 'NONE', #16151, #3976, #9515, .T. ) ;
#14708=CIRCLE ( 'NONE', #19725, 4.999999999999999112 ) ;
#14711=CARTESIAN_POINT ( 'NONE',  ( 116.4251840539369596, 37.77539062499998579, -5.622872871577872189 ) ) ;
#14712=FACE_OUTER_BOUND ( 'NONE', #6273, .T. ) ;
#14714=CARTESIAN_POINT ( 'NONE',  ( 120.4011555911795455, 35.64218750216787868, 9.598844408820459861 ) ) ;
#14717=CARTESIAN_POINT ( 'NONE',  ( 195.0000000000000000, 38.96601562608393721, -13.14518615778179544 ) ) ;
#14718=ORIENTED_EDGE ( 'NONE', *, *, #23600, .T. ) ;
#14722=DIRECTION ( 'NONE',  ( 0.000000000000000000, 0.000000000000000000, -1.000000000000000000 ) ) ;
#14724=CARTESIAN_POINT ( 'NONE',  ( 0.000000000000000000, -7.395377635281828788, 0.000000000000000000 ) ) ;
#14725=CARTESIAN_POINT ( 'NONE',  ( 78.57481594606305464, 39.95820312716787726, -5.622872871577873966 ) ) ;
#14728=CARTESIAN_POINT ( 'NONE',  ( 12.25119088044423776, 36.00000000000000711, 5.405483146088369217 ) ) ;
#14735=CARTESIAN_POINT ( 'NONE',  ( 124.5550856135277087, 39.80937500108392868, -13.14518615778179900 ) ) ;
#14736=CARTESIAN_POINT ( 'NONE',  ( 51.85481384221820633, 36.63437500108393152, 5.444914386472304635 ) ) ;
#14738=CARTESIAN_POINT ( 'NONE',  ( 181.8548138422182205, 39.16445312608393436, 0.000000000000000000 ) ) ;
#14741=CARTESIAN_POINT ( 'NONE',  ( 9.295050272127047819, 35.29492187608393294, 9.295050272127046043 ) ) ;
#14742=LINE ( 'NONE', #25314, #23605 ) ;
#14744=CARTESIAN_POINT ( 'NONE',  ( -13.14518615778179189, 39.80937500108392868, 5.444914386472304635 ) ) ;
#14745=CARTESIAN_POINT ( 'NONE',  ( 3.797451868958014565, 54.08938259242987812, 14.99999999999999645 ) ) ;
#14759=CARTESIAN_POINT ( 'NONE',  ( 99.99999999999995737, 81.18750000136559208, -4.458734125000016313 ) ) ;
#14760=CARTESIAN_POINT ( 'NONE',  ( 74.29505027212704249, 38.86679687608393863, -9.295050272127046043 ) ) ;
#14767=CARTESIAN_POINT ( 'NONE',  ( 143.1451861577818079, 32.46718750108393436, -5.444914386472297529 ) ) ;
#14769=CARTESIAN_POINT ( 'NONE',  ( -0.7197605961091591009, 53.51499872091923748, -15.00000000000000000 ) ) ;
#14773=CARTESIAN_POINT ( 'NONE',  ( 55.40115559117954547, 36.43593750216787441, 9.598844408820459861 ) ) ;
#14774=CYLINDRICAL_SURFACE ( 'NONE', #17516, 5.000000000000004441 ) ;
#14775=CARTESIAN_POINT ( 'NONE',  ( 9.598844408820459861, 36.63437500216787157, 9.598844408820456309 ) ) ;
#14779=CARTESIAN_POINT ( 'NONE',  ( 181.8548138422182205, 37.37851562608393863, 0.000000000000000000 ) ) ;
#14781=CARTESIAN_POINT ( 'NONE',  ( 120.7049497278729575, 37.47773437608393010, 9.295050272127047819 ) ) ;
#14783=LINE ( 'NONE', #1166, #18615 ) ;
#14785=CARTESIAN_POINT ( 'NONE',  ( 51.85481384221820633, 40.75195312608393294, 0.000000000000000000 ) ) ;
#14787=CARTESIAN_POINT ( 'NONE',  ( 189.3771271284221314, 36.38632812499999858, 13.57481594606304753 ) ) ;
#14791=CARTESIAN_POINT ( 'NONE',  ( 65.00000000000000000, 39.16445312608392726, 13.14518615778179544 ) ) ;
#14795=CARTESIAN_POINT ( 'NONE',  ( 116.4251840539369738, 39.46210937499999005, 5.622872871577880183 ) ) ;
#14796=CARTESIAN_POINT ( 'NONE',  ( 9.598844408820456309, 39.11484374999999858, -9.598844408820458085 ) ) ;
#14797=CARTESIAN_POINT ( 'NONE',  ( 143.1451861577818079, 39.56132812608393579, -1.609821015232357215E-15 ) ) ;
#14799=CARTESIAN_POINT ( 'NONE',  ( 96.84719886470459471, 83.56250000136560629, -3.152801135295383084 ) ) ;
#14800=VECTOR ( 'NONE', #11542, 1000.000000000000000 ) ;
#14804=CARTESIAN_POINT ( 'NONE',  ( 55.70494972787295751, 35.89023437608393152, -9.295050272127046043 ) ) ;
#14808=ORIENTED_EDGE ( 'NONE', *, *, #9386, .T. ) ;
#14811=CARTESIAN_POINT ( 'NONE',  ( 200.6228728715778686, 36.58476562716787583, 13.57481594606304576 ) ) ;
#14814=CARTESIAN_POINT ( 'NONE',  ( 202.6219635342048662, 54.91641323977498246, 14.99999999999994671 ) ) ;
#14816=CARTESIAN_POINT ( 'NONE',  ( 139.2950502721270425, 39.46210937608393721, 9.295050272127046043 ) ) ;
#14817=CARTESIAN_POINT ( 'NONE',  ( -13.14518615778179544, 39.16445312608393436, 0.000000000000000000 ) ) ;
#14820=CARTESIAN_POINT ( 'NONE',  ( 78.57481594606304043, 36.68398437499999432, -5.622872871577873077 ) ) ;
#14821=CIRCLE ( 'NONE', #17109, 11.57481594606304398 ) ;
#14827=CARTESIAN_POINT ( 'NONE',  ( 95.54126587499996504, 80.68750000136559208, -1.387778780781445676E-14 ) ) ;
#14836=CARTESIAN_POINT ( 'NONE',  ( 97.92893218813451028, 80.31250000273122680, 4.999999999999989342 ) ) ;
#14838=CARTESIAN_POINT ( 'NONE',  ( 130.0000000000000000, 38.12265625216787157, 13.57481594606304576 ) ) ;
#14839=VECTOR ( 'NONE', #27335, 1000.000000000000000 ) ;
#14840=ORIENTED_EDGE ( 'NONE', *, *, #9653, .T. ) ;
#14841=CARTESIAN_POINT ( 'NONE',  ( 65.00000000000000000, 37.77539062608393294, 13.14518615778179544 ) ) ;
#14842=DIRECTION ( 'NONE',  ( 0.000000000000000000, -0.000000000000000000, -1.000000000000000000 ) ) ;
#14843=FACE_OUTER_BOUND ( 'NONE', #8738, .T. ) ;
#14845=EDGE_LOOP ( 'NONE', ( #6928, #17514, #13524, #16380 ) ) ;
#14847=CARTESIAN_POINT ( 'NONE',  ( -8.769389672081235432, 50.37710889402508485, -14.99999999999737099 ) ) ;
#14849=CARTESIAN_POINT ( 'NONE',  ( 116.4251840539369596, 35.59257812716788294, 5.622872871577880183 ) ) ;
#14851=VECTOR ( 'NONE', #19303, 1000.000000000000000 ) ;
#14852=CARTESIAN_POINT ( 'NONE',  ( 70.44491438647230552, 39.41250000108393436, 13.14518615778179189 ) ) ;
#14854=CARTESIAN_POINT ( 'NONE',  ( 99.99999999999995737, 82.37500000273119838, 4.999999999999990230 ) ) ;
#14855=CARTESIAN_POINT ( 'NONE',  ( 189.5550856135277229, 35.04687500108393294, -13.14518615778179900 ) ) ;
#14857=ADVANCED_FACE ( 'NONE', ( #26516 ), #2578, .T. ) ;
#14858=ORIENTED_EDGE ( 'NONE', *, *, #25852, .T. ) ;
#14859=ORIENTED_EDGE ( 'NONE', *, *, #24118, .F. ) ;
#14862=LINE ( 'NONE', #18744, #20747 ) ;
#14867=DIRECTION ( 'NONE',  ( 0.000000000000000000, 0.000000000000000000, -1.000000000000000000 ) ) ;
#14869=CARTESIAN_POINT ( 'NONE',  ( 189.5550856135277229, 40.10703125108393152, 13.14518615778179722 ) ) ;
#14870=CARTESIAN_POINT ( 'NONE',  ( 135.6228728715778971, 32.51679687499999716, 13.57481594606304576 ) ) ;
#14872=VERTEX_POINT ( 'NONE', #12457 ) ;
#14876=CARTESIAN_POINT ( 'NONE',  ( 135.4449143864723055, 35.44375000108393436, 13.14518615778179189 ) ) ;
#14877=CARTESIAN_POINT ( 'NONE',  ( 78.14518615778179367, 37.82500000108392868, -5.444914386472297529 ) ) ;
#14878=CARTESIAN_POINT ( 'NONE',  ( 189.5550856135277229, 31.67343750108393863, -13.14518615778179900 ) ) ;
#14880=CARTESIAN_POINT ( 'NONE',  ( 5.444914386472302859, 35.24531250108393010, 13.14518615778179189 ) ) ;
#14881=CARTESIAN_POINT ( 'NONE',  ( 136.9023785737939534, 51.13402819307182767, -14.99999999999871036 ) ) ;
#14883=ADVANCED_FACE ( 'NONE', ( #1804 ), #7396, .T. ) ;
#14885=CARTESIAN_POINT ( 'NONE',  ( 13.14518615778179544, 36.98164062608393010, -1.609821015232357215E-15 ) ) ;
#14895=EDGE_CURVE ( 'NONE', #19984, #10588, #3861, .T. ) ;
#14897=DIRECTION ( 'NONE',  ( -0.000000000000000000, 1.000000000000000000, -0.000000000000000000 ) ) ;
#14898=CARTESIAN_POINT ( 'NONE',  ( 99.99999999999995737, 83.93750000136560629, 4.458734124999988779 ) ) ;
#14899=CARTESIAN_POINT ( 'NONE',  ( 59.55508561352770158, 38.22187500108393010, -13.14518615778179900 ) ) ;
#14904=CARTESIAN_POINT ( 'NONE',  ( -20.00000000000000355, 80.00000000000000000, -12.99999999999999822 ) ) ;
#14906=CARTESIAN_POINT ( 'NONE',  ( 139.5988444088204687, 39.71015624999999716, 9.598844408820456309 ) ) ;
#14908=CARTESIAN_POINT ( 'NONE',  ( 130.0000000000000000, -7.395377635281828788, -1.503427012513233026E-14 ) ) ;
#14911=CARTESIAN_POINT ( 'NONE',  ( 98.15313185440925281, 80.25000000136559208, -4.458734125000016313 ) ) ;
#14912=CARTESIAN_POINT ( 'NONE',  ( 143.1451861577818079, 37.03125000108393294, -5.444914386472297529 ) ) ;
#14913=CARTESIAN_POINT ( 'NONE',  ( 74.59884440882045453, 38.42031250216787441, -9.598844408820458085 ) ) ;
#14915=CARTESIAN_POINT ( 'NONE',  ( -13.57481594606304576, 36.33671875216787583, 0.000000000000000000 ) ) ;
#14920=CARTESIAN_POINT ( 'NONE',  ( 204.2950502721270425, 36.88242187608393152, 9.295050272127046043 ) ) ;
#14922=EDGE_CURVE ( 'NONE', #5791, #5488, #14742, .T. ) ;
#14923=CARTESIAN_POINT ( 'NONE',  ( 116.8548138422182205, 39.01562500108393294, 5.444914386472304635 ) ) ;
#14924=ORIENTED_EDGE ( 'NONE', *, *, #239, .F. ) ;
#14927=CARTESIAN_POINT ( 'NONE',  ( 55.81982418635200816, 55.00000000000000000, 14.99999999999998401 ) ) ;
#14931=CARTESIAN_POINT ( 'NONE',  ( 204.5988444088204403, 38.32109374999999574, -9.598844408820458085 ) ) ;
#14933=CARTESIAN_POINT ( 'NONE',  ( 78.14518615778179367, 37.72578125108393721, 5.444914386472293977 ) ) ;
#14935=CARTESIAN_POINT ( 'NONE',  ( 66.13716782454086740, 35.99999999999998579, 13.09590655363602707 ) ) ;
#14938=CARTESIAN_POINT ( 'NONE',  ( 2.493653234604083739E-15, 38.02343749999999289, 13.57481594606304576 ) ) ;
#14939=CARTESIAN_POINT ( 'NONE',  ( 135.4449143864723055, 39.41250000108393436, 13.14518615778179189 ) ) ;
#14942=EDGE_LOOP ( 'NONE', ( #15929, #21672, #4, #2292 ) ) ;
#14943=CARTESIAN_POINT ( 'NONE',  ( 101.8468681455906903, 80.00000000136559208, 4.458734124999987891 ) ) ;
#14944=CIRCLE ( 'NONE', #20895, 13.57481594606304398 ) ;
#14948=CARTESIAN_POINT ( 'NONE',  ( 204.5988444088204403, 37.62656250216787157, -9.598844408820458085 ) ) ;
#14949=CARTESIAN_POINT ( 'NONE',  ( 51.85481384221820633, 35.19570312608393436, 0.000000000000000000 ) ) ;
#14951=CARTESIAN_POINT ( 'NONE',  ( 120.8198241863519939, 55.00000000000000000, -15.00000000000000000 ) ) ;
#14954=CARTESIAN_POINT ( 'NONE',  ( -20.00000000000000355, 55.00000000000000000, -9.999999999999998224 ) ) ;
#14956=UNCERTAINTY_MEASURE_WITH_UNIT (LENGTH_MEASURE( 1.000000000000000082E-05 ), #13307, 'distance_accuracy_value', 'NONE');
#14957=CARTESIAN_POINT ( 'NONE',  ( 195.0000000000000000, 36.53515625216787299, 13.57481594606304576 ) ) ;
#14959=FACE_OUTER_BOUND ( 'NONE', #21401, .T. ) ;
#14960=CARTESIAN_POINT ( 'NONE',  ( 130.0000000000000000, 39.75976562608394005, -13.14518615778179544 ) ) ;
#14961=CARTESIAN_POINT ( 'NONE',  ( 9.295050272127047819, 37.08085937608393579, 9.295050272127046043 ) ) ;
#14963=CARTESIAN_POINT ( 'NONE',  ( 135.4449143864723055, 33.65781250108393152, 13.14518615778179189 ) ) ;
#14964=CARTESIAN_POINT ( 'NONE',  ( 78.57481594606304043, 38.27148437500000711, -5.622872871577873077 ) ) ;
#14968=FACE_OUTER_BOUND ( 'NONE', #23248, .T. ) ;
#14971=CARTESIAN_POINT ( 'NONE',  ( 5.622872871577796694, 39.26367187716788010, -13.57481594606312036 ) ) ;
#14974=CARTESIAN_POINT ( 'NONE',  ( -5.444914386472299306, 39.31328125108394289, 13.14518615778179722 ) ) ;
#14976=EDGE_LOOP ( 'NONE', ( #1, #20746, #23843, #13800 ) ) ;
#14980=CARTESIAN_POINT ( 'NONE',  ( 185.4011555911795597, 36.33671874999999574, 9.598844408820459861 ) ) ;
#14981=CARTESIAN_POINT ( 'NONE',  ( 103.5355339059327093, 84.37500000000000000, 3.535533905932726206 ) ) ;
#14982=EDGE_CURVE ( 'NONE', #23612, #28147, #7110, .T. ) ;
#14983=CARTESIAN_POINT ( 'NONE',  ( 208.1451861577817795, 40.20625000108393010, -5.444914386472297529 ) ) ;
#14986=CARTESIAN_POINT ( 'NONE',  ( 97.92893218813451028, 82.93750000273118417, -5.000000000000031974 ) ) ;
#14987=CARTESIAN_POINT ( 'NONE',  ( 139.5988444088204403, 39.90859374999999432, -9.598844408820458085 ) ) ;
#14992=CARTESIAN_POINT ( 'NONE',  ( 116.4251840539369454, 35.49335937716787015, -5.622872871577873077 ) ) ;
#14993=DIRECTION ( 'NONE',  ( 0.000000000000000000, 1.000000000000000000, 0.000000000000000000 ) ) ;
#14995=CARTESIAN_POINT ( 'NONE',  ( 181.8548138422181921, 34.35234375108393579, -5.444914386472297529 ) ) ;
#14997=EDGE_LOOP ( 'NONE', ( #17703, #22320, #7940, #22098, #13694, #11199, #8030, #21001, #1642, #27257 ) ) ;
#14999=LINE ( 'NONE', #23306, #23024 ) ;
#15000=CARTESIAN_POINT ( 'NONE',  ( 103.1528011352953342, 81.06250000136559208, -3.152801135295383084 ) ) ;
#15001=CARTESIAN_POINT ( 'NONE',  ( 185.7049497278729575, 39.66054687608393436, -9.295050272127046043 ) ) ;
#15005=FACE_BOUND ( 'NONE', #8837, .T. ) ;
#15013=CARTESIAN_POINT ( 'NONE',  ( 116.8548138422182063, 35.24531250108393721, 5.444914386472304635 ) ) ;
#15014=CARTESIAN_POINT ( 'NONE',  ( 74.29505027212704249, 33.11210937608393579, -9.295050272127046043 ) ) ;
#15015=CARTESIAN_POINT ( 'NONE',  ( 181.8548138422181921, 37.52734375108393294, -5.444914386472297529 ) ) ;
#15018=CARTESIAN_POINT ( 'NONE',  ( 13.14518615778179544, 36.98164062608393010, -1.609821015232357215E-15 ) ) ;
#15020=CARTESIAN_POINT ( 'NONE',  ( 121.7403884711141018, 50.00000000056351723, -10.79618466886180173 ) ) ;
#15022=CARTESIAN_POINT ( 'NONE',  ( 214.9999999999999716, 75.00000000000000000, -10.00000000000000000 ) ) ;
#15023=CARTESIAN_POINT ( 'NONE',  ( 13.14518615778179544, 38.56914062608393579, -1.609821015232357215E-15 ) ) ;
#15025=DIRECTION ( 'NONE',  ( -0.000000000000000000, -1.000000000000000000, -0.000000000000000000 ) ) ;
#15026=CARTESIAN_POINT ( 'NONE',  ( 64.16107313071965734, 53.50081894914647762, 14.99999999999997868 ) ) ;
#15028=ORIENTED_EDGE ( 'NONE', *, *, #21801, .T. ) ;
#15030=CARTESIAN_POINT ( 'NONE',  ( 77.53142549111997539, 36.00000000000000000, -5.200562670743043903 ) ) ;
#15034=CARTESIAN_POINT ( 'NONE',  ( 55.40115559117954547, 37.82500000216787583, -9.598844408820458085 ) ) ;
#15037=CARTESIAN_POINT ( 'NONE',  ( 95.54126587499996504, 79.68750000136559208, -1.387778780781445676E-14 ) ) ;
#15038=CARTESIAN_POINT ( 'NONE',  ( 78.14518615778179367, 38.71796875108393721, 5.444914386472293977 ) ) ;
#15040=CARTESIAN_POINT ( 'NONE',  ( -8.049105076161786076E-16, 39.56132812608393579, -13.14518615778179544 ) ) ;
#15043=CARTESIAN_POINT ( 'NONE',  ( -15.00000000000000000, 80.00000000000000000, 10.00000000000000000 ) ) ;
#15045=CARTESIAN_POINT ( 'NONE',  ( 120.4011555911795455, 40.10703124999999147, -9.598844408820458085 ) ) ;
#15046=ORIENTED_EDGE ( 'NONE', *, *, #19587, .F. ) ;
#15050=CARTESIAN_POINT ( 'NONE',  ( 130.0000000000000000, 35.59257812608393579, -13.14518615778179544 ) ) ;
#15051=ADVANCED_FACE ( 'NONE', ( #220 ), #10584, .T. ) ;
#15052=CARTESIAN_POINT ( 'NONE',  ( 74.59884440882045453, 35.84062500216786873, 9.598844408820456309 ) ) ;
#15053=CARTESIAN_POINT ( 'NONE',  ( 103.5355339059327093, 83.37500000000000000, 3.535533905932726206 ) ) ;
#15054=CARTESIAN_POINT ( 'NONE',  ( -5.622872871577873077, 37.27929687716787299, 13.57481594606304753 ) ) ;
#15057=DIRECTION ( 'NONE',  ( 0.000000000000000000, 0.000000000000000000, -1.000000000000000000 ) ) ;
#15058=CARTESIAN_POINT ( 'NONE',  ( 181.8548138422182205, 38.17226562608393436, 0.000000000000000000 ) ) ;
#15063=DIRECTION ( 'NONE',  ( -0.000000000000000000, -1.000000000000000000, -0.000000000000000000 ) ) ;
#15067=CARTESIAN_POINT ( 'NONE',  ( 185.4011555911795597, 37.92421874999999432, 9.598844408820459861 ) ) ;
#15070=CARTESIAN_POINT ( 'NONE',  ( 74.29505027212704249, 37.87460937608393152, -9.295050272127046043 ) ) ;
#15071=( BOUNDED_CURVE ( )  B_SPLINE_CURVE ( 2, ( #16179, #22758, #1099, #7342, #11605 ),
 .UNSPECIFIED., .F., .T. ) 
 B_SPLINE_CURVE_WITH_KNOTS ( ( 3, 2, 3 ),
 ( 0.000000000000000000, 0.01041666666666679446, 0.02083333333333358892 ),
 .UNSPECIFIED. ) 
 CURVE ( )  GEOMETRIC_REPRESENTATION_ITEM ( )  RATIONAL_B_SPLINE_CURVE ( ( 1.000000000000000000, 0.9238795325112867385, 1.000000000000000000, 0.9238795325112848511, 1.000000000000001776 ) ) 
 REPRESENTATION_ITEM ( '' )  );
#15073=DIRECTION ( 'NONE',  ( -1.000000000000000000, 0.000000000000000000, 0.000000000000000000 ) ) ;
#15076=CARTESIAN_POINT ( 'NONE',  ( -13.57481594606304753, 36.18789062499999432, -5.622872871577873077 ) ) ;
#15079=CARTESIAN_POINT ( 'NONE',  ( 94.99999999999995737, 84.00000000000000000, -1.387778780781445676E-14 ) ) ;
#15083=CARTESIAN_POINT ( 'NONE',  ( 51.85481384221820633, 36.03906250108394005, 5.444914386472304635 ) ) ;
#15091=CARTESIAN_POINT ( 'NONE',  ( 185.4011555911795597, 36.43593750216787441, 9.598844408820459861 ) ) ;
#15093=CYLINDRICAL_SURFACE ( 'NONE', #13011, 13.57481594606304398 ) ;
#15094=CARTESIAN_POINT ( 'NONE',  ( 193.8612318828944581, 50.00000000043882409, 13.56816686242560266 ) ) ;
#15095=CARTESIAN_POINT ( 'NONE',  ( 116.8548138422182205, 36.78320312608393294, 0.000000000000000000 ) ) ;
#15096=CARTESIAN_POINT ( 'NONE',  ( -5.444914386472299306, 36.93203125108394147, 13.14518615778179722 ) ) ;
#15097=CARTESIAN_POINT ( 'NONE',  ( 143.1451861577818079, 33.85625000108393579, -5.444914386472297529 ) ) ;
#15098=CARTESIAN_POINT ( 'NONE',  ( 59.37712712842213136, 33.21132812499999432, 13.57481594606304753 ) ) ;
#15099=CARTESIAN_POINT ( 'NONE',  ( -13.14518615778179544, 40.75195312608393294, 0.000000000000000000 ) ) ;
#15101=CARTESIAN_POINT ( 'NONE',  ( 197.2323271553383108, 36.00000000000000711, 12.98409812936874630 ) ) ;
#15106=CARTESIAN_POINT ( 'NONE',  ( 101.8468681455907046, 80.37500000136563472, -4.458734125000016313 ) ) ;
#15108=CARTESIAN_POINT ( 'NONE',  ( 9.295050272127046043, 38.86679687608393863, -9.295050272127046043 ) ) ;
#15111=VERTEX_POINT ( 'NONE', #6904 ) ;
#15113=CARTESIAN_POINT ( 'NONE',  ( 124.3771271284220319, 37.27929687716785878, 13.57481594606295161 ) ) ;
#15116=CARTESIAN_POINT ( 'NONE',  ( 204.2950502721270425, 37.67617187608393436, 9.295050272127046043 ) ) ;
#15126=CARTESIAN_POINT ( 'NONE',  ( 139.5988444088204687, 32.66562500216787157, 9.598844408820456309 ) ) ;
#15128=DIRECTION ( 'NONE',  ( 0.000000000000000000, 0.000000000000000000, 1.000000000000000000 ) ) ;
#15130=CARTESIAN_POINT ( 'NONE',  ( 208.1451861577818079, 34.00507812608393721, -1.609821015232357215E-15 ) ) ;
#15137=EDGE_CURVE ( 'NONE', #12494, #17873, #24299, .T. ) ;
#15139=CARTESIAN_POINT ( 'NONE',  ( 65.00000000000000000, 39.16445312608392726, 13.14518615778179544 ) ) ;
#15140=CARTESIAN_POINT ( 'NONE',  ( 104.4587341249999781, 81.87500000136560629, 1.846868145590721655 ) ) ;
#15141=CARTESIAN_POINT ( 'NONE',  ( 204.2950502721270425, 38.46992187608393010, 9.295050272127046043 ) ) ;
#15144=DIRECTION ( 'NONE',  ( 0.000000000000000000, 0.000000000000000000, -1.000000000000000000 ) ) ;
#15145=CARTESIAN_POINT ( 'NONE',  ( 70.62287287157778337, 39.95820312499999716, -13.57481594606312036 ) ) ;
#15147=ORIENTED_EDGE ( 'NONE', *, *, #19113, .F. ) ;
#15148=( BOUNDED_CURVE ( )  B_SPLINE_CURVE ( 2, ( #731, #11673, #14240, #18394, #22961, #880, #7405, #16098, #27100, #7697, #3423, #16248, #24945, #5431, #22820, #16389, #1294, #12090, #23644, #25771, #6251, #4119, #23231, #8243, #18807, #27784, #5980, #5712, #12645, #16932, #25366, #14923, #12784, #18940, #10513, #21501, #14378, #1437, #18676, #12370, #3568, #21371, #12499, #8109, #27922, #16669, #16530, #25501, #23366, #27649, #1981, #25632, #3708, #17068, #6115, #8383, #23502, #1576, #27377, #23094, #21088, #12226, #14781, #20954, #7969, #10094, #1850, #3982, #16803, #14647, #5845, #7837, #27512, #14515, #10230, #19220, #25223, #3838, #1711, #21227, #10372, #19079, #25917, #24201, #13488, #8804, #8665, #4681, #6391, #28197, #4397, #19499, #26488 ),
 .UNSPECIFIED., .F., .F. ) 
 B_SPLINE_CURVE_WITH_KNOTS ( ( 3, 2, 2, 2, 2, 2, 2, 2, 2, 2, 2, 2, 2, 2, 2, 2, 2, 2, 2, 2, 2, 2, 2, 2, 2, 2, 2, 2, 2, 2, 2, 2, 2, 2, 2, 2, 2, 2, 2, 2, 2, 2, 2, 2, 2, 2, 3 ),
 ( 0.000000000000000000, 0.01041666666666666609, 0.02083333333333333218, 0.03125000000000000000, 0.04166666666666666435, 0.05208333333333333565, 0.06250000000000000000, 0.07291666666666667129, 0.08333333333333332871, 0.09375000000000000000, 0.1041666666666666713, 0.1145833333333333287, 0.1250000000000000000, 0.1354166666666666574, 0.1458333333333333426, 0.1562500000000000278, 0.1666666666666666574, 0.1770833333333333426, 0.1875000000000000000, 0.1979166666666666574, 0.2083333333333333426, 0.2187499999999999722, 0.2291666666666666574, 0.2395833333333333426, 0.2500000000000000000, 0.2604166666666666852, 0.2708333333333333148, 0.2812500000000000000, 0.2916666666666666852, 0.3020833333333333148, 0.3125000000000000555, 0.3229166666666666852, 0.3333333333333333148, 0.3437500000000000000, 0.3541666666666666852, 0.3645833333333333148, 0.3750000000000000000, 0.3854166666666666852, 0.3958333333333333148, 0.4062500000000000000, 0.4166666666666666852, 0.4270833333333333148, 0.4374999999999999445, 0.4479166666666666852, 0.4583333333333333148, 0.4687500000000000000, 0.4779971559588573893 ),
 .UNSPECIFIED. ) 
 CURVE ( )  GEOMETRIC_REPRESENTATION_ITEM ( )  RATIONAL_B_SPLINE_CURVE ( ( 1.000000000000000000, 0.9238795325112867385, 1.000000000000000000, 0.9238795325112867385, 1.000000000000000000, 0.9238795325112867385, 1.000000000000000000, 0.9238795325112867385, 1.000000000000000000, 0.9238795325112867385, 1.000000000000000000, 0.9238795325112867385, 1.000000000000000000, 0.9238795325112867385, 1.000000000000000000, 0.9238795325112867385, 1.000000000000000000, 0.9238795325112867385, 1.000000000000000000, 0.9238795325112867385, 1.000000000000000000, 0.9238795325112867385, 1.000000000000000000, 0.9238795325112867385, 1.000000000000000000, 0.9238795325112867385, 1.000000000000000000, 0.9238795325112867385, 1.000000000000000000, 0.9238795325112867385, 1.000000000000000000, 0.9238795325112867385, 1.000000000000000000, 0.9238795325112867385, 1.000000000000000000, 0.9238795325112867385, 1.000000000000000000, 0.9238795325112867385, 1.000000000000000000, 0.9238795325112867385, 1.000000000000000000, 0.9238795325112867385, 1.000000000000000000, 0.9238795325112867385, 1.000000000000000000, 0.9238795325112867385, 1.000000000000000000, 0.9238795325112867385, 1.000000000000000000, 0.9238795325112867385, 1.000000000000000000, 0.9238795325112867385, 1.000000000000000000, 0.9238795325112867385, 1.000000000000000000, 0.9238795325112867385, 1.000000000000000000, 0.9238795325112867385, 1.000000000000000000, 0.9238795325112867385, 1.000000000000000000, 0.9238795325112867385, 1.000000000000000000, 0.9238795325112867385, 1.000000000000000000, 0.9238795325112867385, 1.000000000000000000, 0.9238795325112867385, 1.000000000000000000, 0.9238795325112867385, 1.000000000000000000, 0.9238795325112867385, 1.000000000000000000, 0.9238795325112867385, 1.000000000000000000, 0.9238795325112867385, 1.000000000000000000, 0.9238795325112867385, 1.000000000000000000, 0.9238795325112867385, 1.000000000000000000, 0.9238795325112867385, 1.000000000000000000, 0.9238795325112867385, 1.000000000000000000, 0.9238795325112867385, 1.000000000000000000, 0.9238795325112867385, 1.000000000000000000, 0.9238795325112867385, 1.000000000000000000, 0.9324258078851906939, 0.9848264816800322841 ) ) 
 REPRESENTATION_ITEM ( '' )  );
#15152=CARTESIAN_POINT ( 'NONE',  ( 139.2950502721270425, 34.89804687608393863, -9.295050272127046043 ) ) ;
#15153=CARTESIAN_POINT ( 'NONE',  ( 70.44491438647230552, 34.74921875108394431, -13.14518615778179900 ) ) ;
#15154=CARTESIAN_POINT ( 'NONE',  ( 204.2950502721270425, 37.08085937608393579, 9.295050272127046043 ) ) ;
#15156=CARTESIAN_POINT ( 'NONE',  ( 6.944423797152705191, 31.55306878032414986, -11.16113333171310451 ) ) ;
#15157=CARTESIAN_POINT ( 'NONE',  ( 181.8473230904129139, 36.00000000000000711, 0.5874252385153372336 ) ) ;
#15161=CARTESIAN_POINT ( 'NONE',  ( -8.049105076161786076E-16, 36.38632812608393152, -13.14518615778179544 ) ) ;
#15164=CARTESIAN_POINT ( 'NONE',  ( 59.63450343195739833, 54.48174559707608466, 14.99999999999998046 ) ) ;
#15166=EDGE_CURVE ( 'NONE', #22369, #2045, #13872, .T. ) ;
#15167=DIRECTION ( 'NONE',  ( -0.000000000000000000, 1.000000000000000000, -0.000000000000000000 ) ) ;
#15169=VERTEX_POINT ( 'NONE', #22599 ) ;
#15172=CARTESIAN_POINT ( 'NONE',  ( 123.5491206573346830, 50.00000000106874154, 11.97362904075384016 ) ) ;
#15175=CARTESIAN_POINT ( 'NONE',  ( 98.15313185440925281, 81.87500000136559208, 4.458734124999987891 ) ) ;
#15176=CARTESIAN_POINT ( 'NONE',  ( 74.29505027212704249, 36.28710937608393294, 9.295050272127046043 ) ) ;
#15180=FACE_OUTER_BOUND ( 'NONE', #14976, .T. ) ;
#15181=DIRECTION ( 'NONE',  ( 0.000000000000000000, 1.000000000000000000, 0.000000000000000000 ) ) ;
#15182=CARTESIAN_POINT ( 'NONE',  ( 104.9999999999999716, 82.50000000000000000, -1.449011120738813565E-14 ) ) ;
#15183=CARTESIAN_POINT ( 'NONE',  ( 143.5748159460630404, 37.37851562499999858, 5.622872871577869525 ) ) ;
#15189=CARTESIAN_POINT ( 'NONE',  ( 143.1451861577818079, 36.23750000108393010, -5.444914386472297529 ) ) ;
#15190=CARTESIAN_POINT ( 'NONE',  ( 78.57481594606305464, 34.35234375216787583, -1.662435489736055892E-15 ) ) ;
#15192=CARTESIAN_POINT ( 'NONE',  ( -5.622872871577873077, 33.80664062716786589, -13.57481594606304753 ) ) ;
#15197=CARTESIAN_POINT ( 'NONE',  ( 195.0000000000000000, 37.18007812608393436, -13.14518615778179544 ) ) ;
#15198=CARTESIAN_POINT ( 'NONE',  ( 120.8198241863519939, 55.00000000000000000, 9.999999999999969802 ) ) ;
#15200=CARTESIAN_POINT ( 'NONE',  ( 181.4251840539369596, 37.87460937716787868, -5.622872871577872189 ) ) ;
#15202=CARTESIAN_POINT ( 'NONE',  ( 204.5988444088204403, 36.73359374999999716, -9.598844408820458085 ) ) ;
#15208=CARTESIAN_POINT ( 'NONE',  ( 200.6228728715778686, 35.69179687499999432, 13.57481594606304576 ) ) ;
#15209=CARTESIAN_POINT ( 'NONE',  ( 65.00000000000000000, 40.00781250000000000, -13.57481594606304576 ) ) ;
#15210=CARTESIAN_POINT ( 'NONE',  ( 70.44491438647230552, 36.03906250108394005, 13.14518615778179189 ) ) ;
#15212=CARTESIAN_POINT ( 'NONE',  ( 99.99999999999995737, 85.00000000000000000, -1.387778780781445676E-14 ) ) ;
#15215=DIRECTION ( 'NONE',  ( 0.000000000000000000, -1.000000000000000000, 0.000000000000000000 ) ) ;
#15216=CARTESIAN_POINT ( 'NONE',  ( 5.622872871577878406, 35.69179687499999432, 13.57481594606304576 ) ) ;
#15217=CARTESIAN_POINT ( 'NONE',  ( 130.0000000000000000, 40.55351562608393579, -13.14518615778179544 ) ) ;
#15218=EDGE_CURVE ( 'NONE', #11953, #4933, #13196, .T. ) ;
#15220=CARTESIAN_POINT ( 'NONE',  ( 99.99999999999995737, 80.93750000136559208, 4.458734124999988779 ) ) ;
#15221=CIRCLE ( 'NONE', #3876, 5.000000000000000000 ) ;
#15223=CARTESIAN_POINT ( 'NONE',  ( 64.82771023522410303, 35.99999999999999289, -13.51468191220837944 ) ) ;
#15225=EDGE_CURVE ( 'NONE', #10588, #18001, #21173, .T. ) ;
#15227=CARTESIAN_POINT ( 'NONE',  ( 78.14518615778179367, 36.43593750108392726, -5.444914386472297529 ) ) ;
#15229=CARTESIAN_POINT ( 'NONE',  ( 143.5748159460630688, 39.16445312716788152, -5.622872871577873966 ) ) ;
#15232=CARTESIAN_POINT ( 'NONE',  ( 99.99999999999995737, 81.87500000273119838, -5.000000000000018652 ) ) ;
#15234=CARTESIAN_POINT ( 'NONE',  ( 195.0000000000000000, 36.93203125216787441, -13.57481594606304576 ) ) ;
#15236=CARTESIAN_POINT ( 'NONE',  ( -20.00000000000000000, 75.00000000000000000, 15.00000000000000178 ) ) ;
#15239=CARTESIAN_POINT ( 'NONE',  ( 13.14518615778179900, 37.92421875108392726, 5.444914386472293977 ) ) ;
#15240=CARTESIAN_POINT ( 'NONE',  ( 116.8548138422182063, 34.94765625108392726, -5.444914386472297529 ) ) ;
#15241=CARTESIAN_POINT ( 'NONE',  ( 78.57481594606304043, 34.99726562500000426, 5.622872871577869525 ) ) ;
#15249=VECTOR ( 'NONE', #2304, 1000.000000000000000 ) ;
#15251=CARTESIAN_POINT ( 'NONE',  ( 96.84719886470459471, 80.81250000136559208, 3.152801135295355994 ) ) ;
#15253=CARTESIAN_POINT ( 'NONE',  ( 9.295050272127047819, 37.08085937608393579, 9.295050272127046043 ) ) ;
#15254=EDGE_CURVE ( 'NONE', #26290, #9425, #16424, .T. ) ;
#15256=ORIENTED_EDGE ( 'NONE', *, *, #2215, .T. ) ;
#15260=CARTESIAN_POINT ( 'NONE',  ( 195.0000000000000000, 38.37070312608393152, 13.14518615778179544 ) ) ;
#15261=ORIENTED_EDGE ( 'NONE', *, *, #11058, .F. ) ;
#15262=CARTESIAN_POINT ( 'NONE',  ( 65.00000000000000000, 36.58476562608393579, -13.14518615778179544 ) ) ;
#15264=CARTESIAN_POINT ( 'NONE',  ( 66.60527187657659454, 53.60388944777320575, -14.99999999999999822 ) ) ;
#15268=CIRCLE ( 'NONE', #1648, 5.000000000000004441 ) ;
#15270=CARTESIAN_POINT ( 'NONE',  ( 135.4449143864723055, 40.00781250108393294, 13.14518615778179189 ) ) ;
#15271=FACE_OUTER_BOUND ( 'NONE', #9575, .T. ) ;
#15273=( BOUNDED_SURFACE ( )  B_SPLINE_SURFACE ( 1, 2, ( 
 ( #15792, #18366, #27216, #2835, #9804, #7524, #7670, #16071, #5404, #20220, #9378, #4980, #20790, #22794, #853, #14215, #3122, #22933, #9663, #18075, #13924, #16363, #26789, #24779, #3263, #3394, #12065, #7234, #1271, #15925, #9935, #18650, #13782, #5260, #7093, #13646, #26934, #22361, #2969, #11503, #12759, #18916, #1412, #7946, #19196, #25608, #27490, #1686, #25478, #27625, #20928, #12476, #14759, #19052, #10071, #8220, #18783, #23066, #21065, #10628, #7813, #16643, #8083, #5685, #16778, #3816, #6092, #27899, #14624, #3959, #12619, #5956, #8359, #21344, #25335, #23479, #3544, #27761, #27355, #5821, #17045 ),
 ( #1823, #23342, #10488, #12347, #3683, #14491, #25749, #21203, #6231, #10345, #1553, #16505, #14898, #16910, #23619, #12201, #4096, #21479, #14351, #1959, #25199, #23208, #10206, #8645, #24313, #11043, #21620, #4799, #26464, #6499, #21910, #382, #17761, #21766, #19333, #15464, #8780, #19898, #4232, #2518, #13171, #25895, #17610, #17468, #10905, #15175, #17334, #13457, #19752, #2096, #22183, #6918, #23894, #2385, #9066, #15611, #26028, #2243, #12890, #2663, #10764, #11180, #26170, #15321, #13317, #235, #28036, #8922, #19475, #28174, #26318, #19614, #6779, #8503, #99, #4373, #17188, #13029, #24178, #6365, #15037 ) ),
 .UNSPECIFIED., .F., .F., .F. ) 
 B_SPLINE_SURFACE_WITH_KNOTS ( ( 2, 2 ),
 ( 3, 2, 2, 2, 2, 2, 2, 2, 2, 2, 2, 2, 2, 2, 2, 2, 2, 2, 2, 2, 2, 2, 2, 2, 2, 2, 2, 2, 2, 2, 2, 2, 2, 2, 2, 2, 2, 2, 2, 2, 3 ),
 ( 0.000000000000000000, 1.000000000000000000 ),
 ( 0.000000000000000000, 0.02500000000000000139, 0.05000000000000000278, 0.07499999999999999722, 0.1000000000000000056, 0.1250000000000000000, 0.1499999999999999944, 0.1749999999999999889, 0.2000000000000000111, 0.2250000000000000056, 0.2500000000000000000, 0.2750000000000000222, 0.2999999999999999889, 0.3250000000000000111, 0.3499999999999999778, 0.3750000000000000000, 0.4000000000000000222, 0.4249999999999999889, 0.4500000000000000111, 0.4749999999999999778, 0.5000000000000000000, 0.5250000000000000222, 0.5500000000000000444, 0.5749999999999999556, 0.5999999999999999778, 0.6250000000000000000, 0.6500000000000000222, 0.6750000000000000444, 0.6999999999999999556, 0.7249999999999999778, 0.7500000000000000000, 0.7750000000000000222, 0.8000000000000000444, 0.8249999999999999556, 0.8499999999999999778, 0.8750000000000000000, 0.9000000000000000222, 0.9250000000000000444, 0.9499999999999999556, 0.9749999999999999778, 1.000000000000000000 ),
 .UNSPECIFIED. ) 
 GEOMETRIC_REPRESENTATION_ITEM ( )  RATIONAL_B_SPLINE_SURFACE ( (
 ( 1.000000000000000000, 0.9238795325112867385, 1.000000000000000000, 0.9238795325112867385, 1.000000000000000000, 0.9238795325112867385, 1.000000000000000000, 0.9238795325112867385, 1.000000000000000000, 0.9238795325112867385, 1.000000000000000000, 0.9238795325112867385, 1.000000000000000000, 0.9238795325112867385, 1.000000000000000000, 0.9238795325112867385, 1.000000000000000000, 0.9238795325112867385, 1.000000000000000000, 0.9238795325112867385, 1.000000000000000000, 0.9238795325112867385, 1.000000000000000000, 0.9238795325112867385, 1.000000000000000000, 0.9238795325112867385, 1.000000000000000000, 0.9238795325112867385, 1.000000000000000000, 0.9238795325112867385, 1.000000000000000000, 0.9238795325112867385, 1.000000000000000000, 0.9238795325112867385, 1.000000000000000000, 0.9238795325112867385, 1.000000000000000000, 0.9238795325112867385, 1.000000000000000000, 0.9238795325112867385, 1.000000000000000000, 0.9238795325112867385, 1.000000000000000000, 0.9238795325112867385, 1.000000000000000000, 0.9238795325112867385, 1.000000000000000000, 0.9238795325112867385, 1.000000000000000000, 0.9238795325112867385, 1.000000000000000000, 0.9238795325112867385, 1.000000000000000000, 0.9238795325112867385, 1.000000000000000000, 0.9238795325112867385, 1.000000000000000000, 0.9238795325112867385, 1.000000000000000000, 0.9238795325112867385, 1.000000000000000000, 0.9238795325112867385, 1.000000000000000000, 0.9238795325112867385, 1.000000000000000000, 0.9238795325112867385, 1.000000000000000000, 0.9238795325112867385, 1.000000000000000000, 0.9238795325112867385, 1.000000000000000000, 0.9238795325112867385, 1.000000000000000000, 0.9238795325112867385, 1.000000000000000000, 0.9238795325112867385, 1.000000000000000000, 0.9238795325112867385, 1.000000000000000000, 0.9238795325112867385, 1.000000000000000000),
 ( 1.000000000000000000, 0.9238795325112867385, 1.000000000000000000, 0.9238795325112867385, 1.000000000000000000, 0.9238795325112867385, 1.000000000000000000, 0.9238795325112867385, 1.000000000000000000, 0.9238795325112867385, 1.000000000000000000, 0.9238795325112867385, 1.000000000000000000, 0.9238795325112867385, 1.000000000000000000, 0.9238795325112867385, 1.000000000000000000, 0.9238795325112867385, 1.000000000000000000, 0.9238795325112867385, 1.000000000000000000, 0.9238795325112867385, 1.000000000000000000, 0.9238795325112867385, 1.000000000000000000, 0.9238795325112867385, 1.000000000000000000, 0.9238795325112867385, 1.000000000000000000, 0.9238795325112867385, 1.000000000000000000, 0.9238795325112867385, 1.000000000000000000, 0.9238795325112867385, 1.000000000000000000, 0.9238795325112867385, 1.000000000000000000, 0.9238795325112867385, 1.000000000000000000, 0.9238795325112867385, 1.000000000000000000, 0.9238795325112867385, 1.000000000000000000, 0.9238795325112867385, 1.000000000000000000, 0.9238795325112867385, 1.000000000000000000, 0.9238795325112867385, 1.000000000000000000, 0.9238795325112867385, 1.000000000000000000, 0.9238795325112867385, 1.000000000000000000, 0.9238795325112867385, 1.000000000000000000, 0.9238795325112867385, 1.000000000000000000, 0.9238795325112867385, 1.000000000000000000, 0.9238795325112867385, 1.000000000000000000, 0.9238795325112867385, 1.000000000000000000, 0.9238795325112867385, 1.000000000000000000, 0.9238795325112867385, 1.000000000000000000, 0.9238795325112867385, 1.000000000000000000, 0.9238795325112867385, 1.000000000000000000, 0.9238795325112867385, 1.000000000000000000, 0.9238795325112867385, 1.000000000000000000, 0.9238795325112867385, 1.000000000000000000, 0.9238795325112867385, 1.000000000000000000, 0.9238795325112867385, 1.000000000000000000) ) ) 
 REPRESENTATION_ITEM ( '' )  SURFACE ( )  );
#15275=CARTESIAN_POINT ( 'NONE',  ( 1.662435489736055498E-15, -7.395377635281828788, -13.57481594606304398 ) ) ;
#15276=CARTESIAN_POINT ( 'NONE',  ( 208.1451861577818079, 33.21132812608393436, -1.609821015232357215E-15 ) ) ;
#15277=EDGE_CURVE ( 'NONE', #7991, #4458, #14439, .T. ) ;
#15278=ORIENTED_EDGE ( 'NONE', *, *, #14192, .F. ) ;
#15285=CARTESIAN_POINT ( 'NONE',  ( 104.4587341249999781, 82.00000000136560629, -1.846868145590750521 ) ) ;
#15286=CARTESIAN_POINT ( 'NONE',  ( 204.2950502721270425, 39.46210937608393010, -9.295050272127046043 ) ) ;
#15288=CARTESIAN_POINT ( 'NONE',  ( 185.8198241863519797, 55.00000000000001421, 14.99999999999995026 ) ) ;
#15289=CIRCLE ( 'NONE', #18523, 5.000000000000004441 ) ;
#15290=DIRECTION ( 'NONE',  ( -0.000000000000000000, 1.000000000000000000, -0.000000000000000000 ) ) ;
#15291=CARTESIAN_POINT ( 'NONE',  ( 200.4449143864723055, 40.50390625108394005, -13.14518615778179722 ) ) ;
#15298=CARTESIAN_POINT ( 'NONE',  ( 143.1451861577818079, 36.43593750108392726, -5.444914386472297529 ) ) ;
#15299=CARTESIAN_POINT ( 'NONE',  ( 65.00000000000000000, 33.60820312608392868, 13.14518615778179544 ) ) ;
#15300=CARTESIAN_POINT ( 'NONE',  ( 181.8548138422181921, 36.03906250108394005, 5.444914386472304635 ) ) ;
#15301=ORIENTED_EDGE ( 'NONE', *, *, #13687, .F. ) ;
#15303=CARTESIAN_POINT ( 'NONE',  ( 5.444914386472302859, 32.86406250108392868, 13.14518615778179189 ) ) ;
#15304=CARTESIAN_POINT ( 'NONE',  ( 122.3780364657951907, 54.91641323977497535, -15.00000000000000000 ) ) ;
#15305=AXIS2_PLACEMENT_3D ( 'NONE', #26070, #17374, #6539 ) ;
#15306=CARTESIAN_POINT ( 'NONE',  ( 5.622872871577928144, 39.16445312500000142, -13.57481594606299247 ) ) ;
#15307=CARTESIAN_POINT ( 'NONE',  ( 99.99999999999995737, 85.00000000000000000, 4.999999999999990230 ) ) ;
#15309=CARTESIAN_POINT ( 'NONE',  ( -13.14518615778179544, 36.58476562608393579, 0.000000000000000000 ) ) ;
#15311=CARTESIAN_POINT ( 'NONE',  ( 103.5355339059327093, 79.50000000273119838, 3.535533905932726206 ) ) ;
#15312=FACE_OUTER_BOUND ( 'NONE', #436, .T. ) ;
#15318=CARTESIAN_POINT ( 'NONE',  ( 128.8612318829052299, 50.00000000043912962, 13.56816686242597392 ) ) ;
#15321=CARTESIAN_POINT ( 'NONE',  ( 95.54126587499995082, 80.75000000136560629, 1.846868145590724986 ) ) ;
#15322=CARTESIAN_POINT ( 'NONE',  ( 55.70494972787295751, 35.09648437608393579, -9.295050272127046043 ) ) ;
#15325=CARTESIAN_POINT ( 'NONE',  ( -13.14518615778179722, 38.91640625108393436, -5.444914386472297529 ) ) ;
#15326=CARTESIAN_POINT ( 'NONE',  ( 99.99999999999995737, 80.37500000273119838, 4.999999999999990230 ) ) ;
#15329=CARTESIAN_POINT ( 'NONE',  ( 116.4251840539369454, 36.98164062499999005, -5.622872871577873077 ) ) ;
#15330=VERTEX_POINT ( 'NONE', #12294 ) ;
#15331=DIRECTION ( 'NONE',  ( 0.000000000000000000, 0.000000000000000000, 1.000000000000000000 ) ) ;
#15334=CARTESIAN_POINT ( 'NONE',  ( 116.8548138422182205, 36.58476562608393579, 0.000000000000000000 ) ) ;
#15335=CARTESIAN_POINT ( 'NONE',  ( 70.62287287157788285, 34.20351562716788862, 13.57481594606304576 ) ) ;
#15336=ADVANCED_FACE ( 'NONE', ( #14712 ), #20599, .F. ) ;
#15338=CARTESIAN_POINT ( 'NONE',  ( -5.622872871577873077, 34.10429687716786873, 13.57481594606304753 ) ) ;
#15341=CARTESIAN_POINT ( 'NONE',  ( 195.0000000000000000, 35.59257812608393579, -13.14518615778179544 ) ) ;
#15344=DIRECTION ( 'NONE',  ( 3.469446951953613696E-16, 0.000000000000000000, -1.000000000000000000 ) ) ;
#15346=DIRECTION ( 'NONE',  ( -1.000000000000000000, 2.507721281754145042E-33, 7.228014483236696740E-18 ) ) ;
#15347=CARTESIAN_POINT ( 'NONE',  ( 131.5010191243050031, 53.60014735326987534, 14.99999999999996803 ) ) ;
#15352=CARTESIAN_POINT ( 'NONE',  ( 185.4011555911795597, 33.95546874999999432, 9.598844408820459861 ) ) ;
#15355=CARTESIAN_POINT ( 'NONE',  ( 143.5748159460630688, 36.58476562499999574, 5.622872871577868636 ) ) ;
#15356=CARTESIAN_POINT ( 'NONE',  ( 51.85481384221819923, 34.15390625108393863, -5.444914386472297529 ) ) ;
#15361=CARTESIAN_POINT ( 'NONE',  ( 13.57481594606304931, 34.99726562500000426, 5.622872871577869525 ) ) ;
#15362=CARTESIAN_POINT ( 'NONE',  ( 143.1451861577818079, 36.43593750108392726, -5.444914386472297529 ) ) ;
#15363=VERTEX_POINT ( 'NONE', #1497 ) ;
#15364=CARTESIAN_POINT ( 'NONE',  ( 102.0710678118654329, 84.31250000000001421, 4.999999999999989342 ) ) ;
#15365=CARTESIAN_POINT ( 'NONE',  ( 97.92893218813451028, 80.93750000273119838, -5.000000000000018652 ) ) ;
#15367=CARTESIAN_POINT ( 'NONE',  ( 53.85445312690458763, 36.00000000000000000, -7.260818043107227560 ) ) ;
#15370=CARTESIAN_POINT ( 'NONE',  ( 65.00000000000000000, 33.80664062608393294, 13.14518615778179544 ) ) ;
#15371=ORIENTED_EDGE ( 'NONE', *, *, #18711, .F. ) ;
#15373=CARTESIAN_POINT ( 'NONE',  ( 143.5748159460630688, 39.06523437716786873, 5.622872871577868636 ) ) ;
#15375=EDGE_CURVE ( 'NONE', #15622, #2100, #7514, .T. ) ;
#15379=CARTESIAN_POINT ( 'NONE',  ( 200.6228728715778686, 36.08867187716787583, -13.57481594606304753 ) ) ;
#15382=CARTESIAN_POINT ( 'NONE',  ( 130.0000000000000000, 37.77539062608393294, 13.14518615778179544 ) ) ;
#15384=CARTESIAN_POINT ( 'NONE',  ( 5.444914386472302859, 39.41250000108393436, 13.14518615778179189 ) ) ;
#15385=CARTESIAN_POINT ( 'NONE',  ( 116.8548138422182063, 34.25312500108393010, 5.444914386472304635 ) ) ;
#15386=CARTESIAN_POINT ( 'NONE',  ( 51.42518405393695957, 35.49335937499999005, 5.622872871577880183 ) ) ;
#15391=CARTESIAN_POINT ( 'NONE',  ( 185.4011555911795597, 37.13046874999999147, 9.598844408820459861 ) ) ;
#15395=CARTESIAN_POINT ( 'NONE',  ( 13.57481594606304753, 39.16445312716788152, -5.622872871577873966 ) ) ;
#15396=CARTESIAN_POINT ( 'NONE',  ( 214.9999999999999716, 55.00000000000000000, 9.999999999999946709 ) ) ;
#15398=CARTESIAN_POINT ( 'NONE',  ( -9.295050272127046043, 35.09648437608393579, -9.295050272127046043 ) ) ;
#15404=CARTESIAN_POINT ( 'NONE',  ( 200.4449143864723055, 40.30546875108393579, -13.14518615778179900 ) ) ;
#15405=ORIENTED_EDGE ( 'NONE', *, *, #18628, .F. ) ;
#15407=LINE ( 'NONE', #10984, #22920 ) ;
#15408=CARTESIAN_POINT ( 'NONE',  ( 187.3834746745192206, 54.91574374957786375, -15.00000000000000178 ) ) ;
#15416=CARTESIAN_POINT ( 'NONE',  ( 124.3771271284221314, 31.72304687716787441, 13.57481594606304753 ) ) ;
#15417=DIRECTION ( 'NONE',  ( 0.000000000000000000, 1.000000000000000000, 0.000000000000000000 ) ) ;
#15419=CARTESIAN_POINT ( 'NONE',  ( 51.85481384221820633, 38.42031250108393436, 5.444914386472304635 ) ) ;
#15421=CARTESIAN_POINT ( 'NONE',  ( 185.7049497278729575, 34.50117187608393721, 9.295050272127047819 ) ) ;
#15422=EDGE_CURVE ( 'NONE', #15363, #7335, #5537, .T. ) ;
#15423=ORIENTED_EDGE ( 'NONE', *, *, #3286, .T. ) ;
#15428=CARTESIAN_POINT ( 'NONE',  ( 99.99999999999995737, 81.68750000136559208, 4.458734124999988779 ) ) ;
#15429=CARTESIAN_POINT ( 'NONE',  ( 195.0000000000000000, 37.97382812608393721, -13.14518615778179544 ) ) ;
#15434=CARTESIAN_POINT ( 'NONE',  ( 74.59884440882045453, 39.71015624999999716, 9.598844408820456309 ) ) ;
#15436=VERTEX_POINT ( 'NONE', #11698 ) ;
#15439=ORIENTED_EDGE ( 'NONE', *, *, #18240, .F. ) ;
#15440=CARTESIAN_POINT ( 'NONE',  ( 120.7049497278729575, 36.68398437608393436, -9.295050272127046043 ) ) ;
#15441=CARTESIAN_POINT ( 'NONE',  ( 51.85481384221820633, 34.25312500108393010, 5.444914386472304635 ) ) ;
#15442=CIRCLE ( 'NONE', #25098, 4.999999999999999112 ) ;
#15443=CARTESIAN_POINT ( 'NONE',  ( 204.2950502721270425, 38.07304687608393579, -9.295050272127046043 ) ) ;
#15444=ORIENTED_EDGE ( 'NONE', *, *, #12266, .T. ) ;
#15446=CARTESIAN_POINT ( 'NONE',  ( 13.14518615778179544, 32.21914062608393436, -1.609821015232357215E-15 ) ) ;
#15447=CARTESIAN_POINT ( 'NONE',  ( 133.1146977455429692, 53.90847045361285694, -15.00000000000000000 ) ) ;
#15448=( BOUNDED_CURVE ( )  B_SPLINE_CURVE ( 2, ( #12514, #1724, #27936, #14795, #25787, #12660, #23246, #12385, #21387 ),
 .UNSPECIFIED., .F., .F. ) 
 B_SPLINE_CURVE_WITH_KNOTS ( ( 3, 2, 2, 2, 3 ),
 ( 0.1458333333333336757, 0.1562500000000002776, 0.1666666666666669072, 0.1770833333333335369, 0.1875000000000001388 ),
 .UNSPECIFIED. ) 
 CURVE ( )  GEOMETRIC_REPRESENTATION_ITEM ( )  RATIONAL_B_SPLINE_CURVE ( ( 0.9999999999999975575, 0.9238795325112891810, 1.000000000000000000, 0.9238795325112867385, 1.000000000000000000, 0.9238795325112867385, 1.000000000000000000, 0.9238795325112857393, 1.000000000000001110 ) ) 
 REPRESENTATION_ITEM ( '' )  );
#15449=ADVANCED_FACE ( 'NONE', ( #13700 ), #11557, .T. ) ;
#15451=CARTESIAN_POINT ( 'NONE',  ( 130.0000000000000000, 40.10703125216787157, -13.57481594606304576 ) ) ;
#15457=VECTOR ( 'NONE', #23445, 1000.000000000000000 ) ;
#15461=CARTESIAN_POINT ( 'NONE',  ( 126.8853022544570450, 53.90847045361285694, 14.99999999999996447 ) ) ;
#15463=DIRECTION ( 'NONE',  ( 0.000000000000000000, 0.000000000000000000, 1.000000000000000000 ) ) ;
#15464=CARTESIAN_POINT ( 'NONE',  ( 98.15313185440925281, 82.50000000136560629, -4.458734125000016313 ) ) ;
#15465=CARTESIAN_POINT ( 'NONE',  ( 74.29505027212704249, 34.10429687608393579, -9.295050272127046043 ) ) ;
#15467=CARTESIAN_POINT ( 'NONE',  ( 5.444914386472302859, 38.42031250108393436, 13.14518615778179189 ) ) ;
#15471=CARTESIAN_POINT ( 'NONE',  ( 116.4251840539369454, 38.56914062500000284, -5.622872871577873077 ) ) ;
#15473=CARTESIAN_POINT ( 'NONE',  ( 99.99999999999995737, 83.75000000000000000, -5.000000000000018652 ) ) ;
#15477=CARTESIAN_POINT ( 'NONE',  ( 120.7049497278729575, 38.07304687608393579, -9.295050272127046043 ) ) ;
#15478=CARTESIAN_POINT ( 'NONE',  ( 65.00000000000000000, 34.94765625216787441, 13.57481594606304576 ) ) ;
#15480=ORIENTED_EDGE ( 'NONE', *, *, #25386, .T. ) ;
#15482=CARTESIAN_POINT ( 'NONE',  ( 9.598844408820459861, 33.45937500216787441, 9.598844408820456309 ) ) ;
#15485=CARTESIAN_POINT ( 'NONE',  ( 189.5550856135277229, 34.05468750108393294, -13.14518615778179900 ) ) ;
#15489=DIRECTION ( 'NONE',  ( -0.000000000000000000, 1.000000000000000000, -0.000000000000000000 ) ) ;
#15490=VERTEX_POINT ( 'NONE', #24696 ) ;
#15494=CARTESIAN_POINT ( 'NONE',  ( 204.5988444088204403, 39.21406250216787015, -9.598844408820458085 ) ) ;
#15499=CARTESIAN_POINT ( 'NONE',  ( 200.6228728715778686, 35.19570312499999432, -13.57481594606304753 ) ) ;
#15501=DIRECTION ( 'NONE',  ( 0.000000000000000000, -1.000000000000000000, -1.040834085586084848E-15 ) ) ;
#15503=CARTESIAN_POINT ( 'NONE',  ( 51.85481384221820633, 34.99726562608393721, 0.000000000000000000 ) ) ;
#15504=ADVANCED_FACE ( 'NONE', ( #1325 ), #18970, .F. ) ;
#15507=ORIENTED_EDGE ( 'NONE', *, *, #14517, .F. ) ;
#15509=CARTESIAN_POINT ( 'NONE',  ( -8.312177448680279460E-16, 35.24531249999999716, -13.57481594606304576 ) ) ;
#15510=CARTESIAN_POINT ( 'NONE',  ( 124.5550856135277087, 36.13828125108393863, 13.14518615778179722 ) ) ;
#15512=VERTEX_POINT ( 'NONE', #16698 ) ;
#15513=CARTESIAN_POINT ( 'NONE',  ( 104.9999999999999716, 83.50000000000000000, -1.449011120738813565E-14 ) ) ;
#15515=CARTESIAN_POINT ( 'NONE',  ( 94.99999999999995737, 84.06250000273119838, -2.071067811865491048 ) ) ;
#15519=CARTESIAN_POINT ( 'NONE',  ( 51.42518405393695957, 40.15664062500000142, -5.622872871577873077 ) ) ;
#15521=CARTESIAN_POINT ( 'NONE',  ( 139.5988444088204687, 39.01562500216787299, 9.598844408820456309 ) ) ;
#15523=ORIENTED_EDGE ( 'NONE', *, *, #27672, .F. ) ;
#15527=CARTESIAN_POINT ( 'NONE',  ( 208.5748159460630688, 33.55859375216787299, -1.662435489736055892E-15 ) ) ;
#15529=CARTESIAN_POINT ( 'NONE',  ( 99.99999999999995737, 80.00000000000000000, -1.387778780781445676E-14 ) ) ;
#15530=ORIENTED_EDGE ( 'NONE', *, *, #5841, .T. ) ;
#15531=CARTESIAN_POINT ( 'NONE',  ( -5.444914386472299306, 34.55078125108393294, 13.14518615778179722 ) ) ;
#15532=CARTESIAN_POINT ( 'NONE',  ( 120.7049497278729575, 34.89804687608393152, -9.295050272127046043 ) ) ;
#15533=CARTESIAN_POINT ( 'NONE',  ( 51.42518405393695957, 33.80664062500000000, -5.622872871577873077 ) ) ;
#15534=DIRECTION ( 'NONE',  ( 1.000000000000000000, 0.000000000000000000, -7.228014483236696740E-18 ) ) ;
#15536=DIRECTION ( 'NONE',  ( 0.000000000000000000, -1.000000000000000000, 0.000000000000000000 ) ) ;
#15542=CARTESIAN_POINT ( 'NONE',  ( 13.14518615778179900, 36.43593750108392726, -5.444914386472297529 ) ) ;
#15544=ORIENTED_EDGE ( 'NONE', *, *, #19113, .T. ) ;
#15547=CARTESIAN_POINT ( 'NONE',  ( 124.3771271284221314, 36.98164062716787015, -13.57481594606304753 ) ) ;
#15549=CARTESIAN_POINT ( 'NONE',  ( 208.1451861577817795, 36.23750000108393010, -5.444914386472297529 ) ) ;
#15550=ORIENTED_EDGE ( 'NONE', *, *, #10490, .F. ) ;
#15552=CARTESIAN_POINT ( 'NONE',  ( 202.6239419619254818, 55.00000000000001421, -15.00000000000000711 ) ) ;
#15554=ORIENTED_EDGE ( 'NONE', *, *, #4251, .T. ) ;
#15558=CARTESIAN_POINT ( 'NONE',  ( 124.3771271284221314, 31.42539062716787157, -13.57481594606304753 ) ) ;
#15559=CARTESIAN_POINT ( 'NONE',  ( -13.14518615778179544, 39.95820312608393010, 0.000000000000000000 ) ) ;
#15560=EDGE_CURVE ( 'NONE', #17002, #10602, #5707, .T. ) ;
#15562=CARTESIAN_POINT ( 'NONE',  ( 70.44491438647230552, 37.03125000108393294, 13.14518615778179189 ) ) ;
#15563=CARTESIAN_POINT ( 'NONE',  ( 60.49511291368164478, 51.44650206077175625, -15.00000000000199130 ) ) ;
#15564=VERTEX_POINT ( 'NONE', #5601 ) ;
#15566=CARTESIAN_POINT ( 'NONE',  ( 200.6228728715778686, 39.95820312499999716, -13.57481594606304753 ) ) ;
#15567=CARTESIAN_POINT ( 'NONE',  ( -15.00000000000000000, 75.00000000000000000, 10.00000000000000000 ) ) ;
#15568=ORIENTED_EDGE ( 'NONE', *, *, #1814, .F. ) ;
#15569=VERTEX_POINT ( 'NONE', #14408 ) ;
#15572=EDGE_CURVE ( 'NONE', #8963, #26902, #3534, .T. ) ;
#15574=CARTESIAN_POINT ( 'NONE',  ( 200.4449143864723055, 37.92421875108393436, -13.14518615778179722 ) ) ;
#15578=CARTESIAN_POINT ( 'NONE',  ( 181.8548138422182205, 36.73359375108393010, -5.444914386472297529 ) ) ;
#15580=EDGE_CURVE ( 'NONE', #19007, #6540, #9040, .T. ) ;
#15581=EDGE_LOOP ( 'NONE', ( #17495, #5910, #21867, #16827 ) ) ;
#15585=CARTESIAN_POINT ( 'NONE',  ( 116.8548138422182063, 33.65781250108393152, 5.444914386472304635 ) ) ;
#15586=CARTESIAN_POINT ( 'NONE',  ( 59.55508561352770158, 33.55859375108393294, 13.14518615778179722 ) ) ;
#15587=AXIS2_PLACEMENT_3D ( 'NONE', #18463, #1228, #16733 ) ;
#15588=EDGE_CURVE ( 'NONE', #439, #1089, #16275, .T. ) ;
#15589=CARTESIAN_POINT ( 'NONE',  ( 195.0000000000000000, 37.37851562608393863, -13.14518615778179544 ) ) ;
#15590=ORIENTED_EDGE ( 'NONE', *, *, #19754, .F. ) ;
#15592=CARTESIAN_POINT ( 'NONE',  ( -5.444914386472297529, 31.67343750108393863, -13.14518615778179900 ) ) ;
#15594=DIRECTION ( 'NONE',  ( 0.000000000000000000, 0.000000000000000000, 1.000000000000000000 ) ) ;
#15598=CARTESIAN_POINT ( 'NONE',  ( 181.8548138422181921, 40.00781250108393294, 5.444914386472304635 ) ) ;
#15600=ORIENTED_EDGE ( 'NONE', *, *, #1090, .T. ) ;
#15606=CARTESIAN_POINT ( 'NONE',  ( 120.8198241863519797, 50.00000000000000000, 14.99999999999996447 ) ) ;
#15608=ADVANCED_FACE ( 'NONE', ( #25250 ), #10417, .T. ) ;
#15611=CARTESIAN_POINT ( 'NONE',  ( 104.4587341249999781, 81.25000000136560629, -1.846868145590750299 ) ) ;
#15612=CARTESIAN_POINT ( 'NONE',  ( 55.70494972787295751, 36.08867187608393579, 9.295050272127047819 ) ) ;
#15614=CARTESIAN_POINT ( 'NONE',  ( -9.295050272127046043, 38.86679687608393863, -9.295050272127046043 ) ) ;
#15615=EDGE_CURVE ( 'NONE', #8262, #25975, #402, .T. ) ;
#15616=CYLINDRICAL_SURFACE ( 'NONE', #10717, 5.000000000000000000 ) ;
#15619=CARTESIAN_POINT ( 'NONE',  ( 120.4011555911795455, 37.13046874999999147, 9.598844408820459861 ) ) ;
#15621=EDGE_CURVE ( 'NONE', #17097, #12117, #14258, .T. ) ;
#15622=VERTEX_POINT ( 'NONE', #20637 ) ;
#15628=CARTESIAN_POINT ( 'NONE',  ( 124.5550856135277087, 34.35234375108392868, 13.14518615778179722 ) ) ;
#15629=CARTESIAN_POINT ( 'NONE',  ( 78.57481594606304043, 34.40195312716787157, -5.622872871577873077 ) ) ;
#15631=CARTESIAN_POINT ( 'NONE',  ( 104.9999999999999716, 83.56250000000002842, -2.071067811865491937 ) ) ;
#15632=CARTESIAN_POINT ( 'NONE',  ( 5.622872871577871301, 32.91367187716787157, -13.57481594606304753 ) ) ;
#15634=AXIS2_PLACEMENT_3D ( 'NONE', #22491, #13630, #2956 ) ;
#15637=CARTESIAN_POINT ( 'NONE',  ( 200.4449143864723055, 34.45156250108393436, 13.14518615778179189 ) ) ;
#15639=CARTESIAN_POINT ( 'NONE',  ( 203.2014461876500775, 50.69246985422139318, 14.99999999999785416 ) ) ;
#15641=CYLINDRICAL_SURFACE ( 'NONE', #10955, 13.57481594606304398 ) ;
#15642=CARTESIAN_POINT ( 'NONE',  ( 214.9999999999999716, 55.00000000000000000, 9.999999999999946709 ) ) ;
#15648=CARTESIAN_POINT ( 'NONE',  ( 195.0000000000000000, 34.45156249999999432, -13.57481594606304576 ) ) ;
#15651=CARTESIAN_POINT ( 'NONE',  ( 55.70494972787295751, 34.89804687608393152, -9.295050272127046043 ) ) ;
#15655=CARTESIAN_POINT ( 'NONE',  ( 2.493653234604083739E-15, 37.22968749999999716, 13.57481594606304576 ) ) ;
#15656=CARTESIAN_POINT ( 'NONE',  ( 116.8548138422182063, 39.11484375108394573, -5.444914386472297529 ) ) ;
#15658=ORIENTED_EDGE ( 'NONE', *, *, #24079, .T. ) ;
#15659=LINE ( 'NONE', #18084, #26390 ) ;
#15661=CARTESIAN_POINT ( 'NONE',  ( 94.99999999999995737, 81.12500000273119838, -1.387778780781445676E-14 ) ) ;
#15664=AXIS2_PLACEMENT_3D ( 'NONE', #6269, #25522, #5867 ) ;
#15666=CARTESIAN_POINT ( 'NONE',  ( 65.00000000000000000, 39.61093749999999147, 13.57481594606304576 ) ) ;
#15667=EDGE_LOOP ( 'NONE', ( #6855, #9939, #18777, #21211 ) ) ;
#15668=DIRECTION ( 'NONE',  ( -1.000000000000000000, 0.000000000000000000, 0.000000000000000000 ) ) ;
#15673=CARTESIAN_POINT ( 'NONE',  ( 185.4011555911795313, 34.65000000216787868, -9.598844408820458085 ) ) ;
#15676=CARTESIAN_POINT ( 'NONE',  ( 130.0000000000000000, 37.37851562608393863, -13.14518615778179544 ) ) ;
#15678=CARTESIAN_POINT ( 'NONE',  ( 9.295050272127047819, 36.28710937608393294, 9.295050272127046043 ) ) ;
#15679=CARTESIAN_POINT ( 'NONE',  ( 124.5550856135277087, 31.97109375108393436, 13.14518615778179722 ) ) ;
#15680=CARTESIAN_POINT ( 'NONE',  ( 55.40115559117954547, 33.95546874999999432, 9.598844408820459861 ) ) ;
#15683=PLANE ( 'NONE',  #26733 ) ;
#15686=PLANE ( 'NONE',  #26367 ) ;
#15687=CARTESIAN_POINT ( 'NONE',  ( 65.00000000000000000, 37.22968749999999716, 13.57481594606304576 ) ) ;
#15689=CARTESIAN_POINT ( 'NONE',  ( 13.14518615778179900, 36.33671875108394289, 5.444914386472293977 ) ) ;
#15692=DIRECTION ( 'NONE',  ( 0.000000000000000000, 0.000000000000000000, -1.000000000000000000 ) ) ;
#15694=DIRECTION ( 'NONE',  ( -1.000000000000000000, -1.203706215242021094E-31, 3.469446951953613696E-16 ) ) ;
#15695=CARTESIAN_POINT ( 'NONE',  ( 208.1451861577817795, 34.65000000108393152, -5.444914386472297529 ) ) ;
#15696=ORIENTED_EDGE ( 'NONE', *, *, #2053, .T. ) ;
#15697=CARTESIAN_POINT ( 'NONE',  ( 198.1165920804657503, 53.90895096933309105, -15.00000000000000178 ) ) ;
#15705=CARTESIAN_POINT ( 'NONE',  ( 116.4251840539369596, 32.41757812716787157, 5.622872871577880183 ) ) ;
#15708=CARTESIAN_POINT ( 'NONE',  ( 51.85481384221819923, 37.52734375108393294, -5.444914386472297529 ) ) ;
#15709=CARTESIAN_POINT ( 'NONE',  ( 71.16106217484892227, 51.27996893916711940, -15.00000000000068390 ) ) ;
#15711=CARTESIAN_POINT ( 'NONE',  ( 208.1451861577817795, 32.36796875108393579, 5.444914386472293977 ) ) ;
#15712=CARTESIAN_POINT ( 'NONE',  ( 66.13716782454086740, 35.99999999999998579, 13.09590655363602707 ) ) ;
#15716=CARTESIAN_POINT ( 'NONE',  ( 78.14518615778179367, 36.18789062608393436, -1.609821015232357215E-15 ) ) ;
#15719=VERTEX_POINT ( 'NONE', #9790 ) ;
#15723=CARTESIAN_POINT ( 'NONE',  ( 181.8548138422182205, 37.57695312608393579, 0.000000000000000000 ) ) ;
#15730=CARTESIAN_POINT ( 'NONE',  ( 116.8548138422182063, 34.45156250108394147, 5.444914386472304635 ) ) ;
#15731=CARTESIAN_POINT ( 'NONE',  ( 65.00000000000000000, 40.55351562608393579, -13.14518615778179544 ) ) ;
#15732=CARTESIAN_POINT ( 'NONE',  ( 181.8548138422182205, 32.81445312608393294, 0.000000000000000000 ) ) ;
#15733=VERTEX_POINT ( 'NONE', #18497 ) ;
#15735=CARTESIAN_POINT ( 'NONE',  ( 5.444914386472297529, 33.16171875108393152, -13.14518615778179900 ) ) ;
#15736=DIRECTION ( 'NONE',  ( -0.8660254037844407060, 0.4999999999999963363, 0.000000000000000000 ) ) ;
#15738=CARTESIAN_POINT ( 'NONE',  ( 2.129810658427479630, 36.02027164734404607, -13.57481594606306352 ) ) ;
#15739=CARTESIAN_POINT ( 'NONE',  ( 195.0000000000000000, 40.40468749999999432, 13.57481594606304576 ) ) ;
#15740=ADVANCED_FACE ( 'NONE', ( #27204 ), #16263, .T. ) ;
#15742=CARTESIAN_POINT ( 'NONE',  ( 73.25961152888550032, 50.00000000056312643, 10.79618466886052630 ) ) ;
#15743=EDGE_LOOP ( 'NONE', ( #10670, #15948, #10043, #8549 ) ) ;
#15745=VECTOR ( 'NONE', #1930, 1000.000000000000000 ) ;
#15746=EDGE_LOOP ( 'NONE', ( #8316, #24570, #16040, #16024 ) ) ;
#15749=CARTESIAN_POINT ( 'NONE',  ( 137.0894172723430415, 49.99999999943648987, 11.59823041028222157 ) ) ;
#15753=CARTESIAN_POINT ( 'NONE',  ( 214.9999999999999716, 55.00000000000000000, -15.00000000000000000 ) ) ;
#15754=CARTESIAN_POINT ( 'NONE',  ( 59.55508561352770158, 35.04687500108393294, -13.14518615778179900 ) ) ;
#15756=CARTESIAN_POINT ( 'NONE',  ( 13.14518615778179722, 37.03125000108393294, -5.444914386472297529 ) ) ;
#15758=CARTESIAN_POINT ( 'NONE',  ( -1.602533130612661116, 53.60343507248209960, 15.00000000000000000 ) ) ;
#15760=CARTESIAN_POINT ( 'NONE',  ( 120.4011555911795455, 38.71796874999999716, 9.598844408820459861 ) ) ;
#15761=ORIENTED_EDGE ( 'NONE', *, *, #2230, .T. ) ;
#15762=CARTESIAN_POINT ( 'NONE',  ( 65.00000000000000000, -7.395377635281828788, 13.57481594606303688 ) ) ;
#15766=CARTESIAN_POINT ( 'NONE',  ( 130.0000000000000000, 32.81445312608393294, 13.14518615778179544 ) ) ;
#15767=CARTESIAN_POINT ( 'NONE',  ( 51.42518405393695957, 33.90585937716787868, -5.622872871577873077 ) ) ;
#15770=CARTESIAN_POINT ( 'NONE',  ( -13.57481594606304576, 31.57421875216786944, 0.000000000000000000 ) ) ;
#15773=DIRECTION ( 'NONE',  ( -1.000000000000000000, 0.000000000000000000, 7.228014483236696740E-18 ) ) ;
#15775=CARTESIAN_POINT ( 'NONE',  ( 189.5550856135277229, 34.35234375108392868, 13.14518615778179722 ) ) ;
#15778=EDGE_CURVE ( 'NONE', #12289, #12988, #28083, .T. ) ;
#15781=CARTESIAN_POINT ( 'NONE',  ( 120.4011555911795455, 36.43593750216787441, 9.598844408820459861 ) ) ;
#15782=CYLINDRICAL_SURFACE ( 'NONE', #22426, 5.000000000000004441 ) ;
#15792=CARTESIAN_POINT ( 'NONE',  ( 95.54126587499996504, 84.43750000136560629, -1.387778780781445676E-14 ) ) ;
#15793=CARTESIAN_POINT ( 'NONE',  ( 78.14518615778179367, 34.60039062608392868, -1.609821015232357215E-15 ) ) ;
#15797=CARTESIAN_POINT ( 'NONE',  ( 13.57481594606304753, 33.50898437499999716, -5.622872871577873077 ) ) ;
#15798=CARTESIAN_POINT ( 'NONE',  ( 120.7049497278729575, 38.46992187608393721, 9.295050272127047819 ) ) ;
#15802=CARTESIAN_POINT ( 'NONE',  ( 104.9999999999999716, 81.62500000273119838, -1.449011120738813565E-14 ) ) ;
#15804=CARTESIAN_POINT ( 'NONE',  ( 68.62861429328485485, 35.99999999999999289, -13.08307257738123575 ) ) ;
#15806=CARTESIAN_POINT ( 'NONE',  ( 70.62287287157788285, 40.45429687500001137, 13.57481594606304576 ) ) ;
#15808=EDGE_LOOP ( 'NONE', ( #19167, #18839, #24940, #22596, #13854, #26372 ) ) ;
#15809=AXIS2_PLACEMENT_3D ( 'NONE', #27404, #22848, #10260 ) ;
#15814=CARTESIAN_POINT ( 'NONE',  ( 181.4251840539369596, 35.54296875216788010, 0.000000000000000000 ) ) ;
#15816=CARTESIAN_POINT ( 'NONE',  ( 207.0772764098356049, 36.00000000000000711, -6.197985357349214297 ) ) ;
#15817=CARTESIAN_POINT ( 'NONE',  ( 208.5748159460630688, 38.32109375216786873, -1.662435489736055892E-15 ) ) ;
#15818=CARTESIAN_POINT ( 'NONE',  ( 13.14518615778179544, 34.00507812608393721, -1.609821015232357215E-15 ) ) ;
#15819=CARTESIAN_POINT ( 'NONE',  ( 120.7049497278729575, 31.72304687608393081, -9.295050272127046043 ) ) ;
#15821=CARTESIAN_POINT ( 'NONE',  ( 214.9999999999999716, 75.00000000000000000, -15.00000000000000000 ) ) ;
#15822=CARTESIAN_POINT ( 'NONE',  ( 117.9434479702998431, 36.00000000000000000, 5.307619621752288630 ) ) ;
#15824=CARTESIAN_POINT ( 'NONE',  ( 0.000000000000000000, 50.00000000000000000, 0.000000000000000000 ) ) ;
#15830=CARTESIAN_POINT ( 'NONE',  ( 5.444914386472302859, 35.44375000108393436, 13.14518615778179189 ) ) ;
#15834=( BOUNDED_CURVE ( )  B_SPLINE_CURVE ( 2, ( #23033, #3505, #20479, #27184, #12166, #959, #7635, #16329, #5226 ),
 .UNSPECIFIED., .F., .F. ) 
 B_SPLINE_CURVE_WITH_KNOTS ( ( 3, 2, 2, 2, 3 ),
 ( 0.02083333333333358892, 0.03125000000000020123, 0.04166666666666681007, 0.05208333333333342585, 0.06250000000000004163 ),
 .UNSPECIFIED. ) 
 CURVE ( )  GEOMETRIC_REPRESENTATION_ITEM ( )  RATIONAL_B_SPLINE_CURVE ( ( 0.9999999999999981126, 0.9238795325112886259, 1.000000000000000000, 0.9238795325112867385, 1.000000000000000000, 0.9238795325112867385, 1.000000000000000000, 0.9238795325112864054, 1.000000000000000222 ) ) 
 REPRESENTATION_ITEM ( '' )  );
#15835=CARTESIAN_POINT ( 'NONE',  ( 185.7049497278729575, 34.30273437608393294, 9.295050272127047819 ) ) ;
#15837=CARTESIAN_POINT ( 'NONE',  ( 217.9999999999999716, 78.00000000000000000, 12.99999999999994316 ) ) ;
#15842=CARTESIAN_POINT ( 'NONE',  ( 96.46446609406721961, 79.25000000273118417, 3.535533905932727539 ) ) ;
#15843=CIRCLE ( 'NONE', #18593, 13.57481594606304398 ) ;
#15844=CARTESIAN_POINT ( 'NONE',  ( 116.8548138422182063, 36.53515625108392584, -5.444914386472297529 ) ) ;
#15846=CARTESIAN_POINT ( 'NONE',  ( 9.295050272127047819, 35.29492187608393294, 9.295050272127046043 ) ) ;
#15849=CARTESIAN_POINT ( 'NONE',  ( 74.29505027212704249, 37.27929687608394005, -9.295050272127046043 ) ) ;
#15850=CARTESIAN_POINT ( 'NONE',  ( 69.92502678366200541, 49.99999999893144320, -12.67776588292042028 ) ) ;
#15852=CARTESIAN_POINT ( 'NONE',  ( 208.1451861577817795, 33.16171875108393863, 5.444914386472293977 ) ) ;
#15857=CARTESIAN_POINT ( 'NONE',  ( 59.55508561352770158, 38.81718750108393579, -13.14518615778179722 ) ) ;
#15861=EDGE_CURVE ( 'NONE', #291, #10253, #27378, .T. ) ;
#15863=CARTESIAN_POINT ( 'NONE',  ( 200.4449143864723055, 38.61875000108392442, 13.14518615778179189 ) ) ;
#15865=ORIENTED_EDGE ( 'NONE', *, *, #4617, .F. ) ;
#15869=CARTESIAN_POINT ( 'NONE',  ( 143.1451861577818079, 33.16171875108393863, 5.444914386472293977 ) ) ;
#15870=CARTESIAN_POINT ( 'NONE',  ( 181.4251840539369596, 37.08085937716787583, -5.622872871577872189 ) ) ;
#15871=CARTESIAN_POINT ( 'NONE',  ( 189.5550856135277229, 32.96328125108393436, 13.14518615778179722 ) ) ;
#15874=CARTESIAN_POINT ( 'NONE',  ( 4.571591632531690763, 51.44262710532315452, -14.99999999999999112 ) ) ;
#15876=CARTESIAN_POINT ( 'NONE',  ( 143.5748159460630404, 37.57695312716787583, -5.622872871577873077 ) ) ;
#15880=CARTESIAN_POINT ( 'NONE',  ( 189.5550856135277229, 40.60312500108393863, -13.14518615778179900 ) ) ;
#15883=ORIENTED_EDGE ( 'NONE', *, *, #2716, .T. ) ;
#15884=CARTESIAN_POINT ( 'NONE',  ( -0.9955612250524552564, 35.99999999999999289, -13.45766439703027118 ) ) ;
#15886=CARTESIAN_POINT ( 'NONE',  ( 135.6228728715779255, 38.17226562716787441, 13.57481594606301023 ) ) ;
#15889=DIRECTION ( 'NONE',  ( 1.000000000000000000, 0.000000000000000000, -2.385244779468110248E-16 ) ) ;
#15892=CARTESIAN_POINT ( 'NONE',  ( -9.295050272127044266, 39.06523437608392868, 9.295050272127047819 ) ) ;
#15893=CARTESIAN_POINT ( 'NONE',  ( 0.3969994146497132781, 51.45716825712461429, 15.00000000000033573 ) ) ;
#15894=CARTESIAN_POINT ( 'NONE',  ( 0.000000000000000000, 36.00000000000000000, 11.57481594606304398 ) ) ;
#15895=CARTESIAN_POINT ( 'NONE',  ( 120.4011555911795455, 35.34453124999998863, -9.598844408820458085 ) ) ;
#15896=ORIENTED_EDGE ( 'NONE', *, *, #8116, .T. ) ;
#15897=EDGE_CURVE ( 'NONE', #8880, #9852, #19168, .T. ) ;
#15901=CARTESIAN_POINT ( 'NONE',  ( 139.2950502721270425, 33.70742187608393436, 9.295050272127046043 ) ) ;
#15902=CARTESIAN_POINT ( 'NONE',  ( 70.44491438647230552, 38.71796875108393721, -13.14518615778179900 ) ) ;
#15903=CARTESIAN_POINT ( 'NONE',  ( -8.312177448680279460E-16, 37.72578125216787726, -13.57481594606304576 ) ) ;
#15904=CARTESIAN_POINT ( 'NONE',  ( -9.295050272127044266, 38.27148437608393294, 9.295050272127047819 ) ) ;
#15911=AXIS2_PLACEMENT_3D ( 'NONE', #21033, #12443, #10170 ) ;
#15914=EDGE_LOOP ( 'NONE', ( #13861, #15301, #12249, #1901 ) ) ;
#15915=EDGE_CURVE ( 'NONE', #19327, #24259, #19518, .T. ) ;
#15916=DIRECTION ( 'NONE',  ( 0.000000000000000000, 0.000000000000000000, -1.000000000000000000 ) ) ;
#15917=LINE ( 'NONE', #22644, #20146 ) ;
#15922=CARTESIAN_POINT ( 'NONE',  ( 200.6228728715778686, 32.51679687499999716, 13.57481594606304576 ) ) ;
#15924=CARTESIAN_POINT ( 'NONE',  ( 9.598844408820459861, 36.53515624999999289, 9.598844408820456309 ) ) ;
#15925=CARTESIAN_POINT ( 'NONE',  ( 98.15313185440925281, 82.62500000136560629, 4.458734124999987891 ) ) ;
#15926=CARTESIAN_POINT ( 'NONE',  ( 59.55508561352770158, 31.67343750108393863, -13.14518615778179900 ) ) ;
#15929=ORIENTED_EDGE ( 'NONE', *, *, #10025, .F. ) ;
#15932=CARTESIAN_POINT ( 'NONE',  ( 5.622872871577871301, 34.40195312499999858, -13.57481594606304753 ) ) ;
#15933=CARTESIAN_POINT ( 'NONE',  ( 130.0000000000000000, 38.96601562608393721, -13.14518615778179544 ) ) ;
#15934=EDGE_LOOP ( 'NONE', ( #9986, #7005, #25825, #17861 ) ) ;
#15935=CARTESIAN_POINT ( 'NONE',  ( 116.6399989480775901, 40.42949218912590936, 0.000000000000000000 ) ) ;
#15938=CARTESIAN_POINT ( 'NONE',  ( 102.0710678118654329, 79.81250000273119838, -5.000000000000018652 ) ) ;
#15940=CARTESIAN_POINT ( 'NONE',  ( 74.59884440882045453, 40.00781250216787299, -9.598844408820458085 ) ) ;
#15943=CARTESIAN_POINT ( 'NONE',  ( 55.40115559117954547, 40.10703124999999147, -9.598844408820458085 ) ) ;
#15944=ORIENTED_EDGE ( 'NONE', *, *, #27136, .T. ) ;
#15945=CARTESIAN_POINT ( 'NONE',  ( 186.3308878946625100, 36.00000000000000000, -10.16963847934286314 ) ) ;
#15948=ORIENTED_EDGE ( 'NONE', *, *, #973, .T. ) ;
#15950=CARTESIAN_POINT ( 'NONE',  ( 189.3771271284221314, 34.60039062716786873, -13.57481594606304753 ) ) ;
#15951=( BOUNDED_CURVE ( )  B_SPLINE_CURVE ( 2, ( #26393, #5015, #18112 ),
 .UNSPECIFIED., .F., .T. ) 
 B_SPLINE_CURVE_WITH_KNOTS ( ( 3, 3 ),
 ( 0.5208333333333332593, 0.5249747582430960291 ),
 .UNSPECIFIED. ) 
 CURVE ( )  GEOMETRIC_REPRESENTATION_ITEM ( )  RATIONAL_B_SPLINE_CURVE ( ( 1.000000000000000888, 0.9697362687807487003, 0.9635368518655809122 ) ) 
 REPRESENTATION_ITEM ( '' )  );
#15953=LINE ( 'NONE', #11104, #3490 ) ;
#15955=CARTESIAN_POINT ( 'NONE',  ( 9.295050272127047819, 35.49335937608393721, 9.295050272127046043 ) ) ;
#15960=CARTESIAN_POINT ( 'NONE',  ( 195.0000000000000000, 40.10703125216787157, -13.57481594606304576 ) ) ;
#15962=CARTESIAN_POINT ( 'NONE',  ( -5.622872871577839327, 38.07304687716787583, 13.57481594606308128 ) ) ;
#15963=AXIS2_PLACEMENT_3D ( 'NONE', #11348, #14061, #18061 ) ;
#15966=DIRECTION ( 'NONE',  ( -0.000000000000000000, 1.000000000000000000, -0.000000000000000000 ) ) ;
#15969=CARTESIAN_POINT ( 'NONE',  ( -9.295050272127046043, 34.30273437608393294, -9.295050272127046043 ) ) ;
#15973=ADVANCED_FACE ( 'NONE', ( #10787 ), #21228, .T. ) ;
#15975=CARTESIAN_POINT ( 'NONE',  ( 181.8548138422182205, 36.58476562608393579, 0.000000000000000000 ) ) ;
#15977=CARTESIAN_POINT ( 'NONE',  ( 188.9209199794811411, 54.65154858643464308, -15.00000000000000000 ) ) ;
#15979=ORIENTED_EDGE ( 'NONE', *, *, #17301, .F. ) ;
#15983=CARTESIAN_POINT ( 'NONE',  ( 13.57481594606304753, 39.06523437499999574, -5.622872871577873966 ) ) ;
#15984=CARTESIAN_POINT ( 'NONE',  ( 135.4449143864723055, 37.62656250108393863, 13.14518615778179189 ) ) ;
#15985=CARTESIAN_POINT ( 'NONE',  ( -13.14518615778179722, 39.11484375108393863, -5.444914386472297529 ) ) ;
#15986=CARTESIAN_POINT ( 'NONE',  ( -13.14518615778179900, 34.15390625108393863, -5.444914386472297529 ) ) ;
#15988=CARTESIAN_POINT ( 'NONE',  ( 73.26859732838660477, 50.00000000054332361, -10.78867689284328790 ) ) ;
#15990=CARTESIAN_POINT ( 'NONE',  ( 66.68551164908284079, 35.99999999999997868, 13.05727741351676130 ) ) ;
#15994=CARTESIAN_POINT ( 'NONE',  ( 65.00000000000000000, 37.97382812608393721, -13.14518615778179544 ) ) ;
#15995=CARTESIAN_POINT ( 'NONE',  ( 2.493653234604083739E-15, 38.81718749999999574, 13.57481594606304576 ) ) ;
#15996=CARTESIAN_POINT ( 'NONE',  ( 181.8548138422182205, 36.58476562608393579, 0.000000000000000000 ) ) ;
#16003=CARTESIAN_POINT ( 'NONE',  ( 185.7049497278729575, 36.88242187608393152, 9.295050272127047819 ) ) ;
#16009=CARTESIAN_POINT ( 'NONE',  ( 143.1451861577818079, 32.36796875108393579, 5.444914386472293977 ) ) ;
#16010=CARTESIAN_POINT ( 'NONE',  ( 185.4011555911795597, 37.22968750216787726, 9.598844408820459861 ) ) ;
#16011=CARTESIAN_POINT ( 'NONE',  ( 208.1451861577817795, 35.54296875108394715, 5.444914386472293977 ) ) ;
#16012=ORIENTED_EDGE ( 'NONE', *, *, #6858, .T. ) ;
#16015=CARTESIAN_POINT ( 'NONE',  ( 120.8198241863519797, 50.00000000000000000, -9.999999999999976907 ) ) ;
#16016=CARTESIAN_POINT ( 'NONE',  ( 130.0000000000000000, 36.53515625216787299, 13.57481594606304576 ) ) ;
#16018=EDGE_CURVE ( 'NONE', #10588, #15564, #23367, .T. ) ;
#16021=CARTESIAN_POINT ( 'NONE',  ( 200.4449143864723055, 40.20625000108394431, 13.14518615778179189 ) ) ;
#16024=ORIENTED_EDGE ( 'NONE', *, *, #23185, .T. ) ;
#16025=CARTESIAN_POINT ( 'NONE',  ( 2.007297010069739596, 35.99999999999998579, -13.40042260803723373 ) ) ;
#16030=CARTESIAN_POINT ( 'NONE',  ( 55.70494972787295751, 33.50898437608393010, -9.295050272127046043 ) ) ;
#16031=CARTESIAN_POINT ( 'NONE',  ( -15.00000000000000355, 55.00000000000000000, -9.999999999999998224 ) ) ;
#16032=CARTESIAN_POINT ( 'NONE',  ( 217.9999999999999716, 80.00000000000000000, 14.99999999999994316 ) ) ;
#16036=CARTESIAN_POINT ( 'NONE',  ( -1.014130826074097769, 51.45790058219388641, 14.99999999999932143 ) ) ;
#16038=CARTESIAN_POINT ( 'NONE',  ( 120.4011555911795455, 33.16171874999999858, 9.598844408820459861 ) ) ;
#16039=VECTOR ( 'NONE', #6118, 1000.000000000000000 ) ;
#16040=ORIENTED_EDGE ( 'NONE', *, *, #23640, .T. ) ;
#16041=CARTESIAN_POINT ( 'NONE',  ( -20.00000000000000000, 80.00000000000000000, 15.00000000000000178 ) ) ;
#16045=CARTESIAN_POINT ( 'NONE',  ( 124.5550856135277087, 34.05468750108393294, -13.14518615778179900 ) ) ;
#16048=CARTESIAN_POINT ( 'NONE',  ( 78.57481594606304043, 31.92148437716787512, 5.622872871577869525 ) ) ;
#16049=CYLINDRICAL_SURFACE ( 'NONE', #10220, 13.57481594606304398 ) ;
#16050=CARTESIAN_POINT ( 'NONE',  ( 13.14518615778179900, 39.31328125108392868, 5.444914386472293977 ) ) ;
#16056=CARTESIAN_POINT ( 'NONE',  ( -8.049105076161786076E-16, 40.35507812608393152, -13.14518615778179544 ) ) ;
#16061=DIRECTION ( 'NONE',  ( 0.000000000000000000, 0.000000000000000000, -1.000000000000000000 ) ) ;
#16068=CARTESIAN_POINT ( 'NONE',  ( 195.0000000000000000, 32.07031249999999289, -13.57481594606304576 ) ) ;
#16071=CARTESIAN_POINT ( 'NONE',  ( 104.4587341249999781, 84.00000000136560629, -1.846868145590750299 ) ) ;
#16072=CARTESIAN_POINT ( 'NONE',  ( 70.44491438647230552, 32.36796875108393579, -13.14518615778179900 ) ) ;
#16076=CARTESIAN_POINT ( 'NONE',  ( -13.57481594606304576, 34.69960937499999432, 5.622872871577880183 ) ) ;
#16077=CARTESIAN_POINT ( 'NONE',  ( 120.7049497278729575, 36.08867187608393579, 9.295050272127047819 ) ) ;
#16078=VERTEX_POINT ( 'NONE', #19080 ) ;
#16079=CARTESIAN_POINT ( 'NONE',  ( 97.92893218813451028, 81.81250000000001421, -5.000000000000018652 ) ) ;
#16081=CARTESIAN_POINT ( 'NONE',  ( 98.15313185440925281, 82.25000000136559208, -4.458734125000016313 ) ) ;
#16083=CARTESIAN_POINT ( 'NONE',  ( 51.42518405393695957, 39.56132812716787583, 5.622872871577880183 ) ) ;
#16084=VECTOR ( 'NONE', #4360, 1000.000000000000000 ) ;
#16085=EDGE_CURVE ( 'NONE', #8914, #22555, #12646, .T. ) ;
#16087=CARTESIAN_POINT ( 'NONE',  ( 78.14518615778179367, 32.36796875108393579, 5.444914386472293977 ) ) ;
#16088=CARTESIAN_POINT ( 'NONE',  ( -13.57481594606304576, 38.76757812716787299, 5.622872871577880183 ) ) ;
#16089=ORIENTED_EDGE ( 'NONE', *, *, #26904, .T. ) ;
#16094=CARTESIAN_POINT ( 'NONE',  ( 181.8548138422182205, 39.75976562608393294, 0.000000000000000000 ) ) ;
#16098=CARTESIAN_POINT ( 'NONE',  ( 143.1451861577818363, 40.20625000108393010, -5.444914386472297529 ) ) ;
#16099=CARTESIAN_POINT ( 'NONE',  ( 2.414731522848535132E-15, 36.18789062608393436, 13.14518615778179544 ) ) ;
#16101=CARTESIAN_POINT ( 'NONE',  ( 139.2950502721270425, 32.31835937608393294, -9.295050272127046043 ) ) ;
#16104=EDGE_CURVE ( 'NONE', #21810, #2105, #23012, .T. ) ;
#16106=CARTESIAN_POINT ( 'NONE',  ( 78.57481594606305464, 36.68398437716787441, 5.622872871577868636 ) ) ;
#16108=FACE_OUTER_BOUND ( 'NONE', #3860, .T. ) ;
#16112=CARTESIAN_POINT ( 'NONE',  ( 214.9999999999999716, 55.00000000000000000, 14.99999999999994316 ) ) ;
#16114=CARTESIAN_POINT ( 'NONE',  ( -13.14518615778179544, 32.02070312608393010, 0.000000000000000000 ) ) ;
#16115=EDGE_CURVE ( 'NONE', #1696, #747, #5067, .T. ) ;
#16116=VERTEX_POINT ( 'NONE', #11069 ) ;
#16119=CARTESIAN_POINT ( 'NONE',  ( 181.8548138422181921, 36.53515625108392584, -5.444914386472297529 ) ) ;
#16120=( BOUNDED_CURVE ( )  B_SPLINE_CURVE ( 2, ( #23560, #12702, #17127, #12280, #16857, #21426, #14288, #1905, #5620 ),
 .UNSPECIFIED., .F., .T. ) 
 B_SPLINE_CURVE_WITH_KNOTS ( ( 3, 2, 2, 2, 3 ),
 ( 0.06250000000000004163, 0.07291666666666665741, 0.08333333333333325932, 0.09374999999999987510, 0.1041666666666664909 ),
 .UNSPECIFIED. ) 
 CURVE ( )  GEOMETRIC_REPRESENTATION_ITEM ( )  RATIONAL_B_SPLINE_CURVE ( ( 0.9999999999999996669, 0.9238795325112870716, 1.000000000000000000, 0.9238795325112867385, 1.000000000000000000, 0.9238795325112867385, 1.000000000000000000, 0.9238795325112880708, 0.9999999999999986677 ) ) 
 REPRESENTATION_ITEM ( '' )  );
#16121=ORIENTED_EDGE ( 'NONE', *, *, #4456, .T. ) ;
#16122=CARTESIAN_POINT ( 'NONE',  ( 194.1234737346433405, 51.45968077934669793, -15.00000000000000000 ) ) ;
#16128=CARTESIAN_POINT ( 'NONE',  ( 130.0000000000000000, -7.395377635281828788, -1.503427012513233026E-14 ) ) ;
#16129=CYLINDRICAL_SURFACE ( 'NONE', #781, 5.000000000000000888 ) ;
#16130=CARTESIAN_POINT ( 'NONE',  ( 139.2950502721270425, 38.46992187608393010, 9.295050272127046043 ) ) ;
#16131=CARTESIAN_POINT ( 'NONE',  ( 5.444914386472297529, 37.32890625108393579, -13.14518615778179722 ) ) ;
#16132=CARTESIAN_POINT ( 'NONE',  ( -9.295050272127044266, 35.89023437608393152, 9.295050272127047819 ) ) ;
#16134=EDGE_CURVE ( 'NONE', #540, #25247, #8594, .T. ) ;
#16136=CARTESIAN_POINT ( 'NONE',  ( 71.45087934266470597, 50.00000000106856390, -11.97362904075383305 ) ) ;
#16139=EDGE_LOOP ( 'NONE', ( #13897, #4364, #26796 ) ) ;
#16143=CARTESIAN_POINT ( 'NONE',  ( 74.29505027212704249, 36.88242187608393152, 9.295050272127046043 ) ) ;
#16144=DIRECTION ( 'NONE',  ( 0.000000000000000000, 0.000000000000000000, 1.000000000000000000 ) ) ;
#16149=CARTESIAN_POINT ( 'NONE',  ( 185.7049497278729575, 39.26367187608393294, 9.295050272127047819 ) ) ;
#16151=VERTEX_POINT ( 'NONE', #2689 ) ;
#16155=EDGE_LOOP ( 'NONE', ( #17955, #9215, #17409, #11443, #7627 ) ) ;
#16157=CARTESIAN_POINT ( 'NONE',  ( 55.70494972787295751, 40.05742187608393579, 9.295050272127047819 ) ) ;
#16159=CARTESIAN_POINT ( 'NONE',  ( 181.8548138422181921, 35.24531250108393721, 5.444914386472304635 ) ) ;
#16161=LINE ( 'NONE', #22739, #18449 ) ;
#16163=EDGE_CURVE ( 'NONE', #17097, #23414, #6658, .T. ) ;
#16164=CARTESIAN_POINT ( 'NONE',  ( 143.5748159460630404, 38.27148437716787299, 5.622872871577869525 ) ) ;
#16166=CARTESIAN_POINT ( 'NONE',  ( 130.0000000000000000, -7.395377635281828788, -1.503427012513233026E-14 ) ) ;
#16168=CARTESIAN_POINT ( 'NONE',  ( 72.08941727233755614, 49.99999999943687357, 11.59823041028754353 ) ) ;
#16170=VECTOR ( 'NONE', #4834, 1000.000000000000000 ) ;
#16171=ORIENTED_EDGE ( 'NONE', *, *, #19646, .F. ) ;
#16174=CARTESIAN_POINT ( 'NONE',  ( -13.10247082172194943, 36.00000000000000711, -1.608626461598226420 ) ) ;
#16179=CARTESIAN_POINT ( 'NONE',  ( -13.57481594606304576, 40.30546875216787583, 0.000000000000000000 ) ) ;
#16181=CARTESIAN_POINT ( 'NONE',  ( 65.00000000000000000, 38.02343749999999289, 13.57481594606304576 ) ) ;
#16183=AXIS2_PLACEMENT_3D ( 'NONE', #19979, #2598, #18116 ) ;
#16185=CARTESIAN_POINT ( 'NONE',  ( 3.044609456929385338, 53.89089363584395898, 14.99999999999999645 ) ) ;
#16186=DIRECTION ( 'NONE',  ( 1.000000000000000000, 0.000000000000000000, 0.000000000000000000 ) ) ;
#16187=CARTESIAN_POINT ( 'NONE',  ( 143.5748159460630404, 35.09648437499998863, -5.622872871577873077 ) ) ;
#16189=LINE ( 'NONE', #9493, #21310 ) ;
#16193=CARTESIAN_POINT ( 'NONE',  ( 120.7049497278729575, 34.30273437608393294, 9.295050272127047819 ) ) ;
#16194=CARTESIAN_POINT ( 'NONE',  ( 51.85481384221820633, 40.55351562608393579, 0.000000000000000000 ) ) ;
#16197=CARTESIAN_POINT ( 'NONE',  ( 9.295050272127046043, 40.25585937608393294, -9.295050272127046043 ) ) ;
#16200=CARTESIAN_POINT ( 'NONE',  ( 217.9999999999999716, 78.00000000000000000, 0.000000000000000000 ) ) ;
#16202=CARTESIAN_POINT ( 'NONE',  ( 200.4449143864723055, 32.07031250108393294, 13.14518615778179189 ) ) ;
#16203=VECTOR ( 'NONE', #25301, 1000.000000000000000 ) ;
#16207=CARTESIAN_POINT ( 'NONE',  ( 128.1834995827138073, 36.00000000000000000, -13.35830014193465587 ) ) ;
#16208=ORIENTED_EDGE ( 'NONE', *, *, #16454, .F. ) ;
#16210=CARTESIAN_POINT ( 'NONE',  ( 195.0000000000000000, -7.395377635281828788, -11.57481594606306707 ) ) ;
#16216=CARTESIAN_POINT ( 'NONE',  ( 185.4011555911795313, 32.96328124999999432, -9.598844408820458085 ) ) ;
#16218=CARTESIAN_POINT ( 'NONE',  ( 5.622872871577832221, 36.48554687499999716, 13.57481594606309194 ) ) ;
#16219=CARTESIAN_POINT ( 'NONE',  ( 130.0000000000000000, -7.395377635281828788, 13.57481594606302799 ) ) ;
#16220=CARTESIAN_POINT ( 'NONE',  ( 55.70494972787295751, 32.71523437608393436, 9.295050272127047819 ) ) ;
#16224=CARTESIAN_POINT ( 'NONE',  ( -8.312177448680279460E-16, 39.31328125216787583, -13.57481594606304576 ) ) ;
#16225=CARTESIAN_POINT ( 'NONE',  ( -5.622872871577873077, 33.21132812499999432, 13.57481594606304753 ) ) ;
#16227=CARTESIAN_POINT ( 'NONE',  ( 116.8548138422182063, 35.14609375108393152, -5.444914386472297529 ) ) ;
#16230=CARTESIAN_POINT ( 'NONE',  ( 96.46446609406721961, 80.87500000000000000, -3.535533905932755072 ) ) ;
#16231=ADVANCED_FACE ( 'NONE', ( #24059 ), #15641, .T. ) ;
#16233=CARTESIAN_POINT ( 'NONE',  ( 95.54126587499995082, 82.37500000136562051, -1.846868145590750077 ) ) ;
#16236=FACE_OUTER_BOUND ( 'NONE', #25766, .T. ) ;
#16238=CARTESIAN_POINT ( 'NONE',  ( 195.0000000000000000, 31.62382812608393579, -13.14518615778179544 ) ) ;
#16239=CARTESIAN_POINT ( 'NONE',  ( 13.57481594606304753, 39.16445312716788152, -5.622872871577873077 ) ) ;
#16240=ORIENTED_EDGE ( 'NONE', *, *, #21846, .T. ) ;
#16241=CARTESIAN_POINT ( 'NONE',  ( 197.0072970100686405, 35.99999999999999289, -13.40042260803738650 ) ) ;
#16245=CARTESIAN_POINT ( 'NONE',  ( 208.1451861577817795, 40.20625000108393010, -5.444914386472297529 ) ) ;
#16248=CARTESIAN_POINT ( 'NONE',  ( 135.4449143864723339, 40.00781250108393294, 13.14518615778179189 ) ) ;
#16249=CARTESIAN_POINT ( 'NONE',  ( 96.46446615806316061, 80.00000000000000000, -3.535533969928681852 ) ) ;
#16250=CARTESIAN_POINT ( 'NONE',  ( 70.62287287157786864, 32.81445312499999289, -13.57481594606304753 ) ) ;
#16254=CARTESIAN_POINT ( 'NONE',  ( 59.55508561352770158, 40.40468750108393436, -13.14518615778179900 ) ) ;
#16258=CARTESIAN_POINT ( 'NONE',  ( 208.5748159460630688, 39.85898437499999858, -5.622872871577873966 ) ) ;
#16259=DIRECTION ( 'NONE',  ( 0.000000000000000000, 0.000000000000000000, 1.000000000000000000 ) ) ;
#16260=CARTESIAN_POINT ( 'NONE',  ( -9.295050272127044266, 32.91367187608393152, 9.295050272127047819 ) ) ;
#16261=VERTEX_POINT ( 'NONE', #262 ) ;
#16263=( BOUNDED_SURFACE ( )  B_SPLINE_SURFACE ( 1, 2, ( 
 ( #7656, #16348, #24627, #13767, #16056, #23052, #5533, #14197, #22917, #23601, #27609, #23466, #21470, #6349, #1946, #14744, #17030, #1536, #21327, #23327, #10614, #4082, #19321, #28023, #8489, #10188, #25594, #3943, #17176, #1808, #6078, #25880, #5942, #5807, #12603, #10473, #19181, #27883, #25464, #14610, #15023, #3801, #23743, #21606, #27747, #18899, #16762, #4218, #8207, #14477, #12877, #23194, #8345, #2084, #10753, #6216, #19464, #12745, #19035, #7930, #3671, #1671, #16627, #25319, #8067, #16896, #12333, #25733, #21052, #12461, #21186, #10328, #14885, #2229, #5179, #22710, #13703, #26992, #26702, #24024, #15309, #20141, #7297, #26016, #15161, #13842, #3180, #7151, #26156, #22567, #23881, #17456, #22283, #8767, #16132, #4896, #17319, #4359, #11421, #11850, #3034, #621, #11703, #17992, #6624, #9437, #15846, #5323, #13560, #20428, #13015, #2758, #9295, #24556, #24840, #5037, #6487, #21754, #22420, #28161, #912, #2891, #9582, #11561, #20277, #18137, #764, #13982, #26850, #15986, #8628, #24700, #18286, #7438, #10893, #19601, #85, #27407, #18975, #1196, #27135, #3874, #7868, #21121, #27683, #9864, #18704, #12124, #14413, #18571, #23401, #1053, #25537, #8146, #16840, #14271, #24979, #8002, #11991, #16563, #5882, #6017, #14551, #25253, #1469, #14131, #5743, #7729, #23267, #16703, #3740, #12400, #1607, #22852, #9996, #23128, #10265, #3604, #12263, #14680, #27274, #18427, #20988 ),
 ( #16420, #20572, #9725, #20850, #3319, #25117, #7587, #1330, #16280, #5462, #20714, #10125, #5604, #22989, #18838, #3458, #25401, #27545, #2306, #8279, #6285, #24098, #21264, #4017, #21543, #19118, #4158, #15384, #27825, #21408, #10965, #12536, #14817, #17396, #6696, #25953, #19677, #10686, #8415, #27959, #12819, #19538, #10411, #16970, #26094, #1746, #19394, #13090, #23541, #23959, #28099, #8562, #6559, #12952, #4438, #25669, #20, #15239, #6151, #17535, #17105, #2161, #12683, #1887, #10551, #2018, #8703, #10823, #19259, #8845, #26239, #17252, #21830, #25809, #14961, #23681, #6427, #15096, #23817, #163, #4295, #21686, #13811, #17679, #18254, #732, #9129, #7406, #22389, #3001, #15678, #2588, #16099, #24524, #4575, #9405, #22533, #13235, #11106, #7264, #17963, #7120, #24378, #589, #881, #5146, #15955, #26673, #21968, #2445, #11674, #26385, #20396, #2861, #19820, #11529, #6840, #22109, #304, #26818, #18105, #22251, #2728, #19967, #8990, #15531, #24238, #6982, #24670, #9553, #4867, #4721, #26962, #13381, #11249, #17822, #15818, #445, #9267, #5009, #26527, #11391, #13531, #20112, #13674, #20246, #3424, #14516, #1295, #7838, #5288, #7970, #11960, #8110, #13953, #22962, #9965, #22821, #24946, #16670, #3709, #7698, #23232, #24806, #22679, #3569, #20682, #12371, #20817, #25367, #5432, #21089, #3289, #27242, #9695, #14379, #11819, #23095, #18395, #14100, #20542, #18808, #10095 ) ),
 .UNSPECIFIED., .F., .F., .T. ) 
 B_SPLINE_SURFACE_WITH_KNOTS ( ( 2, 2 ),
 ( 3, 2, 2, 2, 2, 2, 2, 2, 2, 2, 2, 2, 2, 2, 2, 2, 2, 2, 2, 2, 2, 2, 2, 2, 2, 2, 2, 2, 2, 2, 2, 2, 2, 2, 2, 2, 2, 2, 2, 2, 2, 2, 2, 2, 2, 2, 2, 2, 2, 2, 2, 2, 2, 2, 2, 2, 2, 2, 2, 2, 2, 2, 2, 2, 2, 2, 2, 2, 2, 2, 2, 2, 2, 2, 2, 2, 2, 2, 2, 2, 2, 2, 2, 2, 2, 2, 2, 2, 2, 2, 2, 3 ),
 ( 0.000000000000000000, 1.000000000000000000 ),
 ( 0.000000000000000000, 0.01041666666666666609, 0.02083333333333333218, 0.03125000000000000000, 0.04166666666666666435, 0.05208333333333333565, 0.06250000000000000000, 0.07291666666666667129, 0.08333333333333332871, 0.09375000000000000000, 0.1041666666666666713, 0.1145833333333333287, 0.1250000000000000000, 0.1354166666666666574, 0.1458333333333333426, 0.1562500000000000000, 0.1666666666666666574, 0.1770833333333333426, 0.1875000000000000000, 0.1979166666666666574, 0.2083333333333333426, 0.2187500000000000000, 0.2291666666666666574, 0.2395833333333333426, 0.2500000000000000000, 0.2604166666666666852, 0.2708333333333333148, 0.2812500000000000000, 0.2916666666666666852, 0.3020833333333333148, 0.3125000000000000000, 0.3229166666666666852, 0.3333333333333333148, 0.3437500000000000000, 0.3541666666666666852, 0.3645833333333333148, 0.3750000000000000000, 0.3854166666666666852, 0.3958333333333333148, 0.4062500000000000000, 0.4166666666666666852, 0.4270833333333333148, 0.4375000000000000000, 0.4479166666666666852, 0.4583333333333333148, 0.4687500000000000000, 0.4791666666666666852, 0.4895833333333333148, 0.5000000000000000000, 0.5104166666666666297, 0.5208333333333333703, 0.5312500000000000000, 0.5416666666666666297, 0.5520833333333333703, 0.5625000000000000000, 0.5729166666666666297, 0.5833333333333333703, 0.5937500000000000000, 0.6041666666666666297, 0.6145833333333333703, 0.6250000000000000000, 0.6354166666666666297, 0.6458333333333333703, 0.6562500000000000000, 0.6666666666666666297, 0.6770833333333333703, 0.6875000000000000000, 0.6979166666666666297, 0.7083333333333333703, 0.7187500000000000000, 0.7291666666666666297, 0.7395833333333333703, 0.7500000000000000000, 0.7604166666666666297, 0.7708333333333333703, 0.7812500000000000000, 0.7916666666666666297, 0.8020833333333333703, 0.8125000000000000000, 0.8229166666666666297, 0.8333333333333333703, 0.8437500000000000000, 0.8541666666666666297, 0.8645833333333333703, 0.8750000000000000000, 0.8854166666666666297, 0.8958333333333333703, 0.9062500000000000000, 0.9166666666666666297, 0.9270833333333333703, 0.9375000000000000000, 0.9448587001587775980 ),
 .UNSPECIFIED. ) 
 GEOMETRIC_REPRESENTATION_ITEM ( )  RATIONAL_B_SPLINE_SURFACE ( (
 ( 1.000000000000000000, 0.9238795325112867385, 1.000000000000000000, 0.9238795325112867385, 1.000000000000000000, 0.9238795325112867385, 1.000000000000000000, 0.9238795325112867385, 1.000000000000000000, 0.9238795325112867385, 1.000000000000000000, 0.9238795325112867385, 1.000000000000000000, 0.9238795325112867385, 1.000000000000000000, 0.9238795325112867385, 1.000000000000000000, 0.9238795325112867385, 1.000000000000000000, 0.9238795325112867385, 1.000000000000000000, 0.9238795325112867385, 1.000000000000000000, 0.9238795325112867385, 1.000000000000000000, 0.9238795325112867385, 1.000000000000000000, 0.9238795325112867385, 1.000000000000000000, 0.9238795325112867385, 1.000000000000000000, 0.9238795325112867385, 1.000000000000000000, 0.9238795325112867385, 1.000000000000000000, 0.9238795325112867385, 1.000000000000000000, 0.9238795325112867385, 1.000000000000000000, 0.9238795325112867385, 1.000000000000000000, 0.9238795325112867385, 1.000000000000000000, 0.9238795325112867385, 1.000000000000000000, 0.9238795325112867385, 1.000000000000000000, 0.9238795325112867385, 1.000000000000000000, 0.9238795325112867385, 1.000000000000000000, 0.9238795325112867385, 1.000000000000000000, 0.9238795325112867385, 1.000000000000000000, 0.9238795325112867385, 1.000000000000000000, 0.9238795325112867385, 1.000000000000000000, 0.9238795325112867385, 1.000000000000000000, 0.9238795325112867385, 1.000000000000000000, 0.9238795325112867385, 1.000000000000000000, 0.9238795325112867385, 1.000000000000000000, 0.9238795325112867385, 1.000000000000000000, 0.9238795325112867385, 1.000000000000000000, 0.9238795325112867385, 1.000000000000000000, 0.9238795325112867385, 1.000000000000000000, 0.9238795325112867385, 1.000000000000000000, 0.9238795325112867385, 1.000000000000000000, 0.9238795325112867385, 1.000000000000000000, 0.9238795325112867385, 1.000000000000000000, 0.9238795325112867385, 1.000000000000000000, 0.9238795325112867385, 1.000000000000000000, 0.9238795325112867385, 1.000000000000000000, 0.9238795325112867385, 1.000000000000000000, 0.9238795325112867385, 1.000000000000000000, 0.9238795325112867385, 1.000000000000000000, 0.9238795325112867385, 1.000000000000000000, 0.9238795325112867385, 1.000000000000000000, 0.9238795325112867385, 1.000000000000000000, 0.9238795325112867385, 1.000000000000000000, 0.9238795325112867385, 1.000000000000000000, 0.9238795325112867385, 1.000000000000000000, 0.9238795325112867385, 1.000000000000000000, 0.9238795325112867385, 1.000000000000000000, 0.9238795325112867385, 1.000000000000000000, 0.9238795325112867385, 1.000000000000000000, 0.9238795325112867385, 1.000000000000000000, 0.9238795325112867385, 1.000000000000000000, 0.9238795325112867385, 1.000000000000000000, 0.9238795325112867385, 1.000000000000000000, 0.9238795325112867385, 1.000000000000000000, 0.9238795325112867385, 1.000000000000000000, 0.9238795325112867385, 1.000000000000000000, 0.9238795325112867385, 1.000000000000000000, 0.9238795325112867385, 1.000000000000000000, 0.9238795325112867385, 1.000000000000000000, 0.9238795325112867385, 1.000000000000000000, 0.9238795325112867385, 1.000000000000000000, 0.9238795325112867385, 1.000000000000000000, 0.9238795325112867385, 1.000000000000000000, 0.9238795325112867385, 1.000000000000000000, 0.9238795325112867385, 1.000000000000000000, 0.9238795325112867385, 1.000000000000000000, 0.9238795325112867385, 1.000000000000000000, 0.9238795325112867385, 1.000000000000000000, 0.9238795325112867385, 1.000000000000000000, 0.9238795325112867385, 1.000000000000000000, 0.9238795325112867385, 1.000000000000000000, 0.9238795325112867385, 1.000000000000000000, 0.9238795325112867385, 1.000000000000000000, 0.9238795325112867385, 1.000000000000000000, 0.9238795325112867385, 1.000000000000000000, 0.9238795325112867385, 1.000000000000000000, 0.9238795325112867385, 1.000000000000000000, 0.9238795325112867385, 1.000000000000000000, 0.9238795325112867385, 1.000000000000000000, 0.9238795325112867385, 1.000000000000000000, 0.9238795325112867385, 1.000000000000000000, 0.9238795325112867385, 1.000000000000000000, 0.9462258211652395667, 0.9684275895297407288),
 ( 1.000000000000000000, 0.9238795325112867385, 1.000000000000000000, 0.9238795325112867385, 1.000000000000000000, 0.9238795325112867385, 1.000000000000000000, 0.9238795325112867385, 1.000000000000000000, 0.9238795325112867385, 1.000000000000000000, 0.9238795325112867385, 1.000000000000000000, 0.9238795325112867385, 1.000000000000000000, 0.9238795325112867385, 1.000000000000000000, 0.9238795325112867385, 1.000000000000000000, 0.9238795325112867385, 1.000000000000000000, 0.9238795325112867385, 1.000000000000000000, 0.9238795325112867385, 1.000000000000000000, 0.9238795325112867385, 1.000000000000000000, 0.9238795325112867385, 1.000000000000000000, 0.9238795325112867385, 1.000000000000000000, 0.9238795325112867385, 1.000000000000000000, 0.9238795325112867385, 1.000000000000000000, 0.9238795325112867385, 1.000000000000000000, 0.9238795325112867385, 1.000000000000000000, 0.9238795325112867385, 1.000000000000000000, 0.9238795325112867385, 1.000000000000000000, 0.9238795325112867385, 1.000000000000000000, 0.9238795325112867385, 1.000000000000000000, 0.9238795325112867385, 1.000000000000000000, 0.9238795325112867385, 1.000000000000000000, 0.9238795325112867385, 1.000000000000000000, 0.9238795325112867385, 1.000000000000000000, 0.9238795325112867385, 1.000000000000000000, 0.9238795325112867385, 1.000000000000000000, 0.9238795325112867385, 1.000000000000000000, 0.9238795325112867385, 1.000000000000000000, 0.9238795325112867385, 1.000000000000000000, 0.9238795325112867385, 1.000000000000000000, 0.9238795325112867385, 1.000000000000000000, 0.9238795325112867385, 1.000000000000000000, 0.9238795325112867385, 1.000000000000000000, 0.9238795325112867385, 1.000000000000000000, 0.9238795325112867385, 1.000000000000000000, 0.9238795325112867385, 1.000000000000000000, 0.9238795325112867385, 1.000000000000000000, 0.9238795325112867385, 1.000000000000000000, 0.9238795325112867385, 1.000000000000000000, 0.9238795325112867385, 1.000000000000000000, 0.9238795325112867385, 1.000000000000000000, 0.9238795325112867385, 1.000000000000000000, 0.9238795325112867385, 1.000000000000000000, 0.9238795325112867385, 1.000000000000000000, 0.9238795325112867385, 1.000000000000000000, 0.9238795325112867385, 1.000000000000000000, 0.9238795325112867385, 1.000000000000000000, 0.9238795325112867385, 1.000000000000000000, 0.9238795325112867385, 1.000000000000000000, 0.9238795325112867385, 1.000000000000000000, 0.9238795325112867385, 1.000000000000000000, 0.9238795325112867385, 1.000000000000000000, 0.9238795325112867385, 1.000000000000000000, 0.9238795325112867385, 1.000000000000000000, 0.9238795325112867385, 1.000000000000000000, 0.9238795325112867385, 1.000000000000000000, 0.9238795325112867385, 1.000000000000000000, 0.9238795325112867385, 1.000000000000000000, 0.9238795325112867385, 1.000000000000000000, 0.9238795325112867385, 1.000000000000000000, 0.9238795325112867385, 1.000000000000000000, 0.9238795325112867385, 1.000000000000000000, 0.9238795325112867385, 1.000000000000000000, 0.9238795325112867385, 1.000000000000000000, 0.9238795325112867385, 1.000000000000000000, 0.9238795325112867385, 1.000000000000000000, 0.9238795325112867385, 1.000000000000000000, 0.9238795325112867385, 1.000000000000000000, 0.9238795325112867385, 1.000000000000000000, 0.9238795325112867385, 1.000000000000000000, 0.9238795325112867385, 1.000000000000000000, 0.9238795325112867385, 1.000000000000000000, 0.9238795325112867385, 1.000000000000000000, 0.9238795325112867385, 1.000000000000000000, 0.9238795325112867385, 1.000000000000000000, 0.9238795325112867385, 1.000000000000000000, 0.9238795325112867385, 1.000000000000000000, 0.9238795325112867385, 1.000000000000000000, 0.9238795325112867385, 1.000000000000000000, 0.9238795325112867385, 1.000000000000000000, 0.9238795325112867385, 1.000000000000000000, 0.9238795325112867385, 1.000000000000000000, 0.9238795325112867385, 1.000000000000000000, 0.9238795325112867385, 1.000000000000000000, 0.9238795325112867385, 1.000000000000000000, 0.9238795325112867385, 1.000000000000000000, 0.9238795325112867385, 1.000000000000000000, 0.9462258211652395667, 0.9684275895297407288) ) ) 
 REPRESENTATION_ITEM ( '' )  SURFACE ( )  );
#16266=ADVANCED_FACE ( 'NONE', ( #8946 ), #13343, .T. ) ;
#16268=CARTESIAN_POINT ( 'NONE',  ( 185.7049497278729575, 33.31054687608393294, -9.295050272127046043 ) ) ;
#16270=CARTESIAN_POINT ( 'NONE',  ( 192.9753722744670767, 50.00000000050955862, -13.43320860980940701 ) ) ;
#16272=ORIENTED_EDGE ( 'NONE', *, *, #13648, .T. ) ;
#16275=LINE ( 'NONE', #7865, #11297 ) ;
#16276=CARTESIAN_POINT ( 'NONE',  ( 9.598844408820459861, 38.91640624999999432, 9.598844408820456309 ) ) ;
#16278=CARTESIAN_POINT ( 'NONE',  ( 120.7049497278729575, 37.47773437608393010, 9.295050272127047819 ) ) ;
#16279=CARTESIAN_POINT ( 'NONE',  ( 2.414731522848535132E-15, 38.56914062608393579, 13.14518615778179544 ) ) ;
#16280=CARTESIAN_POINT ( 'NONE',  ( 13.14518615778179544, 40.35507812608393863, -1.609821015232357215E-15 ) ) ;
#16282=CARTESIAN_POINT ( 'NONE',  ( -5.622872871577736298, 36.18789062716787441, -13.57481594606318254 ) ) ;
#16284=DIRECTION ( 'NONE',  ( 0.000000000000000000, -1.000000000000000000, 0.000000000000000000 ) ) ;
#16287=CARTESIAN_POINT ( 'NONE',  ( 101.8468681455907046, 84.37500000136563472, -4.458734125000016313 ) ) ;
#16288=CARTESIAN_POINT ( 'NONE',  ( 95.54126587499996504, 84.56250000136560629, -1.387778780781445676E-14 ) ) ;
#16289=DIRECTION ( 'NONE',  ( -0.000000000000000000, 1.000000000000000000, -0.000000000000000000 ) ) ;
#16290=CARTESIAN_POINT ( 'NONE',  ( 195.0000000000000000, 37.18007812608393436, -13.14518615778179544 ) ) ;
#16295=DIRECTION ( 'NONE',  ( 0.000000000000000000, 0.000000000000000000, -1.000000000000000000 ) ) ;
#16296=EDGE_CURVE ( 'NONE', #10395, #21810, #19335, .T. ) ;
#16301=ORIENTED_EDGE ( 'NONE', *, *, #21526, .F. ) ;
#16304=ORIENTED_EDGE ( 'NONE', *, *, #25372, .T. ) ;
#16305=ADVANCED_FACE ( 'NONE', ( #16353 ), #9513, .T. ) ;
#16308=CARTESIAN_POINT ( 'NONE',  ( 200.4449143864723055, 33.36015625108393579, -13.14518615778179900 ) ) ;
#16314=EDGE_CURVE ( 'NONE', #24113, #17588, #24084, .T. ) ;
#16315=CARTESIAN_POINT ( 'NONE',  ( 116.4251840539369596, 38.71796875216787726, 0.000000000000000000 ) ) ;
#16318=CARTESIAN_POINT ( 'NONE',  ( 181.8548138422181921, 39.11484375108394573, -5.444914386472297529 ) ) ;
#16321=CARTESIAN_POINT ( 'NONE',  ( -2.892062521303301548, 36.00000000000000711, -13.15766692561478024 ) ) ;
#16323=AXIS2_PLACEMENT_3D ( 'NONE', #6506, #15181, #4379 ) ;
#16324=AXIS2_PLACEMENT_3D ( 'NONE', #838, #1397, #12049 ) ;
#16325=CARTESIAN_POINT ( 'NONE',  ( -3.136173621348210983, 36.00000000000000711, 12.79489613812742554 ) ) ;
#16326=CARTESIAN_POINT ( 'NONE',  ( 78.14518615778179367, 32.41757812608393863, -1.609821015232357215E-15 ) ) ;
#16329=CARTESIAN_POINT ( 'NONE',  ( 5.622872871577863307, 40.45429687500001137, 13.57481594606306174 ) ) ;
#16330=VECTOR ( 'NONE', #1543, 1000.000000000000000 ) ;
#16331=DIRECTION ( 'NONE',  ( 1.000000000000000000, -0.000000000000000000, -7.228014483236696740E-18 ) ) ;
#16332=CARTESIAN_POINT ( 'NONE',  ( 4.504887086316609945, 51.44650206077173493, 15.00000000000000000 ) ) ;
#16333=CARTESIAN_POINT ( 'NONE',  ( 135.6228728715778971, 34.10429687499999574, 13.57481594606304576 ) ) ;
#16334=EDGE_LOOP ( 'NONE', ( #16716, #26033, #5348, #27754 ) ) ;
#16335=DIRECTION ( 'NONE',  ( 0.000000000000000000, -0.000000000000000000, 1.000000000000000000 ) ) ;
#16339=CARTESIAN_POINT ( 'NONE',  ( 135.4449143864723055, 40.50390625108394005, -13.14518615778179900 ) ) ;
#16340=CARTESIAN_POINT ( 'NONE',  ( 51.42518405393695957, 31.62382812716787228, 5.622872871577880183 ) ) ;
#16342=CARTESIAN_POINT ( 'NONE',  ( 55.40115559117954547, 37.03125000216787299, -9.598844408820458085 ) ) ;
#16343=CARTESIAN_POINT ( 'NONE',  ( -13.14518615778179189, 37.42812500108393436, 5.444914386472304635 ) ) ;
#16344=CARTESIAN_POINT ( 'NONE',  ( 65.00000000000000000, 50.00000000000000000, -7.517135062566165128E-15 ) ) ;
#16348=CARTESIAN_POINT ( 'NONE',  ( -13.14518615778179900, 40.50390625108394005, -5.444914386472297529 ) ) ;
#16349=LINE ( 'NONE', #18770, #4276 ) ;
#16353=FACE_OUTER_BOUND ( 'NONE', #26456, .T. ) ;
#16363=CARTESIAN_POINT ( 'NONE',  ( 101.8468681455906903, 83.12500000136560629, -4.458734125000016313 ) ) ;
#16364=CARTESIAN_POINT ( 'NONE',  ( 59.55508561352770158, 40.60312500108393863, -13.14518615778179900 ) ) ;
#16366=CARTESIAN_POINT ( 'NONE',  ( 13.57481594606304576, 37.42812499999999432, -1.662435489736055892E-15 ) ) ;
#16367=CARTESIAN_POINT ( 'NONE',  ( 13.57481594606304931, 34.20351562499999432, 5.622872871577869525 ) ) ;
#16369=CARTESIAN_POINT ( 'NONE',  ( 120.7049497278729575, 35.29492187608393294, 9.295050272127047819 ) ) ;
#16371=CARTESIAN_POINT ( 'NONE',  ( 9.180175813647991845, 55.00000000000000000, -14.99999999999999822 ) ) ;
#16373=CARTESIAN_POINT ( 'NONE',  ( 94.99999999999995737, 79.18750000273121259, 2.071067811865466624 ) ) ;
#16376=CARTESIAN_POINT ( 'NONE',  ( 55.40115559117954547, 39.61093750216787868, 9.598844408820459861 ) ) ;
#16378=CARTESIAN_POINT ( 'NONE',  ( 185.7049497278729575, 40.65273437608393436, -9.295050272127046043 ) ) ;
#16379=CARTESIAN_POINT ( 'NONE',  ( 9.598844408820456309, 40.00781250216787299, -9.598844408820458085 ) ) ;
#16380=ORIENTED_EDGE ( 'NONE', *, *, #26391, .T. ) ;
#16383=ORIENTED_EDGE ( 'NONE', *, *, #6824, .T. ) ;
#16385=CARTESIAN_POINT ( 'NONE',  ( 200.6228728715778686, 32.91367187716787157, -13.57481594606304753 ) ) ;
#16387=DIRECTION ( 'NONE',  ( -0.000000000000000000, 1.000000000000000000, -0.000000000000000000 ) ) ;
#16389=CARTESIAN_POINT ( 'NONE',  ( 116.8548138422182205, 39.80937500108393579, 5.444914386472304635 ) ) ;
#16391=ADVANCED_FACE ( 'NONE', ( #10061 ), #25324, .F. ) ;
#16392=CYLINDRICAL_SURFACE ( 'NONE', #21812, 13.57481594606304398 ) ;
#16395=CARTESIAN_POINT ( 'NONE',  ( 181.4251840539369596, 40.25585937499999289, 5.622872871577880183 ) ) ;
#16399=CARTESIAN_POINT ( 'NONE',  ( -5.622872871577964560, 37.77539062716787299, -13.57481594606295339 ) ) ;
#16406=CARTESIAN_POINT ( 'NONE',  ( -5.444914386472299306, 32.96328125108393436, 13.14518615778179722 ) ) ;
#16409=CARTESIAN_POINT ( 'NONE',  ( -13.57481594606304753, 37.77539062499998579, -5.622872871577872189 ) ) ;
#16410=CARTESIAN_POINT ( 'NONE',  ( 195.0000000000000000, 32.81445312608393294, 13.14518615778179544 ) ) ;
#16412=CARTESIAN_POINT ( 'NONE',  ( 196.1387681171055419, 50.00000000043849013, -13.56816686242531667 ) ) ;
#16414=ORIENTED_EDGE ( 'NONE', *, *, #7706, .F. ) ;
#16417=DIRECTION ( 'NONE',  ( 0.000000000000000000, 0.000000000000000000, 1.000000000000000000 ) ) ;
#16419=CARTESIAN_POINT ( 'NONE',  ( 9.295050272127046043, 38.86679687608393863, -9.295050272127046043 ) ) ;
#16420=CARTESIAN_POINT ( 'NONE',  ( -13.14518615778179544, 40.75195312608393294, 0.000000000000000000 ) ) ;
#16422=DIRECTION ( 'NONE',  ( -0.000000000000000000, 1.000000000000000000, -0.000000000000000000 ) ) ;
#16423=CARTESIAN_POINT ( 'NONE',  ( 0.000000000000000000, 50.00000000000000000, 0.000000000000000000 ) ) ;
#16424=( BOUNDED_CURVE ( )  B_SPLINE_CURVE ( 2, ( #5913, #18734, #10295, #27432, #19001, #7896, #27713, #25284, #5770 ),
 .UNSPECIFIED., .F., .T. ) 
 B_SPLINE_CURVE_WITH_KNOTS ( ( 3, 2, 2, 2, 3 ),
 ( 0.3541666666666666852, 0.3645833333333332593, 0.3749999999999998890, 0.3854166666666665741, 0.3958333333333331483 ),
 .UNSPECIFIED. ) 
 CURVE ( )  GEOMETRIC_REPRESENTATION_ITEM ( )  RATIONAL_B_SPLINE_CURVE ( ( 1.000000000000000000, 0.9238795325112867385, 1.000000000000000000, 0.9238795325112867385, 1.000000000000000000, 0.9238795325112867385, 1.000000000000000000, 0.9238795325112879597, 0.9999999999999987788 ) ) 
 REPRESENTATION_ITEM ( '' )  );
#16427=CARTESIAN_POINT ( 'NONE',  ( 104.4587341249999639, 82.18750000136559208, -1.442382525525748735E-14 ) ) ;
#16428=PLANE ( 'NONE',  #26337 ) ;
#16430=VERTEX_POINT ( 'NONE', #8349 ) ;
#16434=CARTESIAN_POINT ( 'NONE',  ( 189.5550856135277229, 36.13828125108393152, 13.14518615778179722 ) ) ;
#16438=ORIENTED_EDGE ( 'NONE', *, *, #6239, .F. ) ;
#16439=DIRECTION ( 'NONE',  ( 0.000000000000000000, -0.000000000000000000, 1.000000000000000000 ) ) ;
#16440=CARTESIAN_POINT ( 'NONE',  ( 51.85481384221821344, 36.83281250108393579, 5.444914386472304635 ) ) ;
#16442=CARTESIAN_POINT ( 'NONE',  ( -9.598844408820458085, 39.31328124999999574, -9.598844408820458085 ) ) ;
#16444=ORIENTED_EDGE ( 'NONE', *, *, #18574, .F. ) ;
#16445=CARTESIAN_POINT ( 'NONE',  ( 70.62287287157786864, 37.57695312499999574, -13.57481594606304753 ) ) ;
#16446=CARTESIAN_POINT ( 'NONE',  ( 8.758334392354081288, 50.00000000000000000, -10.38725784494425675 ) ) ;
#16448=CARTESIAN_POINT ( 'NONE',  ( 139.5988444088204687, 39.01562500216787299, 9.598844408820456309 ) ) ;
#16449=DIRECTION ( 'NONE',  ( 0.000000000000000000, 0.000000000000000000, -1.000000000000000000 ) ) ;
#16452=CARTESIAN_POINT ( 'NONE',  ( 181.8548138422181921, 36.83281250108393579, 5.444914386472304635 ) ) ;
#16454=EDGE_CURVE ( 'NONE', #11953, #2183, #56, .T. ) ;
#16455=ORIENTED_EDGE ( 'NONE', *, *, #24130, .F. ) ;
#16457=DIRECTION ( 'NONE',  ( 0.000000000000000000, -1.000000000000000000, 0.000000000000000000 ) ) ;
#16460=CARTESIAN_POINT ( 'NONE',  ( 103.1528011352953342, 83.81250000136560629, 3.152801135295355106 ) ) ;
#16465=CARTESIAN_POINT ( 'NONE',  ( 12.89215161363577344, 36.00000000000001421, -4.169510824906851099 ) ) ;
#16466=CARTESIAN_POINT ( 'NONE',  ( 9.180175813648009608, 49.99999999999999289, 14.99999999999999822 ) ) ;
#16467=CARTESIAN_POINT ( 'NONE',  ( 116.4251840539369596, 33.90585937500000568, 5.622872871577880183 ) ) ;
#16468=VERTEX_POINT ( 'NONE', #20735 ) ;
#16471=CARTESIAN_POINT ( 'NONE',  ( 74.59884440882045453, 36.73359374999999716, -9.598844408820458085 ) ) ;
#16475=CARTESIAN_POINT ( 'NONE',  ( 120.7049497278729575, 39.26367187608393294, 9.295050272127047819 ) ) ;
#16476=CARTESIAN_POINT ( 'NONE',  ( 78.14518615778179367, 39.36289062608393152, -1.609821015232357215E-15 ) ) ;
#16478=CARTESIAN_POINT ( 'NONE',  ( 60.62597786918168197, 36.00000000000000711, 12.40367315690567196 ) ) ;
#16479=CARTESIAN_POINT ( 'NONE',  ( 9.295050272127046043, 38.66835937608393436, -9.295050272127046043 ) ) ;
#16482=ADVANCED_FACE ( 'NONE', ( #5346 ), #27016, .F. ) ;
#16487=CARTESIAN_POINT ( 'NONE',  ( 141.2065315021356469, 36.00000000000001421, 7.323573988461032691 ) ) ;
#16489=EDGE_CURVE ( 'NONE', #7335, #18339, #18858, .T. ) ;
#16496=ORIENTED_EDGE ( 'NONE', *, *, #18439, .T. ) ;
#16502=AXIS2_PLACEMENT_3D ( 'NONE', #25566, #14993, #15128 ) ;
#16505=CARTESIAN_POINT ( 'NONE',  ( 101.8468681455906903, 84.00000000136560629, 4.458734124999987891 ) ) ;
#16506=CARTESIAN_POINT ( 'NONE',  ( 74.29505027212704249, 40.45429687608393721, -9.295050272127046043 ) ) ;
#16513=CARTESIAN_POINT ( 'NONE',  ( 116.8548138422182063, 36.03906250108394005, 5.444914386472304635 ) ) ;
#16515=CARTESIAN_POINT ( 'NONE',  ( 139.5988444088204403, 37.62656250216787157, -9.598844408820458085 ) ) ;
#16516=CARTESIAN_POINT ( 'NONE',  ( 65.00000000000000000, 38.12265625216787157, 13.57481594606304576 ) ) ;
#16517=CARTESIAN_POINT ( 'NONE',  ( 95.54126587499995082, 84.37500000136562051, -1.846868145590750077 ) ) ;
#16518=CARTESIAN_POINT ( 'NONE',  ( 143.1451861577818079, 38.61875000108393152, -5.444914386472297529 ) ) ;
#16519=CARTESIAN_POINT ( 'NONE',  ( 51.84732309041283571, 36.00000000000001421, 0.5874252385153132527 ) ) ;
#16521=CARTESIAN_POINT ( 'NONE',  ( -9.598844408820454532, 38.81718750216787583, 9.598844408820459861 ) ) ;
#16527=CARTESIAN_POINT ( 'NONE',  ( 204.2950502721270425, 39.26367187608393294, 9.295050272127046043 ) ) ;
#16528=CARTESIAN_POINT ( 'NONE',  ( -8.312177448680279460E-16, 36.93203125216787441, -13.57481594606304576 ) ) ;
#16530=CARTESIAN_POINT ( 'NONE',  ( 120.7049497278729575, 38.27148437608393294, 9.295050272127047819 ) ) ;
#16536=CARTESIAN_POINT ( 'NONE',  ( 181.4251840539369596, 39.36289062499999858, -5.622872871577873077 ) ) ;
#16539=CARTESIAN_POINT ( 'NONE',  ( 127.7020394139926651, 36.00000000000000000, 12.97104423350695690 ) ) ;
#16541=CARTESIAN_POINT ( 'NONE',  ( 195.0000000000000000, 36.83281249999999574, -13.57481594606304576 ) ) ;
#16547=CARTESIAN_POINT ( 'NONE',  ( -5.444914386472299306, 34.55078125108393294, 13.14518615778179722 ) ) ;
#16548=VERTEX_POINT ( 'NONE', #5628 ) ;
#16549=CARTESIAN_POINT ( 'NONE',  ( 96.84719886470459471, 81.81250000136559208, 3.152801135295355994 ) ) ;
#16551=CARTESIAN_POINT ( 'NONE',  ( 200.4449143864723055, 33.16171875108393152, -13.14518615778179900 ) ) ;
#16552=VERTEX_POINT ( 'NONE', #23150 ) ;
#16554=CARTESIAN_POINT ( 'NONE',  ( 193.4945078184423153, 53.60078691996476152, -15.00000000000000000 ) ) ;
#16561=CARTESIAN_POINT ( 'NONE',  ( 5.444914386472302859, 37.03125000108393294, 13.14518615778179189 ) ) ;
#16562=CIRCLE ( 'NONE', #21570, 4.999999999999997335 ) ;
#16563=CARTESIAN_POINT ( 'NONE',  ( -13.14518615778179189, 32.66562500108393863, 5.444914386472304635 ) ) ;
#16569=CARTESIAN_POINT ( 'NONE',  ( 130.0000000000000000, 50.00000000000000000, -1.503427012513233026E-14 ) ) ;
#16571=CARTESIAN_POINT ( 'NONE',  ( 181.4251840539369596, 38.61874999999999147, 0.000000000000000000 ) ) ;
#16579=EDGE_CURVE ( 'NONE', #16552, #2330, #25087, .T. ) ;
#16582=ORIENTED_EDGE ( 'NONE', *, *, #24638, .T. ) ;
#16583=CARTESIAN_POINT ( 'NONE',  ( 59.55508561352770158, 36.63437500108393863, -13.14518615778179722 ) ) ;
#16588=VECTOR ( 'NONE', #17553, 1000.000000000000000 ) ;
#16589=CARTESIAN_POINT ( 'NONE',  ( -4.858499290463643483, 49.99999999891524283, -12.70434618648844705 ) ) ;
#16590=CARTESIAN_POINT ( 'NONE',  ( 198.0393970508025063, 53.88964894337311051, 14.99999999999994671 ) ) ;
#16591=CARTESIAN_POINT ( 'NONE',  ( 124.3771271284221314, 34.60039062716786873, -13.57481594606304753 ) ) ;
#16595=CARTESIAN_POINT ( 'NONE',  ( 189.5550856135277229, 36.93203125108394147, 13.14518615778179722 ) ) ;
#16602=CARTESIAN_POINT ( 'NONE',  ( 95.54126587499996504, 83.50000000136560629, 1.846868145590724986 ) ) ;
#16604=( LENGTH_UNIT ( ) NAMED_UNIT ( * ) SI_UNIT ( .MILLI., .METRE. ) );
#16606=CARTESIAN_POINT ( 'NONE',  ( 95.54126587499996504, 79.68750000136559208, -1.387778780781445676E-14 ) ) ;
#16608=CARTESIAN_POINT ( 'NONE',  ( 94.99999999999995737, 82.93750000000001421, -2.071067811865491493 ) ) ;
#16617=CARTESIAN_POINT ( 'NONE',  ( 116.8548138422182063, 39.90859375108394147, -5.444914386472297529 ) ) ;
#16619=CARTESIAN_POINT ( 'NONE',  ( 51.85481384221820633, 35.84062500108394289, 5.444914386472304635 ) ) ;
#16621=CARTESIAN_POINT ( 'NONE',  ( 1.137167824540872951, 35.99999999999998579, 13.09590655363602707 ) ) ;
#16622=CARTESIAN_POINT ( 'NONE',  ( 9.295050272127047819, 34.50117187608393010, 9.295050272127046043 ) ) ;
#16625=LINE ( 'NONE', #8204, #24461 ) ;
#16626=CARTESIAN_POINT ( 'NONE',  ( -15.00000000000000000, 75.00000000000000000, 10.00000000000000000 ) ) ;
#16627=CARTESIAN_POINT ( 'NONE',  ( -9.295050272127044266, 37.47773437608393010, 9.295050272127047819 ) ) ;
#16630=EDGE_CURVE ( 'NONE', #7460, #17097, #25914, .T. ) ;
#16632=CARTESIAN_POINT ( 'NONE',  ( 181.4251840539369596, 39.46210937499999005, 5.622872871577880183 ) ) ;
#16636=AXIS2_PLACEMENT_3D ( 'NONE', #18898, #27608, #8066 ) ;
#16643=CARTESIAN_POINT ( 'NONE',  ( 98.15313185440925281, 80.62500000136559208, 4.458734124999987891 ) ) ;
#16644=CARTESIAN_POINT ( 'NONE',  ( 74.29505027212704249, 37.27929687608394005, -9.295050272127046043 ) ) ;
#16646=DIRECTION ( 'NONE',  ( 0.8660254037844407060, 0.4999999999999963363, 0.000000000000000000 ) ) ;
#16647=DIRECTION ( 'NONE',  ( 0.000000000000000000, -1.000000000000000000, -0.000000000000000000 ) ) ;
#16648=DIRECTION ( 'NONE',  ( 1.000000000000000000, 0.000000000000000000, -7.228014483236696740E-18 ) ) ;
#16650=CARTESIAN_POINT ( 'NONE',  ( 116.8548138422182063, 35.24531250108393721, 5.444914386472304635 ) ) ;
#16651=EDGE_CURVE ( 'NONE', #1089, #3050, #24640, .T. ) ;
#16652=ORIENTED_EDGE ( 'NONE', *, *, #12250, .T. ) ;
#16653=FACE_OUTER_BOUND ( 'NONE', #12899, .T. ) ;
#16656=CARTESIAN_POINT ( 'NONE',  ( 143.1451861577818079, 39.31328125108392868, 5.444914386472293977 ) ) ;
#16658=CARTESIAN_POINT ( 'NONE',  ( 78.57481594606304043, 35.98945312716787015, -5.622872871577873077 ) ) ;
#16660=CARTESIAN_POINT ( 'NONE',  ( 13.57481594606304576, 38.32109375216786873, -1.662435489736055892E-15 ) ) ;
#16667=CARTESIAN_POINT ( 'NONE',  ( 185.4011555911795313, 31.47500000216787441, -9.598844408820458085 ) ) ;
#16669=CARTESIAN_POINT ( 'NONE',  ( 124.5550856135277087, 38.32109375108394289, 13.14518615778179722 ) ) ;
#16670=CARTESIAN_POINT ( 'NONE',  ( -13.14518615778179189, 32.86406250108393579, 5.444914386472304635 ) ) ;
#16674=CARTESIAN_POINT ( 'NONE',  ( 189.3771271284221314, 37.18007812500000853, 13.57481594606304753 ) ) ;
#16675=CARTESIAN_POINT ( 'NONE',  ( 99.99999999999995737, 85.00000000000000000, -5.000000000000018652 ) ) ;
#16677=CARTESIAN_POINT ( 'NONE',  ( 65.00000000000000000, 38.76757812608393294, -13.14518615778179544 ) ) ;
#16681=CIRCLE ( 'NONE', #2591, 4.999999999999999112 ) ;
#16682=CARTESIAN_POINT ( 'NONE',  ( 204.5988444088204687, 39.71015624999999716, 9.598844408820456309 ) ) ;
#16684=CARTESIAN_POINT ( 'NONE',  ( 9.598844408820459861, 40.50390624999999289, 9.598844408820456309 ) ) ;
#16686=CARTESIAN_POINT ( 'NONE',  ( 103.1528011352953342, 83.31250000136560629, -3.152801135295383084 ) ) ;
#16687=CARTESIAN_POINT ( 'NONE',  ( 195.0000000000000000, -7.395377635281828788, -13.57481594606306707 ) ) ;
#16689=ORIENTED_EDGE ( 'NONE', *, *, #15254, .T. ) ;
#16691=CARTESIAN_POINT ( 'NONE',  ( 185.8198241863519229, 49.99999999999996447, -15.00000000000000000 ) ) ;
#16694=ORIENTED_EDGE ( 'NONE', *, *, #21317, .T. ) ;
#16698=CARTESIAN_POINT ( 'NONE',  ( 99.99999999999995737, 85.00000000000000000, -5.000000000000018652 ) ) ;
#16702=CARTESIAN_POINT ( 'NONE',  ( 143.1451861577818363, 38.71796875108393721, 5.444914386472293977 ) ) ;
#16703=CARTESIAN_POINT ( 'NONE',  ( 13.14518615778179900, 32.16953125108393152, 5.444914386472293977 ) ) ;
#16705=CARTESIAN_POINT ( 'NONE',  ( 55.40115559117954547, 39.31328124999999574, -9.598844408820458085 ) ) ;
#16707=CARTESIAN_POINT ( 'NONE',  ( 78.57481594606305464, 38.27148437500000711, -5.622872871577873966 ) ) ;
#16712=CARTESIAN_POINT ( 'NONE',  ( 98.15313185440923860, 83.87500000136560629, 4.458734124999987891 ) ) ;
#16714=FACE_OUTER_BOUND ( 'NONE', #17707, .T. ) ;
#16715=CARTESIAN_POINT ( 'NONE',  ( 185.4011555911795313, 38.51953124999999289, -9.598844408820458085 ) ) ;
#16716=ORIENTED_EDGE ( 'NONE', *, *, #11191, .T. ) ;
#16718=( BOUNDED_CURVE ( )  B_SPLINE_CURVE ( 2, ( #5554, #24499, #3128, #22798, #999, #24783, #9809, #9668, #18371 ),
 .UNSPECIFIED., .F., .F. ) 
 B_SPLINE_CURVE_WITH_KNOTS ( ( 3, 2, 2, 2, 3 ),
 ( 0.2291666666666665741, 0.2395833333333332316, 0.2499999999999998335, 0.2604166666666665186, 0.2708333333333330928 ),
 .UNSPECIFIED. ) 
 CURVE ( )  GEOMETRIC_REPRESENTATION_ITEM ( )  RATIONAL_B_SPLINE_CURVE ( ( 1.000000000000000666, 0.9238795325112861834, 1.000000000000000000, 0.9238795325112867385, 1.000000000000000000, 0.9238795325112867385, 1.000000000000000000, 0.9238795325112884038, 0.9999999999999983347 ) ) 
 REPRESENTATION_ITEM ( '' )  );
#16725=CARTESIAN_POINT ( 'NONE',  ( 65.00000000000000000, 38.17226562608394147, -13.14518615778179544 ) ) ;
#16730=CARTESIAN_POINT ( 'NONE',  ( -7.621963534194025947, 54.91641323977498246, -15.00000000000000000 ) ) ;
#16732=CARTESIAN_POINT ( 'NONE',  ( 116.4251840539369596, 33.16171875216787868, 0.000000000000000000 ) ) ;
#16733=DIRECTION ( 'NONE',  ( 0.000000000000000000, 0.000000000000000000, 1.000000000000000000 ) ) ;
#16735=CARTESIAN_POINT ( 'NONE',  ( 204.2950502721270425, 37.87460937608393863, 9.295050272127046043 ) ) ;
#16736=ORIENTED_EDGE ( 'NONE', *, *, #9081, .T. ) ;
#16737=ADVANCED_FACE ( 'NONE', ( #23424 ), #2186, .T. ) ;
#16740=CARTESIAN_POINT ( 'NONE',  ( 5.622872871577786924, 38.07304687499999574, 13.57481594606313813 ) ) ;
#16745=CARTESIAN_POINT ( 'NONE',  ( 13.01985494039037050, 36.00000000000000711, 3.369129453356577208 ) ) ;
#16752=CARTESIAN_POINT ( 'NONE',  ( 135.4449143864723055, 39.41250000108393436, 13.14518615778179189 ) ) ;
#16753=CARTESIAN_POINT ( 'NONE',  ( 55.70494972787295751, 35.89023437608393152, 9.295050272127047819 ) ) ;
#16756=CARTESIAN_POINT ( 'NONE',  ( -9.295050272127046043, 36.48554687608393721, -9.295050272127046043 ) ) ;
#16757=CARTESIAN_POINT ( 'NONE',  ( 185.1606183911117967, 36.00000000000000711, -9.004033604612759589 ) ) ;
#16759=CARTESIAN_POINT ( 'NONE',  ( -15.00000000000000355, 80.00000000000000000, -9.999999999999998224 ) ) ;
#16761=LINE ( 'NONE', #25462, #8427 ) ;
#16762=CARTESIAN_POINT ( 'NONE',  ( -9.295050272127044266, 38.27148437608393294, 9.295050272127047819 ) ) ;
#16763=CARTESIAN_POINT ( 'NONE',  ( 137.7541239759952703, 36.00000000000000000, 10.77549638133723953 ) ) ;
#16765=VECTOR ( 'NONE', #7783, 1000.000000000000000 ) ;
#16766=CARTESIAN_POINT ( 'NONE',  ( 65.00000000000000000, 40.00781250000000000, -13.57481594606304576 ) ) ;
#16772=ORIENTED_EDGE ( 'NONE', *, *, #2740, .F. ) ;
#16777=CARTESIAN_POINT ( 'NONE',  ( 185.4011555911795597, 36.43593750216787441, 9.598844408820459861 ) ) ;
#16778=CARTESIAN_POINT ( 'NONE',  ( 95.54126587499996504, 80.43750000136559208, -1.387778780781445676E-14 ) ) ;
#16779=CARTESIAN_POINT ( 'NONE',  ( 51.85481384221819923, 37.52734375108393294, -5.444914386472297529 ) ) ;
#16782=DIRECTION ( 'NONE',  ( 0.000000000000000000, 0.000000000000000000, 1.000000000000000000 ) ) ;
#16784=CARTESIAN_POINT ( 'NONE',  ( 51.42518405393695957, 38.66835937716787441, -5.622872871577872189 ) ) ;
#16786=CARTESIAN_POINT ( 'NONE',  ( 130.0000000000000000, 32.21914062608393436, 13.14518615778179544 ) ) ;
#16788=CARTESIAN_POINT ( 'NONE',  ( 130.0000000000000000, 37.32890625216786873, 13.57481594606304576 ) ) ;
#16790=CARTESIAN_POINT ( 'NONE',  ( 95.54126587499995082, 81.50000000136560629, 1.846868145590724986 ) ) ;
#16791=CARTESIAN_POINT ( 'NONE',  ( 116.8548138422182063, 38.22187500108393010, 5.444914386472304635 ) ) ;
#16792=CARTESIAN_POINT ( 'NONE',  ( 70.62287287157788285, 36.58476562716787583, 13.57481594606304576 ) ) ;
#16794=CIRCLE ( 'NONE', #14037, 5.000000000000000000 ) ;
#16795=CARTESIAN_POINT ( 'NONE',  ( 13.57481594606304576, 35.14609375216787157, -1.662435489736055892E-15 ) ) ;
#16801=CARTESIAN_POINT ( 'NONE',  ( 189.5550856135277229, 36.43593750108392726, -13.14518615778179900 ) ) ;
#16803=CARTESIAN_POINT ( 'NONE',  ( 130.0000000000000000, 37.18007812608393436, -13.14518615778179544 ) ) ;
#16805=CARTESIAN_POINT ( 'NONE',  ( 99.99999999999995737, 85.00000000000000000, -5.000000000000018652 ) ) ;
#16806=CARTESIAN_POINT ( 'NONE',  ( 130.0000000000000000, -7.395377635281828788, -1.503427012513233026E-14 ) ) ;
#16809=ADVANCED_FACE ( 'NONE', ( #4460 ), #19142, .T. ) ;
#16810=CARTESIAN_POINT ( 'NONE',  ( 204.5988444088204403, 37.52734375000000000, -9.598844408820458085 ) ) ;
#16814=CARTESIAN_POINT ( 'NONE',  ( 51.85481384221820633, 39.01562500108393294, 5.444914386472304635 ) ) ;
#16821=CARTESIAN_POINT ( 'NONE',  ( -9.598844408820458085, 40.10703124999999147, -9.598844408820458085 ) ) ;
#16822=CARTESIAN_POINT ( 'NONE',  ( 135.4449143864723055, 40.50390625108394005, -13.14518615778179900 ) ) ;
#16823=ADVANCED_FACE ( 'NONE', ( #27338 ), #18496, .F. ) ;
#16824=ORIENTED_EDGE ( 'NONE', *, *, #8435, .F. ) ;
#16825=CARTESIAN_POINT ( 'NONE',  ( 99.99999999999995737, 82.93750000136560629, 4.458734124999988779 ) ) ;
#16827=ORIENTED_EDGE ( 'NONE', *, *, #24638, .F. ) ;
#16829=ORIENTED_EDGE ( 'NONE', *, *, #15572, .T. ) ;
#16830=CARTESIAN_POINT ( 'NONE',  ( 128.1124712741236067, 53.66306546785492060, -15.00000000000000178 ) ) ;
#16835=CARTESIAN_POINT ( 'NONE',  ( 204.5988444088204403, 37.62656250216787157, -9.598844408820458085 ) ) ;
#16838=CARTESIAN_POINT ( 'NONE',  ( 194.1610731307196147, 53.50081894914376335, 14.99999999999994671 ) ) ;
#16839=CARTESIAN_POINT ( 'NONE',  ( 135.4449143864723339, 38.12265625108393863, -13.14518615778179722 ) ) ;
#16840=CARTESIAN_POINT ( 'NONE',  ( 9.295050272127047819, 32.91367187608393152, 9.295050272127046043 ) ) ;
#16842=CARTESIAN_POINT ( 'NONE',  ( 51.42518405393695957, 39.41249999999999432, 0.000000000000000000 ) ) ;
#16843=LINE ( 'NONE', #3606, #14122 ) ;
#16844=CARTESIAN_POINT ( 'NONE',  ( 205.5630829503605810, 36.00000000000001421, 8.196709705856925154 ) ) ;
#16849=CARTESIAN_POINT ( 'NONE',  ( -13.14518615778179544, 39.16445312608393436, 0.000000000000000000 ) ) ;
#16850=EDGE_CURVE ( 'NONE', #13418, #540, #12246, .T. ) ;
#16856=CARTESIAN_POINT ( 'NONE',  ( 195.0000000000000000, 36.18789062608393436, 13.14518615778179544 ) ) ;
#16857=CARTESIAN_POINT ( 'NONE',  ( -13.57481594606304576, 40.20624999999999005, 0.000000000000000000 ) ) ;
#16860=CARTESIAN_POINT ( 'NONE',  ( 74.29505027212704249, 37.08085937608393579, 9.295050272127046043 ) ) ;
#16862=CARTESIAN_POINT ( 'NONE',  ( 116.6399989480775901, 40.87597656304196647, 0.000000000000000000 ) ) ;
#16864=CARTESIAN_POINT ( 'NONE',  ( -15.00000000000000355, 55.00000000000000000, -10.00000000000000000 ) ) ;
#16865=CARTESIAN_POINT ( 'NONE',  ( 116.4251840539369738, 37.87460937499999147, 5.622872871577880183 ) ) ;
#16867=CARTESIAN_POINT ( 'NONE',  ( 130.0000000000000000, 35.34453125216787583, -13.57481594606304576 ) ) ;
#16872=CARTESIAN_POINT ( 'NONE',  ( 181.8548138422181921, 39.21406250108392300, 5.444914386472304635 ) ) ;
#16874=ORIENTED_EDGE ( 'NONE', *, *, #9081, .F. ) ;
#16876=CARTESIAN_POINT ( 'NONE',  ( 99.99999999999995737, 83.75000000000000000, -5.000000000000018652 ) ) ;
#16879=CARTESIAN_POINT ( 'NONE',  ( 130.0000000000000000, 39.71015625216787015, 13.57481594606304576 ) ) ;
#16882=CARTESIAN_POINT ( 'NONE',  ( 120.4011555911795455, 32.16953124999999147, -9.598844408820458085 ) ) ;
#16887=CARTESIAN_POINT ( 'NONE',  ( 143.1451861577818079, 38.71796875108393721, 5.444914386472293977 ) ) ;
#16888=CARTESIAN_POINT ( 'NONE',  ( 70.44491438647230552, 37.13046875108393152, -13.14518615778179900 ) ) ;
#16889=CARTESIAN_POINT ( 'NONE',  ( 200.4449143864723055, 32.07031250108393294, 13.14518615778179189 ) ) ;
#16891=CARTESIAN_POINT ( 'NONE',  ( 130.0000000000000000, 40.40468749999999432, 13.57481594606304576 ) ) ;
#16892=CARTESIAN_POINT ( 'NONE',  ( -8.049105076161786076E-16, 35.59257812608393579, -13.14518615778179544 ) ) ;
#16893=CARTESIAN_POINT ( 'NONE',  ( 198.6286142932848691, 36.00000000000000000, -13.08307257738122686 ) ) ;
#16895=FACE_OUTER_BOUND ( 'NONE', #14997, .T. ) ;
#16896=CARTESIAN_POINT ( 'NONE',  ( -13.14518615778179900, 37.32890625108393579, -5.444914386472297529 ) ) ;
#16904=VERTEX_POINT ( 'NONE', #23192 ) ;
#16910=CARTESIAN_POINT ( 'NONE',  ( 98.15313185440925281, 83.87500000136560629, 4.458734124999987891 ) ) ;
#16911=CARTESIAN_POINT ( 'NONE',  ( 59.55508561352770158, 38.51953125108393294, 13.14518615778179722 ) ) ;
#16915=CARTESIAN_POINT ( 'NONE',  ( 139.5988444088204687, 38.91640624999999432, 9.598844408820456309 ) ) ;
#16917=CARTESIAN_POINT ( 'NONE',  ( 135.6228728715778686, 39.16445312499999432, -13.57481594606304753 ) ) ;
#16918=VERTEX_POINT ( 'NONE', #1257 ) ;
#16923=CARTESIAN_POINT ( 'NONE',  ( 116.8548138422182205, 40.55351562608393579, 0.000000000000000000 ) ) ;
#16924=CARTESIAN_POINT ( 'NONE',  ( 78.57481594606305464, 36.73359375216787015, -1.662435489736055892E-15 ) ) ;
#16926=FACE_OUTER_BOUND ( 'NONE', #1520, .T. ) ;
#16927=CARTESIAN_POINT ( 'NONE',  ( -9.598844408820454532, 34.84843750216787583, 9.598844408820459861 ) ) ;
#16930=CARTESIAN_POINT ( 'NONE',  ( 204.2950502721270425, 36.08867187608392868, 9.295050272127046043 ) ) ;
#16931=DIRECTION ( 'NONE',  ( 0.000000000000000000, 0.000000000000000000, 1.000000000000000000 ) ) ;
#16932=CARTESIAN_POINT ( 'NONE',  ( 124.5550856135277087, 39.11484375108393863, 13.14518615778179722 ) ) ;
#16936=CARTESIAN_POINT ( 'NONE',  ( 195.0000000000000000, 52.00000000000000711, -2.255140518769849538E-14 ) ) ;
#16938=CARTESIAN_POINT ( 'NONE',  ( 181.4251840539369596, 37.03124999999999289, 0.000000000000000000 ) ) ;
#16941=CARTESIAN_POINT ( 'NONE',  ( 78.14518615778179367, 37.82500000108392868, -5.444914386472297529 ) ) ;
#16946=CARTESIAN_POINT ( 'NONE',  ( -5.622872871577873077, 38.76757812500000000, 13.57481594606304753 ) ) ;
#16947=CARTESIAN_POINT ( 'NONE',  ( 124.5550856135277087, 39.80937500108392868, -13.14518615778179900 ) ) ;
#16949=CARTESIAN_POINT ( 'NONE',  ( 104.4587341249999639, 82.18750000136559208, -1.442382525525748735E-14 ) ) ;
#16950=EDGE_CURVE ( 'NONE', #23060, #10301, #12518, .T. ) ;
#16954=DIRECTION ( 'NONE',  ( 1.000000000000000000, 0.000000000000000000, -7.228014483236696740E-18 ) ) ;
#16955=CARTESIAN_POINT ( 'NONE',  ( 59.55508561352770158, 35.34453125108393579, 13.14518615778179722 ) ) ;
#16956=EDGE_LOOP ( 'NONE', ( #25172, #21256, #16444, #16824 ) ) ;
#16957=ADVANCED_FACE ( 'NONE', ( #1535 ), #10187, .T. ) ;
#16960=EDGE_CURVE ( 'NONE', #10089, #12843, #16761, .T. ) ;
#16964=CARTESIAN_POINT ( 'NONE',  ( 204.5988444088204687, 36.63437500216787157, 9.598844408820456309 ) ) ;
#16968=CARTESIAN_POINT ( 'NONE',  ( 204.1801758136480203, 50.00000000000000000, 9.999999999999946709 ) ) ;
#16969=CARTESIAN_POINT ( 'NONE',  ( 143.1451861577818079, 39.56132812608393579, -1.609821015232357215E-15 ) ) ;
#16970=CARTESIAN_POINT ( 'NONE',  ( 5.444914386472302859, 38.61875000108393152, 13.14518615778179189 ) ) ;
#16972=CARTESIAN_POINT ( 'NONE',  ( 65.00000000000000000, 36.83281249999999574, -13.57481594606304576 ) ) ;
#16973=CARTESIAN_POINT ( 'NONE',  ( 99.99999999999995737, 79.87500000273119838, -5.000000000000018652 ) ) ;
#16980=CARTESIAN_POINT ( 'NONE',  ( 95.54126587499996504, 79.68750000136559208, -1.387778780781445676E-14 ) ) ;
#16982=CARTESIAN_POINT ( 'NONE',  ( -5.444914386472297529, 38.22187500108393010, -13.14518615778179900 ) ) ;
#16986=CARTESIAN_POINT ( 'NONE',  ( 104.9999999999999716, 83.62500000273119838, -1.449011120738813565E-14 ) ) ;
#16988=EDGE_CURVE ( 'NONE', #18589, #1781, #13702, .T. ) ;
#16991=CARTESIAN_POINT ( 'NONE',  ( 78.14518615778179367, 38.76757812608393294, -1.609821015232357215E-15 ) ) ;
#16993=CARTESIAN_POINT ( 'NONE',  ( -13.57481594606304398, 39.46210937499999005, 5.622872871577880183 ) ) ;
#16994=AXIS2_PLACEMENT_3D ( 'NONE', #26051, #2267, #10927 ) ;
#16995=ORIENTED_EDGE ( 'NONE', *, *, #19102, .T. ) ;
#16999=ADVANCED_FACE ( 'NONE', ( #15271 ), #13410, .T. ) ;
#17000=CARTESIAN_POINT ( 'NONE',  ( 120.4011555911795455, 34.84843750216787583, 9.598844408820459861 ) ) ;
#17001=CARTESIAN_POINT ( 'NONE',  ( 204.2950502721270425, 35.49335937608393721, 9.295050272127046043 ) ) ;
#17002=VERTEX_POINT ( 'NONE', #6731 ) ;
#17004=ORIENTED_EDGE ( 'NONE', *, *, #16950, .F. ) ;
#17008=CARTESIAN_POINT ( 'NONE',  ( 98.15313185440923860, 83.62500000136560629, 4.458734124999987891 ) ) ;
#17009=DIRECTION ( 'NONE',  ( -0.000000000000000000, 1.000000000000000000, -0.000000000000000000 ) ) ;
#17012=CARTESIAN_POINT ( 'NONE',  ( 8.193155644909767332, 36.00000000000001421, 10.45682415286414546 ) ) ;
#17013=CARTESIAN_POINT ( 'NONE',  ( 8.754898953241641024, 50.00000000000000000, 10.39041163855821637 ) ) ;
#17014=CARTESIAN_POINT ( 'NONE',  ( 116.4251840539369596, 32.31835937499999289, 5.622872871577880183 ) ) ;
#17020=CARTESIAN_POINT ( 'NONE',  ( 143.1451861577818079, 35.64218750108393152, -5.444914386472297529 ) ) ;
#17021=CARTESIAN_POINT ( 'NONE',  ( 65.00000000000000000, 36.78320312608393294, 13.14518615778179544 ) ) ;
#17022=EDGE_CURVE ( 'NONE', #21964, #24113, #26662, .T. ) ;
#17023=CARTESIAN_POINT ( 'NONE',  ( 181.8548138422181921, 32.66562500108393863, 5.444914386472304635 ) ) ;
#17024=CARTESIAN_POINT ( 'NONE',  ( 55.28645250595090488, 35.99999999999999289, 8.898183052316495534 ) ) ;
#17025=CARTESIAN_POINT ( 'NONE',  ( -9.295050272127046043, 34.89804687608393152, -9.295050272127046043 ) ) ;
#17027=CARTESIAN_POINT ( 'NONE',  ( 123.5871333237427905, 50.00000000108524034, -11.99502265407588730 ) ) ;
#17030=CARTESIAN_POINT ( 'NONE',  ( -13.14518615778179544, 39.75976562608393294, 0.000000000000000000 ) ) ;
#17039=ORIENTED_EDGE ( 'NONE', *, *, #10185, .F. ) ;
#17044=CARTESIAN_POINT ( 'NONE',  ( 0.000000000000000000, -7.395377635281828788, 0.000000000000000000 ) ) ;
#17045=CARTESIAN_POINT ( 'NONE',  ( 95.54126587499996504, 79.43750000136559208, -1.387778780781445676E-14 ) ) ;
#17046=CARTESIAN_POINT ( 'NONE',  ( 51.85481384221820633, 40.00781250108393294, 5.444914386472304635 ) ) ;
#17048=CARTESIAN_POINT ( 'NONE',  ( 65.00000000000000000, -7.395377635281828788, -7.517135062566165128E-15 ) ) ;
#17050=LINE ( 'NONE', #1693, #4963 ) ;
#17052=CARTESIAN_POINT ( 'NONE',  ( 139.5988444088204403, 40.70234374999999716, -9.598844408820458085 ) ) ;
#17057=CARTESIAN_POINT ( 'NONE',  ( 143.1451861577818079, 39.36289062608393152, -1.609821015232357215E-15 ) ) ;
#17058=CARTESIAN_POINT ( 'NONE',  ( 59.37712712842213136, 36.98164062716787015, -13.57481594606304753 ) ) ;
#17061=CARTESIAN_POINT ( 'NONE',  ( 13.57481594606304931, 34.30273437716787299, 5.622872871577869525 ) ) ;
#17065=CARTESIAN_POINT ( 'NONE',  ( 195.0000000000000000, 38.37070312608393152, 13.14518615778179544 ) ) ;
#17068=CARTESIAN_POINT ( 'NONE',  ( 135.4449143864723339, 37.92421875108393436, -13.14518615778179722 ) ) ;
#17069=CARTESIAN_POINT ( 'NONE',  ( 55.81982418635200816, 55.00000000000000000, 9.999999999999984013 ) ) ;
#17074=CARTESIAN_POINT ( 'NONE',  ( 200.6228728715778686, 38.86679687499999858, 13.57481594606304576 ) ) ;
#17075=CARTESIAN_POINT ( 'NONE',  ( 59.37712712842218110, 39.26367187500000000, -13.57481594606310260 ) ) ;
#17077=CARTESIAN_POINT ( 'NONE',  ( 59.55508561352770158, 38.81718750108393579, -13.14518615778179900 ) ) ;
#17079=( BOUNDED_CURVE ( )  B_SPLINE_CURVE ( 2, ( #12172, #14460, #16471, #23177, #14318, #12036, #27458, #3510, #25830 ),
 .UNSPECIFIED., .F., .F. ) 
 B_SPLINE_CURVE_WITH_KNOTS ( ( 3, 2, 2, 2, 3 ),
 ( 0.4375000000000003331, 0.4479166666666669627, 0.4583333333333335369, 0.4687500000000001665, 0.4791666666666667962 ),
 .UNSPECIFIED. ) 
 CURVE ( )  GEOMETRIC_REPRESENTATION_ITEM ( )  RATIONAL_B_SPLINE_CURVE ( ( 0.9999999999999975575, 0.9238795325112891810, 1.000000000000000000, 0.9238795325112867385, 1.000000000000000000, 0.9238795325112867385, 1.000000000000000000, 0.9238795325112859613, 1.000000000000000888 ) ) 
 REPRESENTATION_ITEM ( '' )  );
#17080=AXIS2_PLACEMENT_3D ( 'NONE', #1371, #27861, #25710 ) ;
#17085=CARTESIAN_POINT ( 'NONE',  ( -5.622872871577873077, 38.46992187499999716, -13.57481594606304753 ) ) ;
#17086=CARTESIAN_POINT ( 'NONE',  ( 130.0000000000000000, 39.75976562608394005, -13.14518615778179544 ) ) ;
#17088=CARTESIAN_POINT ( 'NONE',  ( 95.54126587499995082, 81.62500000136560629, -1.846868145590750077 ) ) ;
#17089=AXIS2_PLACEMENT_3D ( 'NONE', #15396, #23827, #4307 ) ;
#17091=ORIENTED_EDGE ( 'NONE', *, *, #12266, .F. ) ;
#17093=CARTESIAN_POINT ( 'NONE',  ( 55.70494972787295751, 33.50898437608393010, -9.295050272127046043 ) ) ;
#17097=VERTEX_POINT ( 'NONE', #9294 ) ;
#17100=CARTESIAN_POINT ( 'NONE',  ( 200.6228728715778686, 38.46992187716787015, -13.57481594606304753 ) ) ;
#17103=CARTESIAN_POINT ( 'NONE',  ( 203.7693896720689963, 50.37710889401661518, 14.99999999999732836 ) ) ;
#17104=CARTESIAN_POINT ( 'NONE',  ( 143.1451861577818363, 38.81718750108393579, -5.444914386472297529 ) ) ;
#17105=CARTESIAN_POINT ( 'NONE',  ( 2.414731522848535132E-15, 37.77539062608393294, 13.14518615778179544 ) ) ;
#17107=CARTESIAN_POINT ( 'NONE',  ( 143.1451861577818079, 33.75703125108393010, 5.444914386472293977 ) ) ;
#17108=CARTESIAN_POINT ( 'NONE',  ( 51.42518405393695957, 37.87460937499999147, 5.622872871577880183 ) ) ;
#17109=AXIS2_PLACEMENT_3D ( 'NONE', #25899, #2389, #13462 ) ;
#17110=CARTESIAN_POINT ( 'NONE',  ( 13.57481594606304931, 38.27148437716787299, 5.622872871577868636 ) ) ;
#17116=( BOUNDED_CURVE ( )  B_SPLINE_CURVE ( 2, ( #1086, #7471, #3633, #9892, #27577 ),
 .UNSPECIFIED., .F., .F. ) 
 B_SPLINE_CURVE_WITH_KNOTS ( ( 3, 2, 3 ),
 ( 0.000000000000000000, 0.01041666666666679446, 0.02083333333333358892 ),
 .UNSPECIFIED. ) 
 CURVE ( )  GEOMETRIC_REPRESENTATION_ITEM ( )  RATIONAL_B_SPLINE_CURVE ( ( 1.000000000000000000, 0.9238795325112867385, 1.000000000000000000, 0.9238795325112848511, 1.000000000000001776 ) ) 
 REPRESENTATION_ITEM ( '' )  );
#17119=CARTESIAN_POINT ( 'NONE',  ( -9.295050272127046043, 38.27148437608393294, -9.295050272127046043 ) ) ;
#17127=CARTESIAN_POINT ( 'NONE',  ( -9.598844408820454532, 40.30546874999999574, 9.598844408820459861 ) ) ;
#17129=CARTESIAN_POINT ( 'NONE',  ( 185.7049497278729575, 39.85898437608393152, 9.295050272127047819 ) ) ;
#17131=ORIENTED_EDGE ( 'NONE', *, *, #2461, .F. ) ;
#17134=AXIS2_PLACEMENT_3D ( 'NONE', #12828, #173, #17546 ) ;
#17136=ORIENTED_EDGE ( 'NONE', *, *, #11224, .T. ) ;
#17140=CARTESIAN_POINT ( 'NONE',  ( 124.3771271284221314, 34.89804687716787868, 13.57481594606304753 ) ) ;
#17141=VECTOR ( 'NONE', #25097, 1000.000000000000000 ) ;
#17142=CARTESIAN_POINT ( 'NONE',  ( 99.99999999999995737, 81.37500000273119838, 4.999999999999990230 ) ) ;
#17144=CARTESIAN_POINT ( 'NONE',  ( 185.7049497278729575, 35.09648437608393579, -9.295050272127046043 ) ) ;
#17146=ORIENTED_EDGE ( 'NONE', *, *, #22375, .F. ) ;
#17149=DIRECTION ( 'NONE',  ( -0.8660254037844407060, 0.4999999999999963363, 0.000000000000000000 ) ) ;
#17150=EDGE_CURVE ( 'NONE', #21981, #15490, #620, .T. ) ;
#17153=CARTESIAN_POINT ( 'NONE',  ( 96.84719886470459471, 81.31250000136559208, -3.152801135295383084 ) ) ;
#17154=CARTESIAN_POINT ( 'NONE',  ( 181.8548138422182205, 38.91640625108393436, -5.444914386472297529 ) ) ;
#17158=CARTESIAN_POINT ( 'NONE',  ( 204.2950502721270425, 39.66054687608393436, -9.295050272127046043 ) ) ;
#17160=EDGE_CURVE ( 'NONE', #12494, #2842, #24085, .T. ) ;
#17167=CARTESIAN_POINT ( 'NONE',  ( 130.0000000000000000, 35.39414062608393863, 13.14518615778179544 ) ) ;
#17168=AXIS2_PLACEMENT_3D ( 'NONE', #25014, #1083, #23296 ) ;
#17169=CARTESIAN_POINT ( 'NONE',  ( 59.55508561352770158, 38.02343750108394005, -13.14518615778179900 ) ) ;
#17170=EDGE_CURVE ( 'NONE', #4508, #17588, #9689, .T. ) ;
#17171=CARTESIAN_POINT ( 'NONE',  ( 181.8548138422181921, 39.21406250108392300, 5.444914386472304635 ) ) ;
#17172=DIRECTION ( 'NONE',  ( 0.000000000000000000, 1.000000000000000000, 0.000000000000000000 ) ) ;
#17173=CARTESIAN_POINT ( 'NONE',  ( -5.444914386472299306, 34.35234375108392868, 13.14518615778179722 ) ) ;
#17174=CARTESIAN_POINT ( 'NONE',  ( 123.9140557840132573, 54.65299103241509471, -15.00000000000000000 ) ) ;
#17175=CARTESIAN_POINT ( 'NONE',  ( 124.3771271284221172, 40.35507812499999147, 13.57481594606302444 ) ) ;
#17176=CARTESIAN_POINT ( 'NONE',  ( 2.414731522848535132E-15, 39.16445312608392726, 13.14518615778179544 ) ) ;
#17178=CYLINDRICAL_SURFACE ( 'NONE', #5971, 5.000000000000004441 ) ;
#17185=CARTESIAN_POINT ( 'NONE',  ( 130.4460412567749188, 49.99999999978043519, 13.57776691409199898 ) ) ;
#17188=CARTESIAN_POINT ( 'NONE',  ( 99.99999999999995737, 79.93750000136559208, 4.458734124999988779 ) ) ;
#17189=CARTESIAN_POINT ( 'NONE',  ( 59.55508561352770158, 37.42812500108394147, -13.14518615778179900 ) ) ;
#17191=CARTESIAN_POINT ( 'NONE',  ( -13.14518615778179722, 39.71015625108393010, -5.444914386472297529 ) ) ;
#17192=PLANE ( 'NONE',  #2570 ) ;
#17195=CARTESIAN_POINT ( 'NONE',  ( 124.3771271284221314, 40.35507812499998437, 13.57481594606304753 ) ) ;
#17196=EDGE_CURVE ( 'NONE', #11161, #22131, #27019, .T. ) ;
#17197=ORIENTED_EDGE ( 'NONE', *, *, #10510, .F. ) ;
#17202=CARTESIAN_POINT ( 'NONE',  ( 135.4449143864723055, 36.03906250108394005, 13.14518615778179189 ) ) ;
#17203=CARTESIAN_POINT ( 'NONE',  ( 51.42518405393695957, 36.28710937716787299, -5.622872871577873077 ) ) ;
#17205=CARTESIAN_POINT ( 'NONE',  ( -9.598844408820458085, 37.03125000216787299, -9.598844408820458085 ) ) ;
#17209=CARTESIAN_POINT ( 'NONE',  ( 185.4011555911795597, 33.16171874999999858, 9.598844408820459861 ) ) ;
#17210=CARTESIAN_POINT ( 'NONE',  ( 204.2950502721270425, 38.66835937608393436, -9.295050272127046043 ) ) ;
#17211=CARTESIAN_POINT ( 'NONE',  ( 65.00000000000000000, 38.42031249999999432, -13.57481594606304576 ) ) ;
#17215=CARTESIAN_POINT ( 'NONE',  ( 126.1345856245867907, 54.10683252460150072, 14.99999999999996980 ) ) ;
#17216=CARTESIAN_POINT ( 'NONE',  ( 51.42518405393695957, 37.08085937499999574, 5.622872871577880183 ) ) ;
#17219=CARTESIAN_POINT ( 'NONE',  ( 181.4251840539369596, 37.77539062499999289, -5.622872871577873077 ) ) ;
#17220=CARTESIAN_POINT ( 'NONE',  ( 65.00000000000000000, -7.395377635281828788, -13.57481594606305109 ) ) ;
#17222=CARTESIAN_POINT ( 'NONE',  ( 70.44491438647230552, 37.92421875108392726, -13.14518615778179900 ) ) ;
#17227=CARTESIAN_POINT ( 'NONE',  ( 5.622872871577871301, 39.16445312499999432, -13.57481594606304753 ) ) ;
#17228=CARTESIAN_POINT ( 'NONE',  ( 124.5550856135277087, 39.31328125108394289, 13.14518615778179722 ) ) ;
#17229=AXIS2_PLACEMENT_3D ( 'NONE', #5789, #8050, #20897 ) ;
#17231=VERTEX_POINT ( 'NONE', #17534 ) ;
#17232=CARTESIAN_POINT ( 'NONE',  ( 97.92893218813451028, 83.18750000000001421, 4.999999999999989342 ) ) ;
#17233=AXIS2_PLACEMENT_3D ( 'NONE', #13300, #19599, #20173 ) ;
#17237=CARTESIAN_POINT ( 'NONE',  ( 74.29505027212704249, 33.31054687608394005, -9.295050272127046043 ) ) ;
#17242=EDGE_LOOP ( 'NONE', ( #18606, #11476, #59, #22591 ) ) ;
#17245=UNCERTAINTY_MEASURE_WITH_UNIT (LENGTH_MEASURE( 1.000000000000000082E-05 ), #16604, 'distance_accuracy_value', 'NONE');
#17246=EDGE_CURVE ( 'NONE', #3560, #4816, #21967, .T. ) ;
#17247=CARTESIAN_POINT ( 'NONE',  ( 208.5748159460630688, 39.11484375216787157, -1.662435489736055892E-15 ) ) ;
#17250=CARTESIAN_POINT ( 'NONE',  ( 196.8921833570923923, 53.66387243068088964, 14.99999999999994671 ) ) ;
#17251=CARTESIAN_POINT ( 'NONE',  ( 116.8548138422182205, 38.42031250108393436, 5.444914386472304635 ) ) ;
#17252=CARTESIAN_POINT ( 'NONE',  ( 13.14518615778179900, 37.22968750108393721, -5.444914386472297529 ) ) ;
#17254=CARTESIAN_POINT ( 'NONE',  ( 135.4449143864723055, 35.54296875108393294, -13.14518615778179900 ) ) ;
#17255=CARTESIAN_POINT ( 'NONE',  ( 70.62287287157786864, 38.37070312499999147, -13.57481594606304753 ) ) ;
#17257=AXIS2_PLACEMENT_3D ( 'NONE', #6850, #10696, #4584 ) ;
#17259=CARTESIAN_POINT ( 'NONE',  ( 196.1371678245420753, 35.99999999999999289, 13.09590655363592582 ) ) ;
#17262=CARTESIAN_POINT ( 'NONE',  ( 9.598844408820459861, 39.01562500216787299, 9.598844408820456309 ) ) ;
#17263=DIRECTION ( 'NONE',  ( 0.000000000000000000, 1.000000000000000000, 0.000000000000000000 ) ) ;
#17265=CARTESIAN_POINT ( 'NONE',  ( 5.444914386472297529, 38.91640625108393436, -13.14518615778179900 ) ) ;
#17269=CARTESIAN_POINT ( 'NONE',  ( 99.99999999999995737, 79.87500000273119838, -5.000000000000018652 ) ) ;
#17271=CARTESIAN_POINT ( 'NONE',  ( 195.0000000000000000, 39.16445312608392726, 13.14518615778179544 ) ) ;
#17274=VECTOR ( 'NONE', #1182, 1000.000000000000000 ) ;
#17276=CARTESIAN_POINT ( 'NONE',  ( 139.5988444088204687, 39.71015624999999716, 9.598844408820456309 ) ) ;
#17277=ORIENTED_EDGE ( 'NONE', *, *, #11512, .T. ) ;
#17282=CARTESIAN_POINT ( 'NONE',  ( 135.4449143864723055, 40.30546875108393579, -13.14518615778179900 ) ) ;
#17285=CARTESIAN_POINT ( 'NONE',  ( 78.14518615778179367, 39.56132812608393579, -1.609821015232357215E-15 ) ) ;
#17287=CARTESIAN_POINT ( 'NONE',  ( 208.1451861577817795, 34.84843750108393579, -5.444914386472297529 ) ) ;
#17288=ORIENTED_EDGE ( 'NONE', *, *, #21750, .T. ) ;
#17292=CARTESIAN_POINT ( 'NONE',  ( 51.85481384221820633, 39.75976562608393294, 0.000000000000000000 ) ) ;
#17293=CARTESIAN_POINT ( 'NONE',  ( 103.1528011352953342, 80.81250000136559208, 3.152801135295355106 ) ) ;
#17294=CARTESIAN_POINT ( 'NONE',  ( 200.4449143864723055, 38.71796875108393721, -13.14518615778179722 ) ) ;
#17301=EDGE_CURVE ( 'NONE', #21288, #12843, #2071, .T. ) ;
#17306=CARTESIAN_POINT ( 'NONE',  ( 124.5550856135277087, 36.13828125108393863, 13.14518615778179722 ) ) ;
#17307=CARTESIAN_POINT ( 'NONE',  ( 65.00000000000000000, 32.41757812608393863, -13.14518615778179544 ) ) ;
#17308=CARTESIAN_POINT ( 'NONE',  ( 195.0000000000000000, 38.17226562608394147, -13.14518615778179544 ) ) ;
#17311=CARTESIAN_POINT ( 'NONE',  ( -13.14518615778179544, 31.82226562608393650, 0.000000000000000000 ) ) ;
#17312=CARTESIAN_POINT ( 'NONE',  ( 138.4023157812348472, 54.99999999485618929, -15.00000000000000000 ) ) ;
#17313=EDGE_CURVE ( 'NONE', #10602, #8880, #27919, .T. ) ;
#17314=CARTESIAN_POINT ( 'NONE',  ( 190.2199608011490852, 35.99999999999998579, 12.25280873422859784 ) ) ;
#17318=EDGE_CURVE ( 'NONE', #27401, #2214, #3000, .T. ) ;
#17319=CARTESIAN_POINT ( 'NONE',  ( -13.14518615778179544, 35.79101562608393294, 0.000000000000000000 ) ) ;
#17320=CARTESIAN_POINT ( 'NONE',  ( -18.00000000000000355, 80.00000000000000000, 13.00000000000000178 ) ) ;
#17323=CARTESIAN_POINT ( 'NONE',  ( 55.81982418635200105, 50.00000000000001421, 14.99999999999998934 ) ) ;
#17333=LINE ( 'NONE', #19897, #8566 ) ;
#17334=CARTESIAN_POINT ( 'NONE',  ( 96.84719886470459471, 81.81250000136559208, 3.152801135295355994 ) ) ;
#17335=CARTESIAN_POINT ( 'NONE',  ( 74.29505027212704249, 34.89804687608393863, -9.295050272127046043 ) ) ;
#17336=( BOUNDED_SURFACE ( )  B_SPLINE_SURFACE ( 3, 2, ( 
 ( #4511, #15606, #6496 ),
 ( #22039, #4370, #13168 ),
 ( #4228, #24309, #12887 ),
 ( #17607, #21617, #26314 ),
 ( #15172, #2093, #2515 ),
 ( #10761, #8919, #28171 ),
 ( #23891, #11177, #15461 ),
 ( #19895, #4795, #13026 ),
 ( #15318, #13454, #21907 ),
 ( #17185, #21763, #2240 ),
 ( #2381, #24032, #11039 ),
 ( #19749, #232, #6775 ),
 ( #24176, #1095, #22890 ),
 ( #5080, #5221, #24740 ),
 ( #11601, #13602, #13886 ),
 ( #9762, #24884, #2931 ),
 ( #15749, #13742, #3355 ),
 ( #11463, #811, #26604 ),
 ( #20042, #7050, #666 ),
 ( #521, #22325, #5363 ) ),
 .UNSPECIFIED., .F., .F., .F. ) 
 B_SPLINE_SURFACE_WITH_KNOTS ( ( 4, 2, 2, 2, 2, 2, 2, 2, 2, 4 ),
 ( 3, 3 ),
 ( 0.009073803551359473779, 0.01139250602759182829, 0.01371120850382418453, 0.01602991098005654078, 0.01834861345628889528, 0.01950796469440507080, 0.02066731593252124979, 0.02298601840875360430, 0.02530472088498595881, 0.02762342336121831332 ),
 ( 0.000000000000000000, 1.000000000000000000 ),
 .UNSPECIFIED. ) 
 GEOMETRIC_REPRESENTATION_ITEM ( )  RATIONAL_B_SPLINE_SURFACE ( (
 ( 1.000000000000000000, 0.7071067811865476838, 1.000000000000000000),
 ( 1.000000000000000000, 0.7344871497827925033, 1.000000000000000000),
 ( 1.000000000000000000, 0.7612510203320145274, 1.000000000000000000),
 ( 1.000000000000000000, 0.8116663633842718939, 1.000000000000000000),
 ( 1.000000000000000000, 0.8353358059749915743, 1.000000000000000000),
 ( 1.000000000000000000, 0.8764699612587960598, 1.000000000000000000),
 ( 1.000000000000000000, 0.8939017358719169026, 1.000000000000000000),
 ( 1.000000000000000000, 0.9185314935647126422, 1.000000000000000000),
 ( 1.000000000000000000, 0.9256439951240776898, 1.000000000000000000),
 ( 1.000000000000000000, 0.9261623622475867457, 1.000000000000000000),
 ( 1.000000000000000000, 0.9246301385979069920, 1.000000000000000000),
 ( 1.000000000000000000, 0.9183304321347807164, 1.000000000000000000),
 ( 1.000000000000000000, 0.9135987334167550156, 1.000000000000000000),
 ( 1.000000000000000000, 0.8954110486041423345, 1.000000000000000000),
 ( 1.000000000000000000, 0.8779877431162668167, 1.000000000000000000),
 ( 1.000000000000000000, 0.8366182664710850592, 1.000000000000000000),
 ( 1.000000000000000000, 0.8126941604011834741, 1.000000000000000000),
 ( 1.000000000000000000, 0.7617527316309427032, 1.000000000000000000),
 ( 1.000000000000000000, 0.7347103785789421693, 1.000000000000000000),
 ( 1.000000000000000000, 0.7071067811865464625, 1.000000000000000000) ) ) 
 REPRESENTATION_ITEM ( '' )  SURFACE ( )  );
#17338=CARTESIAN_POINT ( 'NONE',  ( 104.9999999999999716, 80.68750000273119838, -2.071067811865491937 ) ) ;
#17340=CARTESIAN_POINT ( 'NONE',  ( 143.5748159460630688, 39.01562500000000000, -1.662435489736055892E-15 ) ) ;
#17346=CARTESIAN_POINT ( 'NONE',  ( 124.5550856135277087, 36.43593750108392726, -13.14518615778179900 ) ) ;
#17347=CARTESIAN_POINT ( 'NONE',  ( 70.62287287157788285, 32.61601562716786873, 13.57481594606304576 ) ) ;
#17350=CARTESIAN_POINT ( 'NONE',  ( 13.57481594606304931, 35.89023437716787868, 5.622872871577869525 ) ) ;
#17352=CARTESIAN_POINT ( 'NONE',  ( -20.00000000000000355, 55.00000000000000000, -14.99999999999999822 ) ) ;
#17354=CARTESIAN_POINT ( 'NONE',  ( 204.2950502721270425, 37.08085937608393579, -9.295050272127046043 ) ) ;
#17355=CARTESIAN_POINT ( 'NONE',  ( 70.62287287157791127, 38.86679687500001279, 13.57481594606301023 ) ) ;
#17358=CARTESIAN_POINT ( 'NONE',  ( 195.0000000000000000, 38.12265625216787157, 13.57481594606304576 ) ) ;
#17360=CARTESIAN_POINT ( 'NONE',  ( 122.3760580380745324, 55.00000000000000711, 14.99999999999997158 ) ) ;
#17365=CARTESIAN_POINT ( 'NONE',  ( 181.4251840539369596, 33.06249999999999289, 0.000000000000000000 ) ) ;
#17368=CARTESIAN_POINT ( 'NONE',  ( 59.55508561352770158, 34.35234375108392868, 13.14518615778179722 ) ) ;
#17373=CARTESIAN_POINT ( 'NONE',  ( 9.598844408820459861, 35.74140624999999716, 9.598844408820456309 ) ) ;
#17374=DIRECTION ( 'NONE',  ( -2.385244779468110248E-16, 0.000000000000000000, -1.000000000000000000 ) ) ;
#17375=ORIENTED_EDGE ( 'NONE', *, *, #5970, .T. ) ;
#17376=CARTESIAN_POINT ( 'NONE',  ( 102.0710678118654329, 83.31250000000000000, 4.999999999999989342 ) ) ;
#17379=ORIENTED_EDGE ( 'NONE', *, *, #23264, .F. ) ;
#17381=CARTESIAN_POINT ( 'NONE',  ( 78.14518615778179367, 34.79882812608394005, -1.609821015232357215E-15 ) ) ;
#17382=ORIENTED_EDGE ( 'NONE', *, *, #971, .T. ) ;
#17385=EDGE_CURVE ( 'NONE', #16078, #19393, #2759, .T. ) ;
#17387=DIRECTION ( 'NONE',  ( 0.000000000000000000, 0.000000000000000000, -1.000000000000000000 ) ) ;
#17389=CARTESIAN_POINT ( 'NONE',  ( 200.6228728715778686, 37.67617187716787441, -13.57481594606304753 ) ) ;
#17391=DIRECTION ( 'NONE',  ( -1.000000000000000000, -0.000000000000000000, 2.385244779468110248E-16 ) ) ;
#17392=CARTESIAN_POINT ( 'NONE',  ( 203.2596115289017291, 50.00000000056336091, 10.79618466885029093 ) ) ;
#17394=CARTESIAN_POINT ( 'NONE',  ( 116.9040934463640156, 35.99999999999999289, 1.137167824541468031 ) ) ;
#17396=CARTESIAN_POINT ( 'NONE',  ( -13.14518615778179900, 39.11484375108394573, -5.444914386472297529 ) ) ;
#17397=CARTESIAN_POINT ( 'NONE',  ( 130.0000000000000000, 35.98945312608393010, 13.14518615778179544 ) ) ;
#17398=CARTESIAN_POINT ( 'NONE',  ( 51.42518405393695957, 33.85624999999999574, 0.000000000000000000 ) ) ;
#17403=LINE ( 'NONE', #12962, #19997 ) ;
#17406=CARTESIAN_POINT ( 'NONE',  ( -13.14518615778179189, 36.03906250108394005, 5.444914386472304635 ) ) ;
#17407=AXIS2_PLACEMENT_3D ( 'NONE', #14519, #23234, #8385 ) ;
#17409=ORIENTED_EDGE ( 'NONE', *, *, #246, .F. ) ;
#17412=CARTESIAN_POINT ( 'NONE',  ( 130.0000000000000000, 36.93203125216787441, -13.57481594606304576 ) ) ;
#17414=CARTESIAN_POINT ( 'NONE',  ( 200.4449143864723055, 40.00781250108393294, 13.14518615778179189 ) ) ;
#17416=CARTESIAN_POINT ( 'NONE',  ( 70.44491438647229131, 36.53515625108394715, -13.14518615778179722 ) ) ;
#17419=EDGE_LOOP ( 'NONE', ( #22812, #17908 ) ) ;
#17423=AXIS2_PLACEMENT_3D ( 'NONE', #14724, #25575, #7907 ) ;
#17424=CARTESIAN_POINT ( 'NONE',  ( 135.4449143864723055, 39.21406250108392300, 13.14518615778179189 ) ) ;
#17425=CARTESIAN_POINT ( 'NONE',  ( -13.14518615778179722, 40.70234375108392300, -5.444914386472297529 ) ) ;
#17427=CARTESIAN_POINT ( 'NONE',  ( 59.55508561352770158, 40.10703125108393152, 13.14518615778179722 ) ) ;
#17429=CARTESIAN_POINT ( 'NONE',  ( 181.8548138422182205, 35.19570312608393436, 0.000000000000000000 ) ) ;
#17435=CARTESIAN_POINT ( 'NONE',  ( 51.85481384221820633, 39.71015625108393010, -5.444914386472297529 ) ) ;
#17436=CARTESIAN_POINT ( 'NONE',  ( 95.54126587499996504, 82.43750000136559208, -1.387778780781445676E-14 ) ) ;
#17437=CARTESIAN_POINT ( 'NONE',  ( 181.8548138422182205, 39.71015625108393010, -5.444914386472297529 ) ) ;
#17443=ORIENTED_EDGE ( 'NONE', *, *, #23954, .T. ) ;
#17444=VECTOR ( 'NONE', #21225, 1000.000000000000000 ) ;
#17448=CARTESIAN_POINT ( 'NONE',  ( 116.8548138422182205, 36.78320312608393294, 0.000000000000000000 ) ) ;
#17449=CARTESIAN_POINT ( 'NONE',  ( 78.14518615778179367, 34.55078125108393294, 5.444914386472293977 ) ) ;
#17450=CARTESIAN_POINT ( 'NONE',  ( 185.7049497278729575, 36.08867187608393579, 9.295050272127047819 ) ) ;
#17452=( BOUNDED_CURVE ( )  B_SPLINE_CURVE ( 2, ( #12783, #6389, #1980, #10649, #4253, #13052, #8664, #17355, #21788 ),
 .UNSPECIFIED., .F., .F. ) 
 B_SPLINE_CURVE_WITH_KNOTS ( ( 3, 2, 2, 2, 3 ),
 ( 0.1875000000000001388, 0.1979166666666667407, 0.2083333333333333703, 0.2187499999999999722, 0.2291666666666665741 ),
 .UNSPECIFIED. ) 
 CURVE ( )  GEOMETRIC_REPRESENTATION_ITEM ( )  RATIONAL_B_SPLINE_CURVE ( ( 0.9999999999999990008, 0.9238795325112877377, 1.000000000000000000, 0.9238795325112867385, 1.000000000000000000, 0.9238795325112867385, 1.000000000000000000, 0.9238795325112872936, 0.9999999999999994449 ) ) 
 REPRESENTATION_ITEM ( '' )  );
#17454=CARTESIAN_POINT ( 'NONE',  ( 116.4251840539369454, 40.25585937716787299, -5.622872871577873077 ) ) ;
#17456=CARTESIAN_POINT ( 'NONE',  ( 5.444914386472302859, 36.03906250108394005, 13.14518615778179189 ) ) ;
#17460=ORIENTED_EDGE ( 'NONE', *, *, #17313, .T. ) ;
#17467=FACE_OUTER_BOUND ( 'NONE', #635, .T. ) ;
#17468=CARTESIAN_POINT ( 'NONE',  ( 101.8468681455906903, 82.00000000136560629, 4.458734124999987891 ) ) ;
#17469=CARTESIAN_POINT ( 'NONE',  ( 78.14518615778179367, 34.00507812608393721, -1.609821015232357215E-15 ) ) ;
#17471=CARTESIAN_POINT ( 'NONE',  ( 9.295050272127046043, 38.66835937608393436, -9.295050272127046043 ) ) ;
#17472=EDGE_CURVE ( 'NONE', #12585, #17231, #15148, .T. ) ;
#17473=DIRECTION ( 'NONE',  ( 0.000000000000000000, -1.000000000000000000, 0.000000000000000000 ) ) ;
#17474=DIRECTION ( 'NONE',  ( -0.000000000000000000, -1.000000000000000000, -0.000000000000000000 ) ) ;
#17476=CARTESIAN_POINT ( 'NONE',  ( 124.3771271284221314, 38.46992187499999716, -13.57481594606304753 ) ) ;
#17478=ORIENTED_EDGE ( 'NONE', *, *, #15375, .T. ) ;
#17483=CARTESIAN_POINT ( 'NONE',  ( 120.7049497278729575, 36.68398437608392726, 9.295050272127047819 ) ) ;
#17484=CARTESIAN_POINT ( 'NONE',  ( 78.57481594606305464, 33.55859375216787299, -1.662435489736055892E-15 ) ) ;
#17487=CARTESIAN_POINT ( 'NONE',  ( 9.598844408820456309, 32.86406250216787583, -9.598844408820458085 ) ) ;
#17489=EDGE_CURVE ( 'NONE', #22555, #16261, #18089, .T. ) ;
#17492=CARTESIAN_POINT ( 'NONE',  ( 200.4449143864723055, 33.65781250108393152, 13.14518615778179189 ) ) ;
#17495=ORIENTED_EDGE ( 'NONE', *, *, #16104, .F. ) ;
#17497=CARTESIAN_POINT ( 'NONE',  ( 94.99999999999995737, 84.12500000273119838, -1.387778780781445676E-14 ) ) ;
#17498=DIRECTION ( 'NONE',  ( 0.000000000000000000, 0.000000000000000000, -1.000000000000000000 ) ) ;
#17500=CARTESIAN_POINT ( 'NONE',  ( 143.5748159460630688, 38.22187499999999716, -1.662435489736055892E-15 ) ) ;
#17503=CARTESIAN_POINT ( 'NONE',  ( 208.5748159460630120, 34.99726562500000426, 5.622872871577869525 ) ) ;
#17506=CARTESIAN_POINT ( 'NONE',  ( 74.29505027212704249, 35.29492187608393294, 9.295050272127046043 ) ) ;
#17511=LINE ( 'NONE', #17652, #20280 ) ;
#17512=CARTESIAN_POINT ( 'NONE',  ( -5.622872871577873077, 35.29492187500000000, -13.57481594606304753 ) ) ;
#17513=CARTESIAN_POINT ( 'NONE',  ( 139.2950502721270425, 36.48554687608393721, -9.295050272127046043 ) ) ;
#17514=ORIENTED_EDGE ( 'NONE', *, *, #6175, .T. ) ;
#17515=CARTESIAN_POINT ( 'NONE',  ( 96.84719886470459471, 79.81250000136559208, 3.152801135295355994 ) ) ;
#17516=AXIS2_PLACEMENT_3D ( 'NONE', #17778, #26481, #4389 ) ;
#17517=CARTESIAN_POINT ( 'NONE',  ( 97.92893218813451028, 81.93750000273118417, -5.000000000000018652 ) ) ;
#17519=CARTESIAN_POINT ( 'NONE',  ( 61.57977918782911786, 35.99999999999998579, -13.02105590829194348 ) ) ;
#17522=CARTESIAN_POINT ( 'NONE',  ( 65.00000000000000000, 35.39414062608393863, 13.14518615778179544 ) ) ;
#17531=CARTESIAN_POINT ( 'NONE',  ( 208.5748159460630120, 34.40195312716787157, -5.622872871577873077 ) ) ;
#17534=CARTESIAN_POINT ( 'NONE',  ( 131.1371678245417627, 36.00000000000000000, 13.09590655363595602 ) ) ;
#17535=CARTESIAN_POINT ( 'NONE',  ( 5.444914386472302859, 37.82500000108392868, 13.14518615778179189 ) ) ;
#17536=CARTESIAN_POINT ( 'NONE',  ( 124.5550856135277087, 34.84843750108393579, -13.14518615778179900 ) ) ;
#17537=CARTESIAN_POINT ( 'NONE',  ( 78.57481594606304043, 35.09648437499998863, -5.622872871577873077 ) ) ;
#17540=CARTESIAN_POINT ( 'NONE',  ( 208.0420085811496733, 36.00000000000001421, -3.640726557254588158 ) ) ;
#17543=DIRECTION ( 'NONE',  ( 0.000000000000000000, 0.000000000000000000, 1.000000000000000000 ) ) ;
#17545=AXIS2_PLACEMENT_3D ( 'NONE', #23483, #25342, #6097 ) ;
#17546=DIRECTION ( 'NONE',  ( 0.000000000000000000, 0.000000000000000000, -1.000000000000000000 ) ) ;
#17548=CARTESIAN_POINT ( 'NONE',  ( 9.295050272127047819, 35.49335937608393721, 9.295050272127046043 ) ) ;
#17553=DIRECTION ( 'NONE',  ( -0.000000000000000000, 1.000000000000000000, -0.000000000000000000 ) ) ;
#17555=CARTESIAN_POINT ( 'NONE',  ( 189.5550856135277229, 40.40468750108393436, -13.14518615778179900 ) ) ;
#17556=EDGE_LOOP ( 'NONE', ( #24719, #13357, #25885, #27277, #7641, #4046 ) ) ;
#17557=CARTESIAN_POINT ( 'NONE',  ( 78.14518615778180788, 36.33671875108393579, 5.444914386472293977 ) ) ;
#17559=CARTESIAN_POINT ( 'NONE',  ( 65.84210759546466818, 53.50112910130383881, -15.00000000000000000 ) ) ;
#17564=CARTESIAN_POINT ( 'NONE',  ( 139.5988444088204403, 32.07031250216787299, -9.598844408820458085 ) ) ;
#17565=DIRECTION ( 'NONE',  ( 0.000000000000000000, 0.000000000000000000, 1.000000000000000000 ) ) ;
#17567=CARTESIAN_POINT ( 'NONE',  ( 59.55508561352770158, 36.93203125108394147, 13.14518615778179722 ) ) ;
#17568=CARTESIAN_POINT ( 'NONE',  ( 99.99999999999995737, 80.00000000000000000, -5.000000000000018652 ) ) ;
#17569=CARTESIAN_POINT ( 'NONE',  ( 200.4449143864723055, 35.44375000108393436, 13.14518615778179189 ) ) ;
#17575=AXIS2_PLACEMENT_3D ( 'NONE', #4014, #19115, #4155 ) ;
#17577=CARTESIAN_POINT ( 'NONE',  ( 104.4587341249999781, 79.87500000136560629, 1.846868145590721655 ) ) ;
#17578=CARTESIAN_POINT ( 'NONE',  ( 181.8548138422182205, 38.22187500108393721, 5.444914386472304635 ) ) ;
#17581=AXIS2_PLACEMENT_3D ( 'NONE', #16862, #10436, #18859 ) ;
#17583=CYLINDRICAL_SURFACE ( 'NONE', #6361, 13.57481594606304398 ) ;
#17588=VERTEX_POINT ( 'NONE', #26921 ) ;
#17589=CARTESIAN_POINT ( 'NONE',  ( 143.1451861577818079, 37.18007812608393436, -1.609821015232357215E-15 ) ) ;
#17590=CARTESIAN_POINT ( 'NONE',  ( 55.70494972787295751, 33.50898437608393010, 9.295050272127047819 ) ) ;
#17591=CARTESIAN_POINT ( 'NONE',  ( 208.1451861577817795, 36.33671875108394289, 5.444914386472293977 ) ) ;
#17594=CARTESIAN_POINT ( 'NONE',  ( 9.295050272127046043, 33.90585937608393152, -9.295050272127046043 ) ) ;
#17595=CARTESIAN_POINT ( 'NONE',  ( 131.1387681171055419, 50.00000000043814907, -13.56816686242498271 ) ) ;
#17596=CARTESIAN_POINT ( 'NONE',  ( 13.57481594606304576, 39.01562500000000000, -1.662435489736055892E-15 ) ) ;
#17597=CARTESIAN_POINT ( 'NONE',  ( 124.3771271284221314, 40.15664062716787441, -13.57481594606304753 ) ) ;
#17607=CARTESIAN_POINT ( 'NONE',  ( 122.8845096081448816, 49.99999999945637796, 11.58166858713987324 ) ) ;
#17610=CARTESIAN_POINT ( 'NONE',  ( 103.1528011352953342, 82.06250000136559208, 3.152801135295355106 ) ) ;
#17611=CARTESIAN_POINT ( 'NONE',  ( 70.44491438647230552, 34.65000000108393863, 13.14518615778179189 ) ) ;
#17613=CARTESIAN_POINT ( 'NONE',  ( 13.14518615778179722, 39.31328125108392868, 5.444914386472293977 ) ) ;
#17614=AXIS2_PLACEMENT_3D ( 'NONE', #27780, #12639, #15057 ) ;
#17616=CYLINDRICAL_SURFACE ( 'NONE', #13577, 13.57481594606304398 ) ;
#17617=CARTESIAN_POINT ( 'NONE',  ( 130.0000000000000000, 40.80156249999999574, -13.57481594606304576 ) ) ;
#17618=CARTESIAN_POINT ( 'NONE',  ( 120.4011555911795455, 36.33671874999999574, 9.598844408820459861 ) ) ;
#17620=ORIENTED_EDGE ( 'NONE', *, *, #14982, .T. ) ;
#17625=CARTESIAN_POINT ( 'NONE',  ( 139.2950502721270425, 37.08085937608393579, -9.295050272127046043 ) ) ;
#17626=CARTESIAN_POINT ( 'NONE',  ( 55.40115559117954547, 34.65000000216787868, -9.598844408820458085 ) ) ;
#17628=CARTESIAN_POINT ( 'NONE',  ( -8.049105076161786076E-16, 40.35507812608393152, -13.14518615778179544 ) ) ;
#17631=CARTESIAN_POINT ( 'NONE',  ( 185.7049497278729575, 34.89804687608393152, -9.295050272127046043 ) ) ;
#17632=VECTOR ( 'NONE', #10547, 1000.000000000000227 ) ;
#17636=CARTESIAN_POINT ( 'NONE',  ( 185.4011555911795597, 40.30546874999999574, 9.598844408820459861 ) ) ;
#17639=LINE ( 'NONE', #25919, #9507 ) ;
#17640=CARTESIAN_POINT ( 'NONE',  ( 126.8834079195342355, 53.90895096933309105, 14.99999999999996803 ) ) ;
#17645=CARTESIAN_POINT ( 'NONE',  ( 181.4251840539369596, 34.60039062499999574, -5.622872871577873077 ) ) ;
#17647=CARTESIAN_POINT ( 'NONE',  ( 143.5748159460630688, 36.63437499999999858, -1.662435489736055892E-15 ) ) ;
#17648=CARTESIAN_POINT ( 'NONE',  ( 78.14518615778179367, 35.34453125108392868, 5.444914386472293977 ) ) ;
#17651=ORIENTED_EDGE ( 'NONE', *, *, #7090, .T. ) ;
#17652=CARTESIAN_POINT ( 'NONE',  ( 219.9999999999999716, 55.00000000000000000, 14.99999999999994316 ) ) ;
#17653=CARTESIAN_POINT ( 'NONE',  ( 13.57481594606304576, 35.84062499999999574, -1.662435489736055892E-15 ) ) ;
#17654=CARTESIAN_POINT ( 'NONE',  ( 120.7049497278729575, 37.67617187608393436, 9.295050272127047819 ) ) ;
#17655=VERTEX_POINT ( 'NONE', #16766 ) ;
#17656=ORIENTED_EDGE ( 'NONE', *, *, #22631, .F. ) ;
#17657=CARTESIAN_POINT ( 'NONE',  ( 97.92893218813451028, 84.81250000000001421, -5.000000000000018652 ) ) ;
#17658=CARTESIAN_POINT ( 'NONE',  ( 104.9999999999999574, 83.56250000273119838, 2.071067811865462627 ) ) ;
#17660=CARTESIAN_POINT ( 'NONE',  ( 58.52943630333427194, 36.00000000000001421, -11.78199955157067436 ) ) ;
#17662=ADVANCED_FACE ( 'NONE', ( #25467 ), #5945, .T. ) ;
#17664=CARTESIAN_POINT ( 'NONE',  ( 78.14518615778179367, 32.46718750108393436, -5.444914386472297529 ) ) ;
#17665=ORIENTED_EDGE ( 'NONE', *, *, #21004, .T. ) ;
#17670=( BOUNDED_CURVE ( )  B_SPLINE_CURVE ( 2, ( #24183, #8786, #6642, #24042, #19758, #4518, #13176, #21915, #11049 ),
 .UNSPECIFIED., .F., .F. ) 
 B_SPLINE_CURVE_WITH_KNOTS ( ( 3, 2, 2, 2, 3 ),
 ( 0.4791666666666667962, 0.4895833333333333703, 0.5000000000000000000, 0.5104166666666665186, 0.5208333333333332593 ),
 .UNSPECIFIED. ) 
 CURVE ( )  GEOMETRIC_REPRESENTATION_ITEM ( )  RATIONAL_B_SPLINE_CURVE ( ( 0.9999999999999992228, 0.9238795325112875156, 1.000000000000000000, 0.9238795325112867385, 1.000000000000000000, 0.9238795325112867385, 1.000000000000000000, 0.9238795325112875156, 0.9999999999999992228 ) ) 
 REPRESENTATION_ITEM ( '' )  );
#17672=CARTESIAN_POINT ( 'NONE',  ( 204.5988444088204403, 35.24531250216787726, -9.598844408820458085 ) ) ;
#17676=CARTESIAN_POINT ( 'NONE',  ( 204.5988444088204403, 36.03906250216787299, -9.598844408820458085 ) ) ;
#17677=DIRECTION ( 'NONE',  ( 0.000000000000000000, 0.000000000000000000, 1.000000000000000000 ) ) ;
#17678=VERTEX_POINT ( 'NONE', #21189 ) ;
#17679=CARTESIAN_POINT ( 'NONE',  ( -5.444914386472297529, 36.63437500108393152, -13.14518615778179900 ) ) ;
#17681=CARTESIAN_POINT ( 'NONE',  ( 124.5550856135277087, 34.35234375108392868, 13.14518615778179722 ) ) ;
#17682=CARTESIAN_POINT ( 'NONE',  ( 70.62287287157788285, 34.89804687499999147, 13.57481594606304576 ) ) ;
#17688=CYLINDRICAL_SURFACE ( 'NONE', #13033, 5.000000000000000000 ) ;
#17695=CARTESIAN_POINT ( 'NONE',  ( 13.14518615778179544, 37.18007812608393436, -1.609821015232357215E-15 ) ) ;
#17702=CARTESIAN_POINT ( 'NONE',  ( 208.1451861577818079, 37.77539062608393294, -1.609821015232357215E-15 ) ) ;
#17703=ORIENTED_EDGE ( 'NONE', *, *, #8444, .F. ) ;
#17704=CARTESIAN_POINT ( 'NONE',  ( 141.1048480505471332, 36.02027164848243501, -8.092840767093784748 ) ) ;
#17705=CARTESIAN_POINT ( 'NONE',  ( 204.1801758136479918, 55.00000000000000000, -15.00000000000000000 ) ) ;
#17707=EDGE_LOOP ( 'NONE', ( #10109, #5737, #25276, #15600, #16272, #20292, #14618, #13975, #19072, #22405, #27045, #13972, #2176, #26889, #6737, #5004, #13272 ) ) ;
#17713=CARTESIAN_POINT ( 'NONE',  ( 143.5748159460630404, 32.71523437716787441, 5.622872871577869525 ) ) ;
#17714=CARTESIAN_POINT ( 'NONE',  ( -13.14518615778179189, 40.00781250108393294, 5.444914386472304635 ) ) ;
#17716=CARTESIAN_POINT ( 'NONE',  ( 65.00000000000000000, 38.56914062608393579, 13.14518615778179544 ) ) ;
#17717=CARTESIAN_POINT ( 'NONE',  ( 61.36350375319361916, 51.46815297079188412, -14.99999999999999822 ) ) ;
#17719=CARTESIAN_POINT ( 'NONE',  ( 208.5748159460630120, 40.65273437499998721, -5.622872871577873077 ) ) ;
#17722=ORIENTED_EDGE ( 'NONE', *, *, #4953, .T. ) ;
#17726=CARTESIAN_POINT ( 'NONE',  ( 55.40115559117954547, 36.43593750216787441, 9.598844408820459861 ) ) ;
#17727=CARTESIAN_POINT ( 'NONE',  ( 181.8548138422182205, 38.17226562608393436, 0.000000000000000000 ) ) ;
#17731=CARTESIAN_POINT ( 'NONE',  ( 200.4449143864723055, 40.20625000108394431, 13.14518615778179189 ) ) ;
#17737=CARTESIAN_POINT ( 'NONE',  ( 116.8548138422182205, 33.60820312608393579, 0.000000000000000000 ) ) ;
#17738=CARTESIAN_POINT ( 'NONE',  ( 70.44491438647230552, 33.95546875108393436, -13.14518615778179900 ) ) ;
#17740=CARTESIAN_POINT ( 'NONE',  ( 185.7049497278729575, 38.27148437608393294, -9.295050272127046043 ) ) ;
#17743=CARTESIAN_POINT ( 'NONE',  ( -9.295050272127044266, 31.92148437608393508, 9.295050272127047819 ) ) ;
#17745=LINE ( 'NONE', #15307, #10393 ) ;
#17749=CARTESIAN_POINT ( 'NONE',  ( 60.42840836746411526, 51.44262710532056815, 14.99999999999998046 ) ) ;
#17751=ORIENTED_EDGE ( 'NONE', *, *, #24711, .T. ) ;
#17752=( NAMED_UNIT ( * ) SI_UNIT ( $, .STERADIAN. ) SOLID_ANGLE_UNIT ( ) );
#17753=VERTEX_POINT ( 'NONE', #4362 ) ;
#17758=CARTESIAN_POINT ( 'NONE',  ( 65.00000000000000000, 37.72578125216787726, -13.57481594606304576 ) ) ;
#17761=CARTESIAN_POINT ( 'NONE',  ( 95.54126587499996504, 82.68750000136560629, -1.387778780781445676E-14 ) ) ;
#17762=CARTESIAN_POINT ( 'NONE',  ( 51.85481384221820633, 36.78320312608393294, 0.000000000000000000 ) ) ;
#17764=CARTESIAN_POINT ( 'NONE',  ( 13.14518615778179722, 36.23750000108393010, -5.444914386472297529 ) ) ;
#17765=CARTESIAN_POINT ( 'NONE',  ( 99.99999999999995737, 80.87500000273119838, -5.000000000000018652 ) ) ;
#17768=CARTESIAN_POINT ( 'NONE',  ( 139.5988444088204687, 38.12265624999999858, 9.598844408820456309 ) ) ;
#17774=CARTESIAN_POINT ( 'NONE',  ( 130.0000000000000000, 33.60820312608392868, 13.14518615778179544 ) ) ;
#17775=CARTESIAN_POINT ( 'NONE',  ( 55.40115559117954547, 33.06250000216787299, -9.598844408820458085 ) ) ;
#17777=VERTEX_POINT ( 'NONE', #11033 ) ;
#17778=CARTESIAN_POINT ( 'NONE',  ( 99.99999999999995737, 85.00000000000000000, -1.387778780781445676E-14 ) ) ;
#17779=CARTESIAN_POINT ( 'NONE',  ( 9.598844408820456309, 33.65781250216787157, -9.598844408820458085 ) ) ;
#17780=DIRECTION ( 'NONE',  ( 3.469446951953614682E-16, 0.000000000000000000, 1.000000000000000000 ) ) ;
#17783=CARTESIAN_POINT ( 'NONE',  ( 181.8548138422181921, 34.15390625108393863, -5.444914386472297529 ) ) ;
#17784=PLANE ( 'NONE',  #15634 ) ;
#17786=DIRECTION ( 'NONE',  ( 0.000000000000000000, 0.000000000000000000, 1.000000000000000000 ) ) ;
#17788=CARTESIAN_POINT ( 'NONE',  ( 131.8875287258764217, 53.66306546785491349, 14.99999999999996447 ) ) ;
#17794=CARTESIAN_POINT ( 'NONE',  ( 195.0000000000000000, 36.03906250000000000, -13.57481594606304576 ) ) ;
#17797=CARTESIAN_POINT ( 'NONE',  ( 78.14518615778179367, 36.18789062608393436, -1.609821015232357215E-15 ) ) ;
#17801=CARTESIAN_POINT ( 'NONE',  ( 13.57481594606304931, 37.37851562499999858, 5.622872871577869525 ) ) ;
#17802=CARTESIAN_POINT ( 'NONE',  ( 124.5550856135277087, 38.51953125108393294, 13.14518615778179722 ) ) ;
#17803=EDGE_LOOP ( 'NONE', ( #10678, #25718, #17382, #22862 ) ) ;
#17804=CARTESIAN_POINT ( 'NONE',  ( 101.8468681455906903, 80.37500000136562051, -4.458734125000016313 ) ) ;
#17806=CARTESIAN_POINT ( 'NONE',  ( 195.0000000000000000, -7.395377635281828788, -2.255140518769849538E-14 ) ) ;
#17807=CARTESIAN_POINT ( 'NONE',  ( 94.99999999999995737, 81.18750000273119838, 2.071067811865466624 ) ) ;
#17811=CARTESIAN_POINT ( 'NONE',  ( 55.70494972787295751, 31.92148437608393508, -9.295050272127046043 ) ) ;
#17817=CARTESIAN_POINT ( 'NONE',  ( 200.6228728715778686, 35.29492187716788720, -13.57481594606304753 ) ) ;
#17820=CARTESIAN_POINT ( 'NONE',  ( 139.2950502721270425, 36.28710937608393294, 9.295050272127046043 ) ) ;
#17822=CARTESIAN_POINT ( 'NONE',  ( 13.14518615778179900, 34.05468750108394005, -5.444914386472297529 ) ) ;
#17824=CARTESIAN_POINT ( 'NONE',  ( 74.59884440882045453, 34.35234374999999574, -9.598844408820458085 ) ) ;
#17827=DIRECTION ( 'NONE',  ( 0.000000000000000000, 0.000000000000000000, -1.000000000000000000 ) ) ;
#17828=ADVANCED_FACE ( 'NONE', ( #15312 ), #21346, .T. ) ;
#17831=CYLINDRICAL_SURFACE ( 'NONE', #2263, 11.57481594606304398 ) ;
#17832=DIRECTION ( 'NONE',  ( 0.000000000000000000, 0.000000000000000000, 1.000000000000000000 ) ) ;
#17834=CARTESIAN_POINT ( 'NONE',  ( -8.049105076161786076E-16, 34.99726562608393721, -13.14518615778179544 ) ) ;
#17841=ADVANCED_FACE ( 'NONE', ( #804 ), #13319, .T. ) ;
#17843=CARTESIAN_POINT ( 'NONE',  ( 195.0000000000000000, 35.98945312608393010, 13.14518615778179544 ) ) ;
#17845=DIRECTION ( 'NONE',  ( 0.000000000000000000, 0.000000000000000000, 1.000000000000000000 ) ) ;
#17852=CARTESIAN_POINT ( 'NONE',  ( 143.1451861577818079, 40.10703125108393152, 5.444914386472293977 ) ) ;
#17853=CARTESIAN_POINT ( 'NONE',  ( 13.14518615778179722, 39.51171875108393294, 5.444914386472293977 ) ) ;
#17855=CARTESIAN_POINT ( 'NONE',  ( 51.85481384221820633, 38.37070312608393152, 0.000000000000000000 ) ) ;
#17856=CARTESIAN_POINT ( 'NONE',  ( 61.19694562675306315, 54.09082899096448926, -14.99999999999999645 ) ) ;
#17859=CARTESIAN_POINT ( 'NONE',  ( 185.7049497278729575, 32.71523437608393436, -9.295050272127046043 ) ) ;
#17861=ORIENTED_EDGE ( 'NONE', *, *, #12410, .F. ) ;
#17864=CARTESIAN_POINT ( 'NONE',  ( 65.00000000000000000, 37.57695312608392868, 13.14518615778179544 ) ) ;
#17865=EDGE_CURVE ( 'NONE', #9074, #26975, #7943, .T. ) ;
#17866=CARTESIAN_POINT ( 'NONE',  ( 55.40115559117954547, 38.51953124999999289, -9.598844408820458085 ) ) ;
#17868=ORIENTED_EDGE ( 'NONE', *, *, #17964, .F. ) ;
#17870=ORIENTED_EDGE ( 'NONE', *, *, #6858, .F. ) ;
#17871=CARTESIAN_POINT ( 'NONE',  ( 204.2950502721270425, 38.86679687608393863, -9.295050272127046043 ) ) ;
#17873=VERTEX_POINT ( 'NONE', #10068 ) ;
#17876=ORIENTED_EDGE ( 'NONE', *, *, #26252, .F. ) ;
#17877=CARTESIAN_POINT ( 'NONE',  ( 124.5550856135277087, 32.16953125108393152, 13.14518615778179722 ) ) ;
#17880=CARTESIAN_POINT ( 'NONE',  ( 208.1451861577818079, 35.59257812608393579, -1.609821015232357215E-15 ) ) ;
#17884=CARTESIAN_POINT ( 'NONE',  ( 13.14518615778179900, 33.06250000108393294, -5.444914386472297529 ) ) ;
#17886=CARTESIAN_POINT ( 'NONE',  ( 70.62287287157788285, 40.45429687500001137, 13.57481594606306174 ) ) ;
#17888=DIRECTION ( 'NONE',  ( 0.000000000000000000, 0.000000000000000000, 1.000000000000000000 ) ) ;
#17890=CARTESIAN_POINT ( 'NONE',  ( 65.39699941464660071, 51.45716825712325715, 14.99999999999964118 ) ) ;
#17896=CARTESIAN_POINT ( 'NONE',  ( 143.5748159460630688, 38.37070312716787157, -5.622872871577873966 ) ) ;
#17900=CARTESIAN_POINT ( 'NONE',  ( 51.85481384221820633, 35.19570312608393436, 0.000000000000000000 ) ) ;
#17901=CARTESIAN_POINT ( 'NONE',  ( 195.0000000000000000, 37.62656249999999858, -13.57481594606304576 ) ) ;
#17902=CARTESIAN_POINT ( 'NONE',  ( 2.414731522848535132E-15, 38.37070312608393152, 13.14518615778179544 ) ) ;
#17904=CARTESIAN_POINT ( 'NONE',  ( 7.089417272335208686, 49.99999999943681672, 11.59823041028890955 ) ) ;
#17906=CARTESIAN_POINT ( 'NONE',  ( 135.6228728715778686, 37.57695312499998863, -13.57481594606304753 ) ) ;
#17908=ORIENTED_EDGE ( 'NONE', *, *, #16579, .T. ) ;
#17909=DIRECTION ( 'NONE',  ( -1.000000000000000000, 0.000000000000000000, 7.228014483236696740E-18 ) ) ;
#17913=CARTESIAN_POINT ( 'NONE',  ( 116.8548138422182205, 34.20351562608393436, 0.000000000000000000 ) ) ;
#17914=CARTESIAN_POINT ( 'NONE',  ( 70.62287287157786864, 33.70742187716787441, -13.57481594606304753 ) ) ;
#17916=CARTESIAN_POINT ( 'NONE',  ( 9.598844408820459861, 31.87187500216787228, 9.598844408820456309 ) ) ;
#17918=AXIS2_PLACEMENT_3D ( 'NONE', #12462, #14198, #24908 ) ;
#17919=CARTESIAN_POINT ( 'NONE',  ( 99.99999999999995737, 84.75000000000000000, -5.000000000000018652 ) ) ;
#17921=CARTESIAN_POINT ( 'NONE',  ( 200.4449143864723055, 32.86406250108392868, 13.14518615778179189 ) ) ;
#17929=CARTESIAN_POINT ( 'NONE',  ( 139.1801758136479918, 50.00000000000000000, 9.999999999999976907 ) ) ;
#17932=CARTESIAN_POINT ( 'NONE',  ( 208.5748159460630688, 33.45937499999999432, -1.662435489736055892E-15 ) ) ;
#17934=CARTESIAN_POINT ( 'NONE',  ( 130.0000000000000000, -7.395377635281828788, -13.57481594606305997 ) ) ;
#17936=CARTESIAN_POINT ( 'NONE',  ( 78.14518615778179367, 34.65000000108393152, -5.444914386472297529 ) ) ;
#17941=CARTESIAN_POINT ( 'NONE',  ( 13.57481594606304576, 34.25312499999999716, -1.662435489736055892E-15 ) ) ;
#17942=CARTESIAN_POINT ( 'NONE',  ( 143.1451861577818079, 37.13046875108393863, 5.444914386472293977 ) ) ;
#17944=CARTESIAN_POINT ( 'NONE',  ( 99.99999999999995737, 82.25000000000000000, 4.999999999999990230 ) ) ;
#17945=DIRECTION ( 'NONE',  ( 0.000000000000000000, 0.000000000000000000, 1.000000000000000000 ) ) ;
#17946=CARTESIAN_POINT ( 'NONE',  ( 104.9999999999999574, 82.68750000273121259, -2.071067811865491937 ) ) ;
#17951=CARTESIAN_POINT ( 'NONE',  ( 55.70494972787295751, 32.91367187608393152, 9.295050272127047819 ) ) ;
#17955=ORIENTED_EDGE ( 'NONE', *, *, #5487, .T. ) ;
#17957=CARTESIAN_POINT ( 'NONE',  ( 185.4011555911795597, 34.05468750216788010, 9.598844408820459861 ) ) ;
#17958=( BOUNDED_CURVE ( )  B_SPLINE_CURVE ( 2, ( #20346, #18053, #20063, #13623, #26769, #5098, #16342, #25041, #2950 ),
 .UNSPECIFIED., .F., .T. ) 
 B_SPLINE_CURVE_WITH_KNOTS ( ( 3, 2, 2, 2, 3 ),
 ( 0.3125000000000002220, 0.3229166666666668517, 0.3333333333333334259, 0.3437500000000000555, 0.3541666666666666852 ),
 .UNSPECIFIED. ) 
 CURVE ( )  GEOMETRIC_REPRESENTATION_ITEM ( )  RATIONAL_B_SPLINE_CURVE ( ( 0.9999999999999983347, 0.9238795325112884038, 1.000000000000000000, 0.9238795325112867385, 1.000000000000000000, 0.9238795325112867385, 1.000000000000000000, 0.9238795325112867385, 1.000000000000000000 ) ) 
 REPRESENTATION_ITEM ( '' )  );
#17959=ORIENTED_EDGE ( 'NONE', *, *, #8973, .T. ) ;
#17961=CARTESIAN_POINT ( 'NONE',  ( 74.18017581364799184, 55.00000000000000000, -9.999999999999998224 ) ) ;
#17962=CARTESIAN_POINT ( 'NONE',  ( 120.7049497278729575, 37.47773437608393010, -9.295050272127046043 ) ) ;
#17963=CARTESIAN_POINT ( 'NONE',  ( -8.049105076161786076E-16, 35.79101562608394005, -13.14518615778179544 ) ) ;
#17964=EDGE_CURVE ( 'NONE', #10805, #9259, #27191, .T. ) ;
#17966=CARTESIAN_POINT ( 'NONE',  ( 51.42518405393695957, 32.21914062500000142, -5.622872871577873077 ) ) ;
#17968=CARTESIAN_POINT ( 'NONE',  ( 123.6617092076501905, 35.99999999999997868, 11.53992004315006703 ) ) ;
#17970=FACE_OUTER_BOUND ( 'NONE', #19733, .T. ) ;
#17977=CARTESIAN_POINT ( 'NONE',  ( 9.295050272127046043, 36.48554687608393721, -9.295050272127046043 ) ) ;
#17978=ORIENTED_EDGE ( 'NONE', *, *, #2542, .T. ) ;
#17981=CARTESIAN_POINT ( 'NONE',  ( 200.4449143864723055, 34.45156250108393436, 13.14518615778179189 ) ) ;
#17983=CARTESIAN_POINT ( 'NONE',  ( 99.99999999999995737, 85.00000000000000000, -1.387778780781445676E-14 ) ) ;
#17987=CIRCLE ( 'NONE', #27129, 5.000000000000000000 ) ;
#17990=CARTESIAN_POINT ( 'NONE',  ( 135.4449143864723055, 36.83281250108392868, 13.14518615778179189 ) ) ;
#17991=CARTESIAN_POINT ( 'NONE',  ( -8.049105076161786076E-16, 40.55351562608393579, -13.14518615778179544 ) ) ;
#17992=CARTESIAN_POINT ( 'NONE',  ( 13.14518615778179900, 35.44375000108393436, -5.444914386472297529 ) ) ;
#17995=CARTESIAN_POINT ( 'NONE',  ( 65.00000000000000000, 36.98164062608393721, 13.14518615778179544 ) ) ;
#17996=CARTESIAN_POINT ( 'NONE',  ( 67.16995658311145689, 49.99999999883969082, -13.43548448457778477 ) ) ;
#17999=CARTESIAN_POINT ( 'NONE',  ( 195.0000000000000000, 32.61601562608393579, -13.14518615778179544 ) ) ;
#18001=VERTEX_POINT ( 'NONE', #26461 ) ;
#18004=CARTESIAN_POINT ( 'NONE',  ( 51.85481384221820633, 37.32890625108393579, -5.444914386472297529 ) ) ;
#18006=CARTESIAN_POINT ( 'NONE',  ( 200.4449143864723055, 36.33671875108393579, -13.14518615778179722 ) ) ;
#18008=( BOUNDED_CURVE ( )  B_SPLINE_CURVE ( 2, ( #10215, #7679, #16515, #5695, #23078, #12210, #20937, #1421, #16788 ),
 .UNSPECIFIED., .F., .F. ) 
 B_SPLINE_CURVE_WITH_KNOTS ( ( 3, 2, 2, 2, 3 ),
 ( 0.2708333333333330928, 0.2812499999999998890, 0.2916666666666666852, 0.3020833333333334259, 0.3125000000000002220 ),
 .UNSPECIFIED. ) 
 CURVE ( )  GEOMETRIC_REPRESENTATION_ITEM ( )  RATIONAL_B_SPLINE_CURVE ( ( 1.000000000000001554, 0.9238795325112850731, 1.000000000000000000, 0.9238795325112867385, 1.000000000000000000, 0.9238795325112867385, 1.000000000000000000, 0.9238795325112850731, 1.000000000000001554 ) ) 
 REPRESENTATION_ITEM ( '' )  );
#18010=CARTESIAN_POINT ( 'NONE',  ( 181.8548138422182205, 37.62656250108393152, 5.444914386472304635 ) ) ;
#18012=ORIENTED_EDGE ( 'NONE', *, *, #2573, .T. ) ;
#18016=CARTESIAN_POINT ( 'NONE',  ( 124.5550856135277087, 34.25312500108393010, -13.14518615778179900 ) ) ;
#18018=CARTESIAN_POINT ( 'NONE',  ( 181.8548138422181921, 32.86406250108393579, 5.444914386472304635 ) ) ;
#18021=CARTESIAN_POINT ( 'NONE',  ( -0.9830651850993568086, 49.99999999948985874, -13.54930971656723493 ) ) ;
#18026=CARTESIAN_POINT ( 'NONE',  ( 73.76938967208273823, 50.37710889401973446, 15.00000000000719602 ) ) ;
#18027=ORIENTED_EDGE ( 'NONE', *, *, #13351, .F. ) ;
#18029=AXIS2_PLACEMENT_3D ( 'NONE', #21467, #26153, #25730 ) ;
#18030=ORIENTED_EDGE ( 'NONE', *, *, #6530, .T. ) ;
#18033=CARTESIAN_POINT ( 'NONE',  ( 135.6228728715779255, 38.46992187716787726, -13.57481594606299247 ) ) ;
#18036=FACE_OUTER_BOUND ( 'NONE', #19797, .T. ) ;
#18037=CARTESIAN_POINT ( 'NONE',  ( 70.62287287157776916, 37.67617187716787441, -13.57481594606313990 ) ) ;
#18039=CARTESIAN_POINT ( 'NONE',  ( -13.14518615778179544, 37.37851562608393863, 0.000000000000000000 ) ) ;
#18040=( BOUNDED_SURFACE ( )  B_SPLINE_SURFACE ( 1, 2, ( 
 ( #9821, #23085, #10086, #11808, #20672, #14092, #16379, #20531, #25357, #2988, #1156, #12218, #5567, #1013, #22952, #25214, #3279, #14230, #7828, #25079, #11948, #3559, #9955, #16239, #18798, #18528, #27505, #3414, #5276, #27233, #16521, #16088, #7688, #12082, #24936, #24794, #7394, #20945, #13942, #20806, #16660, #5838, #1286, #22523, #27369, #7961, #11662, #871, #5423, #18667, #5702, #20384, #9682, #14369, #9542, #22811, #18243, #26951, #22668, #18385, #27640, #15054, #4112, #1569, #21362, #21494, #17205, #21640, #25910, #6108, #6382, #10780, #19351, #28053, #14775, #23771, #8520, #23358, #12778, #10222, #14915, #26046, #3831, #4247, #19071, #12907, #2113, #18932, #25626, #17350, #14507, #19212, #23636, #12493, #19492, #12635, #8101, #28191, #27777, #23495, #1975, #21219, #3700, #8236, #16795, #1843, #10645, #3975, #1703, #23224, #16927, #10506, #10361, #8659, #12362, #21080, #25493, #27915, #5973, #8376, #14640, #17061, #25764, #6246, #13624, #15338, #4675, #26336, #401, #24053, #9361, #15192, #13337, #24478, #17779, #4529, #6937, #9224, #15482, #26482, #20064, #9083, #24196, #7075, #22202, #19771, #22345, #2541, #2816, #15632, #17487, #22064, #543, #114, #11201, #19917, #254, #8796, #19632, #4962, #26186, #24333, #686, #6652, #23910, #4819, #11484, #13479, #20200, #8938, #17916, #4390, #6795, #26627, #18054, #11341, #15770, #2679, #6516, #13047, #13190, #21782, #2262 ),
 ( #10923, #21926, #2402, #11060, #17628, #11768, #16197, #22486, #25175, #5099, #5525, #24903, #976, #26770, #22911, #5383, #27333, #11624, #1253, #18202, #9501, #18492, #14053, #18347, #22633, #16050, #3522, #27199, #833, #12181, #5664, #13905, #1115, #7793, #14328, #24760, #9643, #20347, #16479, #26912, #9914, #22774, #3240, #20768, #7651, #18630, #15904, #7213, #23047, #20909, #27052, #20632, #1391, #7503, #10053, #11908, #24622, #13763, #2951, #7357, #9783, #5240, #3102, #16343, #25042, #14191, #20492, #3373, #12043, #3663, #23739, #12597, #15018, #12871, #3937, #6074, #19176, #21323, #25590, #6211, #21601, #25728, #16756, #2079, #10468, #18764, #23595, #28018, #27467, #25313, #3796, #1803, #23460, #6343, #8061, #21464, #12740, #23323, #10323, #7924, #16892, #27879, #12325, #19317, #8340, #5803, #14741, #14880, #8201, #8484, #21045, #1941, #10181, #1529, #17025, #4078, #19029, #14605, #25456, #4214, #10610, #18891, #16622, #25875, #5937, #17173, #14469, #23187, #12456, #21181, #27601, #1663, #27741, #22167, #17594, #6763, #4780, #11163, #2645, #28156, #19458, #11307, #508, #21894, #4638, #9189, #11022, #20029, #2366, #15735, #24439, #17884, #8622, #13296, #78, #15303, #13155, #19735, #26301, #21748, #10747, #4497, #23875, #4926, #22024, #7036, #13589, #24161, #15446, #19879, #2502, #364, #26444, #22311, #17743, #8763, #17311, #9051, #26011, #15592, #26589, #6482, #15156 ) ),
 .UNSPECIFIED., .F., .F., .T. ) 
 B_SPLINE_SURFACE_WITH_KNOTS ( ( 2, 2 ),
 ( 3, 2, 2, 2, 2, 2, 2, 2, 2, 2, 2, 2, 2, 2, 2, 2, 2, 2, 2, 2, 2, 2, 2, 2, 2, 2, 2, 2, 2, 2, 2, 2, 2, 2, 2, 2, 2, 2, 2, 2, 2, 2, 2, 2, 2, 2, 2, 2, 2, 2, 2, 2, 2, 2, 2, 2, 2, 2, 2, 2, 2, 2, 2, 2, 2, 2, 2, 2, 2, 2, 2, 2, 2, 2, 2, 2, 2, 2, 2, 2, 2, 2, 2, 2, 2, 2, 2, 2, 2, 2, 2, 3 ),
 ( 0.000000000000000000, 1.000000000000000000 ),
 ( 0.000000000000000000, 0.01041666666666666609, 0.02083333333333333218, 0.03125000000000000000, 0.04166666666666666435, 0.05208333333333333565, 0.06250000000000000000, 0.07291666666666667129, 0.08333333333333332871, 0.09375000000000000000, 0.1041666666666666713, 0.1145833333333333287, 0.1250000000000000000, 0.1354166666666666574, 0.1458333333333333426, 0.1562500000000000000, 0.1666666666666666574, 0.1770833333333333426, 0.1875000000000000000, 0.1979166666666666574, 0.2083333333333333426, 0.2187500000000000000, 0.2291666666666666574, 0.2395833333333333426, 0.2500000000000000000, 0.2604166666666666852, 0.2708333333333333148, 0.2812500000000000000, 0.2916666666666666852, 0.3020833333333333148, 0.3125000000000000000, 0.3229166666666666852, 0.3333333333333333148, 0.3437500000000000000, 0.3541666666666666852, 0.3645833333333333148, 0.3750000000000000000, 0.3854166666666666852, 0.3958333333333333148, 0.4062500000000000000, 0.4166666666666666852, 0.4270833333333333148, 0.4375000000000000000, 0.4479166666666666852, 0.4583333333333333148, 0.4687500000000000000, 0.4791666666666666852, 0.4895833333333333148, 0.5000000000000000000, 0.5104166666666666297, 0.5208333333333333703, 0.5312500000000000000, 0.5416666666666666297, 0.5520833333333333703, 0.5625000000000000000, 0.5729166666666666297, 0.5833333333333333703, 0.5937500000000000000, 0.6041666666666666297, 0.6145833333333333703, 0.6250000000000000000, 0.6354166666666666297, 0.6458333333333333703, 0.6562500000000000000, 0.6666666666666666297, 0.6770833333333333703, 0.6875000000000000000, 0.6979166666666666297, 0.7083333333333333703, 0.7187500000000000000, 0.7291666666666666297, 0.7395833333333333703, 0.7500000000000000000, 0.7604166666666666297, 0.7708333333333333703, 0.7812500000000000000, 0.7916666666666666297, 0.8020833333333333703, 0.8125000000000000000, 0.8229166666666666297, 0.8333333333333333703, 0.8437500000000000000, 0.8541666666666666297, 0.8645833333333333703, 0.8750000000000000000, 0.8854166666666666297, 0.8958333333333333703, 0.9062500000000000000, 0.9166666666666666297, 0.9270833333333333703, 0.9375000000000000000, 0.9448586970929392370 ),
 .UNSPECIFIED. ) 
 GEOMETRIC_REPRESENTATION_ITEM ( )  RATIONAL_B_SPLINE_SURFACE ( (
 ( 1.000000000000000000, 0.9238795325112867385, 1.000000000000000000, 0.9238795325112867385, 1.000000000000000000, 0.9238795325112867385, 1.000000000000000000, 0.9238795325112867385, 1.000000000000000000, 0.9238795325112867385, 1.000000000000000000, 0.9238795325112867385, 1.000000000000000000, 0.9238795325112867385, 1.000000000000000000, 0.9238795325112867385, 1.000000000000000000, 0.9238795325112867385, 1.000000000000000000, 0.9238795325112867385, 1.000000000000000000, 0.9238795325112867385, 1.000000000000000000, 0.9238795325112867385, 1.000000000000000000, 0.9238795325112867385, 1.000000000000000000, 0.9238795325112867385, 1.000000000000000000, 0.9238795325112867385, 1.000000000000000000, 0.9238795325112867385, 1.000000000000000000, 0.9238795325112867385, 1.000000000000000000, 0.9238795325112867385, 1.000000000000000000, 0.9238795325112867385, 1.000000000000000000, 0.9238795325112867385, 1.000000000000000000, 0.9238795325112867385, 1.000000000000000000, 0.9238795325112867385, 1.000000000000000000, 0.9238795325112867385, 1.000000000000000000, 0.9238795325112867385, 1.000000000000000000, 0.9238795325112867385, 1.000000000000000000, 0.9238795325112867385, 1.000000000000000000, 0.9238795325112867385, 1.000000000000000000, 0.9238795325112867385, 1.000000000000000000, 0.9238795325112867385, 1.000000000000000000, 0.9238795325112867385, 1.000000000000000000, 0.9238795325112867385, 1.000000000000000000, 0.9238795325112867385, 1.000000000000000000, 0.9238795325112867385, 1.000000000000000000, 0.9238795325112867385, 1.000000000000000000, 0.9238795325112867385, 1.000000000000000000, 0.9238795325112867385, 1.000000000000000000, 0.9238795325112867385, 1.000000000000000000, 0.9238795325112867385, 1.000000000000000000, 0.9238795325112867385, 1.000000000000000000, 0.9238795325112867385, 1.000000000000000000, 0.9238795325112867385, 1.000000000000000000, 0.9238795325112867385, 1.000000000000000000, 0.9238795325112867385, 1.000000000000000000, 0.9238795325112867385, 1.000000000000000000, 0.9238795325112867385, 1.000000000000000000, 0.9238795325112867385, 1.000000000000000000, 0.9238795325112867385, 1.000000000000000000, 0.9238795325112867385, 1.000000000000000000, 0.9238795325112867385, 1.000000000000000000, 0.9238795325112867385, 1.000000000000000000, 0.9238795325112867385, 1.000000000000000000, 0.9238795325112867385, 1.000000000000000000, 0.9238795325112867385, 1.000000000000000000, 0.9238795325112867385, 1.000000000000000000, 0.9238795325112867385, 1.000000000000000000, 0.9238795325112867385, 1.000000000000000000, 0.9238795325112867385, 1.000000000000000000, 0.9238795325112867385, 1.000000000000000000, 0.9238795325112867385, 1.000000000000000000, 0.9238795325112867385, 1.000000000000000000, 0.9238795325112867385, 1.000000000000000000, 0.9238795325112867385, 1.000000000000000000, 0.9238795325112867385, 1.000000000000000000, 0.9238795325112867385, 1.000000000000000000, 0.9238795325112867385, 1.000000000000000000, 0.9238795325112867385, 1.000000000000000000, 0.9238795325112867385, 1.000000000000000000, 0.9238795325112867385, 1.000000000000000000, 0.9238795325112867385, 1.000000000000000000, 0.9238795325112867385, 1.000000000000000000, 0.9238795325112867385, 1.000000000000000000, 0.9238795325112867385, 1.000000000000000000, 0.9238795325112867385, 1.000000000000000000, 0.9238795325112867385, 1.000000000000000000, 0.9238795325112867385, 1.000000000000000000, 0.9238795325112867385, 1.000000000000000000, 0.9238795325112867385, 1.000000000000000000, 0.9238795325112867385, 1.000000000000000000, 0.9238795325112867385, 1.000000000000000000, 0.9238795325112867385, 1.000000000000000000, 0.9238795325112867385, 1.000000000000000000, 0.9238795325112867385, 1.000000000000000000, 0.9238795325112867385, 1.000000000000000000, 0.9238795325112867385, 1.000000000000000000, 0.9238795325112867385, 1.000000000000000000, 0.9238795325112867385, 1.000000000000000000, 0.9238795325112867385, 1.000000000000000000, 0.9238795325112867385, 1.000000000000000000, 0.9238795325112867385, 1.000000000000000000, 0.9238795325112867385, 1.000000000000000000, 0.9462258435690522607, 0.9684275710300105366),
 ( 1.000000000000000000, 0.9238795325112867385, 1.000000000000000000, 0.9238795325112867385, 1.000000000000000000, 0.9238795325112867385, 1.000000000000000000, 0.9238795325112867385, 1.000000000000000000, 0.9238795325112867385, 1.000000000000000000, 0.9238795325112867385, 1.000000000000000000, 0.9238795325112867385, 1.000000000000000000, 0.9238795325112867385, 1.000000000000000000, 0.9238795325112867385, 1.000000000000000000, 0.9238795325112867385, 1.000000000000000000, 0.9238795325112867385, 1.000000000000000000, 0.9238795325112867385, 1.000000000000000000, 0.9238795325112867385, 1.000000000000000000, 0.9238795325112867385, 1.000000000000000000, 0.9238795325112867385, 1.000000000000000000, 0.9238795325112867385, 1.000000000000000000, 0.9238795325112867385, 1.000000000000000000, 0.9238795325112867385, 1.000000000000000000, 0.9238795325112867385, 1.000000000000000000, 0.9238795325112867385, 1.000000000000000000, 0.9238795325112867385, 1.000000000000000000, 0.9238795325112867385, 1.000000000000000000, 0.9238795325112867385, 1.000000000000000000, 0.9238795325112867385, 1.000000000000000000, 0.9238795325112867385, 1.000000000000000000, 0.9238795325112867385, 1.000000000000000000, 0.9238795325112867385, 1.000000000000000000, 0.9238795325112867385, 1.000000000000000000, 0.9238795325112867385, 1.000000000000000000, 0.9238795325112867385, 1.000000000000000000, 0.9238795325112867385, 1.000000000000000000, 0.9238795325112867385, 1.000000000000000000, 0.9238795325112867385, 1.000000000000000000, 0.9238795325112867385, 1.000000000000000000, 0.9238795325112867385, 1.000000000000000000, 0.9238795325112867385, 1.000000000000000000, 0.9238795325112867385, 1.000000000000000000, 0.9238795325112867385, 1.000000000000000000, 0.9238795325112867385, 1.000000000000000000, 0.9238795325112867385, 1.000000000000000000, 0.9238795325112867385, 1.000000000000000000, 0.9238795325112867385, 1.000000000000000000, 0.9238795325112867385, 1.000000000000000000, 0.9238795325112867385, 1.000000000000000000, 0.9238795325112867385, 1.000000000000000000, 0.9238795325112867385, 1.000000000000000000, 0.9238795325112867385, 1.000000000000000000, 0.9238795325112867385, 1.000000000000000000, 0.9238795325112867385, 1.000000000000000000, 0.9238795325112867385, 1.000000000000000000, 0.9238795325112867385, 1.000000000000000000, 0.9238795325112867385, 1.000000000000000000, 0.9238795325112867385, 1.000000000000000000, 0.9238795325112867385, 1.000000000000000000, 0.9238795325112867385, 1.000000000000000000, 0.9238795325112867385, 1.000000000000000000, 0.9238795325112867385, 1.000000000000000000, 0.9238795325112867385, 1.000000000000000000, 0.9238795325112867385, 1.000000000000000000, 0.9238795325112867385, 1.000000000000000000, 0.9238795325112867385, 1.000000000000000000, 0.9238795325112867385, 1.000000000000000000, 0.9238795325112867385, 1.000000000000000000, 0.9238795325112867385, 1.000000000000000000, 0.9238795325112867385, 1.000000000000000000, 0.9238795325112867385, 1.000000000000000000, 0.9238795325112867385, 1.000000000000000000, 0.9238795325112867385, 1.000000000000000000, 0.9238795325112867385, 1.000000000000000000, 0.9238795325112867385, 1.000000000000000000, 0.9238795325112867385, 1.000000000000000000, 0.9238795325112867385, 1.000000000000000000, 0.9238795325112867385, 1.000000000000000000, 0.9238795325112867385, 1.000000000000000000, 0.9238795325112867385, 1.000000000000000000, 0.9238795325112867385, 1.000000000000000000, 0.9238795325112867385, 1.000000000000000000, 0.9238795325112867385, 1.000000000000000000, 0.9238795325112867385, 1.000000000000000000, 0.9238795325112867385, 1.000000000000000000, 0.9238795325112867385, 1.000000000000000000, 0.9238795325112867385, 1.000000000000000000, 0.9238795325112867385, 1.000000000000000000, 0.9238795325112867385, 1.000000000000000000, 0.9238795325112867385, 1.000000000000000000, 0.9238795325112867385, 1.000000000000000000, 0.9238795325112867385, 1.000000000000000000, 0.9238795325112867385, 1.000000000000000000, 0.9238795325112867385, 1.000000000000000000, 0.9238795325112867385, 1.000000000000000000, 0.9462258435690522607, 0.9684275710300105366) ) ) 
 REPRESENTATION_ITEM ( '' )  SURFACE ( )  );
#18041=CARTESIAN_POINT ( 'NONE',  ( -6.161062174842506955, 51.27996893917265453, 14.99999999999930900 ) ) ;
#18043=CARTESIAN_POINT ( 'NONE',  ( 139.5988444088204403, 35.14609374999999858, -9.598844408820458085 ) ) ;
#18044=ADVANCED_FACE ( 'NONE', ( #6634 ), #17336, .T. ) ;
#18045=EDGE_LOOP ( 'NONE', ( #15046, #1632, #27284, #22953 ) ) ;
#18051=CARTESIAN_POINT ( 'NONE',  ( 120.7049497278729575, 33.31054687608393294, -9.295050272127046043 ) ) ;
#18052=CARTESIAN_POINT ( 'NONE',  ( 78.14518615778179367, 38.61875000108393152, -5.444914386472297529 ) ) ;
#18053=CARTESIAN_POINT ( 'NONE',  ( 59.37712712842203189, 37.27929687716785878, 13.57481594606295161 ) ) ;
#18054=CARTESIAN_POINT ( 'NONE',  ( -9.598844408820454532, 31.67343750216787512, 9.598844408820459861 ) ) ;
#18059=CARTESIAN_POINT ( 'NONE',  ( 181.8548138422181921, 33.36015625108393579, -5.444914386472297529 ) ) ;
#18060=DIRECTION ( 'NONE',  ( 1.000000000000000000, 0.000000000000000000, -5.551115123125784280E-15 ) ) ;
#18061=DIRECTION ( 'NONE',  ( 0.000000000000000000, 0.000000000000000000, -1.000000000000000000 ) ) ;
#18072=EDGE_CURVE ( 'NONE', #6018, #13666, #1872, .T. ) ;
#18075=CARTESIAN_POINT ( 'NONE',  ( 98.15313185440925281, 83.25000000136560629, -4.458734125000016313 ) ) ;
#18076=CARTESIAN_POINT ( 'NONE',  ( 51.85481384221820633, 32.66562500108393863, 5.444914386472304635 ) ) ;
#18079=ORIENTED_EDGE ( 'NONE', *, *, #15572, .F. ) ;
#18081=CARTESIAN_POINT ( 'NONE',  ( -13.57481594606304753, 34.60039062499999574, -5.622872871577873077 ) ) ;
#18082=CARTESIAN_POINT ( 'NONE',  ( 124.5550856135277087, 37.42812500108394147, -13.14518615778179900 ) ) ;
#18083=ORIENTED_EDGE ( 'NONE', *, *, #25674, .F. ) ;
#18084=CARTESIAN_POINT ( 'NONE',  ( -20.00000000000000000, 75.00000000000000000, 15.00000000000000178 ) ) ;
#18086=CARTESIAN_POINT ( 'NONE',  ( 101.8468681455906903, 84.12500000136560629, -4.458734125000016313 ) ) ;
#18089=( BOUNDED_CURVE ( )  B_SPLINE_CURVE ( 2, ( #19923, #23918, #9090, #13053, #2268, #23776, #6945, #2119, #4829 ),
 .UNSPECIFIED., .F., .F. ) 
 B_SPLINE_CURVE_WITH_KNOTS ( ( 3, 2, 2, 2, 3 ),
 ( 0.6500000000000005773, 0.6750000000000005995, 0.7000000000000006217, 0.7250000000000006439, 0.7500000000000006661 ),
 .UNSPECIFIED. ) 
 CURVE ( )  GEOMETRIC_REPRESENTATION_ITEM ( )  RATIONAL_B_SPLINE_CURVE ( ( 0.9999999999999983347, 0.9238795325112884038, 1.000000000000000000, 0.9238795325112867385, 1.000000000000000000, 0.9238795325112867385, 1.000000000000000000, 0.9238795325112847401, 1.000000000000001998 ) ) 
 REPRESENTATION_ITEM ( '' )  );
#18091=CARTESIAN_POINT ( 'NONE',  ( 51.85481384221820633, 32.86406250108393579, 5.444914386472304635 ) ) ;
#18092=ORIENTED_EDGE ( 'NONE', *, *, #10643, .F. ) ;
#18094=CIRCLE ( 'NONE', #9439, 5.000000000000000000 ) ;
#18099=CARTESIAN_POINT ( 'NONE',  ( 208.5748159460630120, 34.30273437716787299, 5.622872871577869525 ) ) ;
#18103=CARTESIAN_POINT ( 'NONE',  ( 219.9999999999999716, 55.00000000000000000, 9.999999999999946709 ) ) ;
#18105=CARTESIAN_POINT ( 'NONE',  ( 13.14518615778179544, 34.79882812608394005, -1.609821015232357215E-15 ) ) ;
#18110=PLANE ( 'NONE',  #7732 ) ;
#18112=CARTESIAN_POINT ( 'NONE',  ( 134.1572863549629062, 35.99999999999997158, -12.92256159328817411 ) ) ;
#18115=CARTESIAN_POINT ( 'NONE',  ( 0.000000000000000000, -7.395377635281828788, 0.000000000000000000 ) ) ;
#18116=DIRECTION ( 'NONE',  ( 0.000000000000000000, 0.000000000000000000, -1.000000000000000000 ) ) ;
#18117=DIRECTION ( 'NONE',  ( 0.000000000000000000, 0.000000000000000000, 1.000000000000000000 ) ) ;
#18118=CARTESIAN_POINT ( 'NONE',  ( 9.295050272127047819, 32.31835937608393294, 9.295050272127046043 ) ) ;
#18119=ORIENTED_EDGE ( 'NONE', *, *, #26391, .F. ) ;
#18122=CARTESIAN_POINT ( 'NONE',  ( -13.57481594606304753, 36.18789062499999432, -5.622872871577872189 ) ) ;
#18124=CARTESIAN_POINT ( 'NONE',  ( 189.5550856135277229, 34.84843750108393579, -13.14518615778179900 ) ) ;
#18127=CARTESIAN_POINT ( 'NONE',  ( 5.622872871577976994, 40.05742187716787583, -13.57481594606294095 ) ) ;
#18134=AXIS2_PLACEMENT_3D ( 'NONE', #5232, #24895, #13898 ) ;
#18135=CARTESIAN_POINT ( 'NONE',  ( 143.1451861577818079, 36.98164062608393010, -1.609821015232357215E-15 ) ) ;
#18136=CARTESIAN_POINT ( 'NONE',  ( 13.14518615778179544, 37.18007812608393436, -1.609821015232357215E-15 ) ) ;
#18137=CARTESIAN_POINT ( 'NONE',  ( -5.444914386472299306, 34.35234375108392868, 13.14518615778179722 ) ) ;
#18140=CARTESIAN_POINT ( 'NONE',  ( 2.493653234604083739E-15, 36.53515625216787299, 13.57481594606304576 ) ) ;
#18142=CARTESIAN_POINT ( 'NONE',  ( 195.0000000000000000, 39.61093749999999147, 13.57481594606304576 ) ) ;
#18143=CARTESIAN_POINT ( 'NONE',  ( 74.03144042245413914, 36.00000000000002132, 9.765766397119163500 ) ) ;
#18147=CARTESIAN_POINT ( 'NONE',  ( 74.29505027212704249, 36.28710937608393294, -9.295050272127046043 ) ) ;
#18149=CARTESIAN_POINT ( 'NONE',  ( 181.8548138422182205, 36.63437500108393863, 5.444914386472304635 ) ) ;
#18151=ORIENTED_EDGE ( 'NONE', *, *, #5141, .T. ) ;
#18154=CARTESIAN_POINT ( 'NONE',  ( 195.0000000000000000, 36.98164062608393721, 13.14518615778179544 ) ) ;
#18157=VERTEX_POINT ( 'NONE', #20182 ) ;
#18158=EDGE_CURVE ( 'NONE', #1420, #21223, #6590, .T. ) ;
#18161=CIRCLE ( 'NONE', #26341, 11.57481594606304398 ) ;
#18162=ORIENTED_EDGE ( 'NONE', *, *, #19982, .F. ) ;
#18163=CARTESIAN_POINT ( 'NONE',  ( 130.0000000000000000, 31.82226562608393650, -13.14518615778179544 ) ) ;
#18164=CARTESIAN_POINT ( 'NONE',  ( 181.4251840539369596, 37.18007812716787441, 5.622872871577880183 ) ) ;
#18165=CARTESIAN_POINT ( 'NONE',  ( 208.1451861577818079, 34.00507812608393721, -1.609821015232357215E-15 ) ) ;
#18168=FACE_OUTER_BOUND ( 'NONE', #16155, .T. ) ;
#18170=CARTESIAN_POINT ( 'NONE',  ( 135.6228728715778971, 36.58476562716787583, 13.57481594606304576 ) ) ;
#18174=CARTESIAN_POINT ( 'NONE',  ( 195.0000000000000000, 40.55351562608393579, -13.14518615778179544 ) ) ;
#18178=EDGE_LOOP ( 'NONE', ( #4331, #2009, #16240, #26473 ) ) ;
#18187=CARTESIAN_POINT ( 'NONE',  ( -8.312177448680279460E-16, 39.31328125216787583, -13.57481594606304576 ) ) ;
#18189=FACE_OUTER_BOUND ( 'NONE', #11099, .T. ) ;
#18190=CARTESIAN_POINT ( 'NONE',  ( 130.0000000000000000, 40.40468749999999432, 13.57481594606304576 ) ) ;
#18191=CARTESIAN_POINT ( 'NONE',  ( 143.5748159460630688, 33.45937499999999432, -1.662435489736055892E-15 ) ) ;
#18193=LINE ( 'NONE', #15762, #25862 ) ;
#18197=CARTESIAN_POINT ( 'NONE',  ( 143.1451861577818079, 33.01289062608393010, -1.609821015232357215E-15 ) ) ;
#18199=CARTESIAN_POINT ( 'NONE',  ( 55.70494972787295751, 39.06523437608392868, 9.295050272127047819 ) ) ;
#18202=CARTESIAN_POINT ( 'NONE',  ( -5.444914386472297529, 39.61093750108393152, -13.14518615778179900 ) ) ;
#18203=EDGE_CURVE ( 'NONE', #15512, #10978, #5504, .T. ) ;
#18209=CARTESIAN_POINT ( 'NONE',  ( -13.14518615778179544, 40.65273437608393436, 0.000000000000000000 ) ) ;
#18213=CARTESIAN_POINT ( 'NONE',  ( 118.0647576233092764, 36.00000000000000711, -5.809862729997675501 ) ) ;
#18215=DIRECTION ( 'NONE',  ( -0.000000000000000000, -1.000000000000000000, -0.000000000000000000 ) ) ;
#18226=CARTESIAN_POINT ( 'NONE',  ( 74.29505027212704249, 32.11992187608393579, 9.295050272127046043 ) ) ;
#18227=DIRECTION ( 'NONE',  ( -0.000000000000000000, -1.000000000000000000, -0.000000000000000000 ) ) ;
#18229=CARTESIAN_POINT ( 'NONE',  ( 2.493653234604083739E-15, 32.46718749999999432, 13.57481594606304576 ) ) ;
#18230=CARTESIAN_POINT ( 'NONE',  ( 120.7049497278729575, 35.09648437608393579, -9.295050272127046043 ) ) ;
#18233=CARTESIAN_POINT ( 'NONE',  ( 102.0710678118654329, 82.31250000000000000, 4.999999999999989342 ) ) ;
#18236=CARTESIAN_POINT ( 'NONE',  ( 95.54126587499995082, 82.50000000136560629, 1.846868145590724986 ) ) ;
#18238=CARTESIAN_POINT ( 'NONE',  ( 200.6228728715779255, 37.27929687499999289, 13.57481594606297115 ) ) ;
#18240=EDGE_CURVE ( 'NONE', #28031, #7991, #22095, .T. ) ;
#18242=CARTESIAN_POINT ( 'NONE',  ( 74.59884440882045453, 39.90859374999999432, -9.598844408820458085 ) ) ;
#18243=CARTESIAN_POINT ( 'NONE',  ( 13.57481594606304576, 37.52734375216787299, -1.662435489736055892E-15 ) ) ;
#18246=EDGE_CURVE ( 'NONE', #13216, #467, #4606, .T. ) ;
#18250=CARTESIAN_POINT ( 'NONE',  ( 195.0000000000000000, 32.56640625216787299, 13.57481594606304576 ) ) ;
#18254=CARTESIAN_POINT ( 'NONE',  ( -8.049105076161786076E-16, 36.58476562608393579, -13.14518615778179544 ) ) ;
#18259=CARTESIAN_POINT ( 'NONE',  ( 70.62287287157786864, 36.88242187716787157, -13.57481594606304753 ) ) ;
#18268=CARTESIAN_POINT ( 'NONE',  ( 9.295050272127046043, 32.51679687608393721, -9.295050272127046043 ) ) ;
#18273=AXIS2_PLACEMENT_3D ( 'NONE', #22735, #23290, #22875 ) ;
#18275=CARTESIAN_POINT ( 'NONE',  ( 189.5550856135277229, 35.93984375108392726, 13.14518615778179722 ) ) ;
#18276=VERTEX_POINT ( 'NONE', #9898 ) ;
#18277=CARTESIAN_POINT ( 'NONE',  ( 185.8198241863518945, 55.00000000000000000, -15.00000000000000000 ) ) ;
#18284=CARTESIAN_POINT ( 'NONE',  ( 116.8548138422182063, 39.01562500108393294, 5.444914386472304635 ) ) ;
#18285=CARTESIAN_POINT ( 'NONE',  ( 13.14518615778179544, 37.97382812608393721, -1.609821015232357215E-15 ) ) ;
#18286=CARTESIAN_POINT ( 'NONE',  ( -8.049105076161786076E-16, 34.00507812608393721, -13.14518615778179544 ) ) ;
#18288=CARTESIAN_POINT ( 'NONE',  ( 66.94732592208626443, 51.47162402671428083, -15.00000000000065725 ) ) ;
#18291=DIRECTION ( 'NONE',  ( -0.000000000000000000, 1.000000000000000000, -0.000000000000000000 ) ) ;
#18294=CARTESIAN_POINT ( 'NONE',  ( 74.29505027212704249, 37.08085937608393579, -9.295050272127046043 ) ) ;
#18300=CARTESIAN_POINT ( 'NONE',  ( 185.7049497278729575, 38.27148437608393294, -9.295050272127046043 ) ) ;
#18306=EDGE_LOOP ( 'NONE', ( #28086, #4589, #11128, #11383 ) ) ;
#18307=CARTESIAN_POINT ( 'NONE',  ( 139.2950502721270425, 33.11210937608393579, 9.295050272127046043 ) ) ;
#18308=CARTESIAN_POINT ( 'NONE',  ( 55.70494972787295751, 31.72304687608393081, -9.295050272127046043 ) ) ;
#18310=CARTESIAN_POINT ( 'NONE',  ( 189.5550856135277229, 34.55078125108393294, 13.14518615778179722 ) ) ;
#18315=CARTESIAN_POINT ( 'NONE',  ( 143.5748159460630688, 39.11484375216787157, -1.662435489736055892E-15 ) ) ;
#18319=CARTESIAN_POINT ( 'NONE',  ( 65.32860027656705881, 53.49358765998906762, 14.99999999999997868 ) ) ;
#18322=ORIENTED_EDGE ( 'NONE', *, *, #4456, .F. ) ;
#18325=ORIENTED_EDGE ( 'NONE', *, *, #19766, .T. ) ;
#18329=CARTESIAN_POINT ( 'NONE',  ( 189.3771271284222166, 40.15664062716787441, -13.57481594606315412 ) ) ;
#18330=CARTESIAN_POINT ( 'NONE',  ( 74.29505027212704249, 33.11210937608393579, 9.295050272127046043 ) ) ;
#18333=CARTESIAN_POINT ( 'NONE',  ( -13.57481594606304398, 38.66835937499999432, 5.622872871577880183 ) ) ;
#18335=CARTESIAN_POINT ( 'NONE',  ( 5.323790963956049893, 54.47170356488337006, 14.99999999999999645 ) ) ;
#18336=FACE_OUTER_BOUND ( 'NONE', #25164, .T. ) ;
#18337=CARTESIAN_POINT ( 'NONE',  ( 116.4251840539369596, 34.69960937499999432, 5.622872871577880183 ) ) ;
#18339=VERTEX_POINT ( 'NONE', #23857 ) ;
#18344=CARTESIAN_POINT ( 'NONE',  ( 143.1451861577818079, 34.55078125108393294, 5.444914386472293977 ) ) ;
#18346=CARTESIAN_POINT ( 'NONE',  ( 59.37712712842213136, 32.21914062716787441, -13.57481594606304753 ) ) ;
#18347=CARTESIAN_POINT ( 'NONE',  ( 13.14518615778179900, 39.41250000108393436, -5.444914386472297529 ) ) ;
#18349=LINE ( 'NONE', #16200, #5352 ) ;
#18351=CARTESIAN_POINT ( 'NONE',  ( 99.99999999999995737, 82.37500000273119838, 4.999999999999990230 ) ) ;
#18354=AXIS2_PLACEMENT_3D ( 'NONE', #14031, #11750, #22756 ) ;
#18356=CARTESIAN_POINT ( 'NONE',  ( 189.3771271284219608, 39.56132812500000284, 13.57481594606290720 ) ) ;
#18366=CARTESIAN_POINT ( 'NONE',  ( 95.54126587499995082, 84.37500000136562051, -1.846868145590750077 ) ) ;
#18367=CARTESIAN_POINT ( 'NONE',  ( 78.14518615778179367, 33.85625000108393579, -5.444914386472297529 ) ) ;
#18370=CARTESIAN_POINT ( 'NONE',  ( 195.0000000000000000, 40.80156249999999574, -13.57481594606304576 ) ) ;
#18371=CARTESIAN_POINT ( 'NONE',  ( 130.0000000000000000, 37.72578125216787726, -13.57481594606304576 ) ) ;
#18372=CARTESIAN_POINT ( 'NONE',  ( -9.598844408820458085, 32.16953124999999147, -9.598844408820458085 ) ) ;
#18374=CARTESIAN_POINT ( 'NONE',  ( 130.0000000000000000, 33.01289062608393721, 13.14518615778179544 ) ) ;
#18376=CARTESIAN_POINT ( 'NONE',  ( 94.99999999999995737, 81.06250000000000000, 2.071067811865466624 ) ) ;
#18378=CARTESIAN_POINT ( 'NONE',  ( 103.1528011352953342, 83.81250000136560629, 3.152801135295355106 ) ) ;
#18380=CARTESIAN_POINT ( 'NONE',  ( 120.4011555911795455, 38.51953124999999289, -9.598844408820458085 ) ) ;
#18384=CARTESIAN_POINT ( 'NONE',  ( 185.7049497278729575, 32.71523437608393436, 9.295050272127047819 ) ) ;
#18385=CARTESIAN_POINT ( 'NONE',  ( 5.622872871577878406, 37.37851562716787157, 13.57481594606304576 ) ) ;
#18388=ORIENTED_EDGE ( 'NONE', *, *, #7194, .T. ) ;
#18390=CARTESIAN_POINT ( 'NONE',  ( 185.7049497278729575, 40.45429687608393721, -9.295050272127046043 ) ) ;
#18394=CARTESIAN_POINT ( 'NONE',  ( 124.5550856135277087, 40.40468750108393436, -13.14518615778179722 ) ) ;
#18395=CARTESIAN_POINT ( 'NONE',  ( -9.295050272127046043, 31.92148437608393508, -9.295050272127046043 ) ) ;
#18396=CARTESIAN_POINT ( 'NONE',  ( 116.8548138422182063, 32.66562500108393863, 5.444914386472304635 ) ) ;
#18397=CARTESIAN_POINT ( 'NONE',  ( 78.57481594606304043, 32.71523437500000142, -5.622872871577873077 ) ) ;
#18399=EDGE_CURVE ( 'NONE', #15569, #13131, #157, .T. ) ;
#18401=CARTESIAN_POINT ( 'NONE',  ( 99.99999999999995737, 85.00000000000000000, -5.000000000000018652 ) ) ;
#18409=CARTESIAN_POINT ( 'NONE',  ( -9.295050272127046043, 33.50898437608393010, -9.295050272127046043 ) ) ;
#18411=ORIENTED_EDGE ( 'NONE', *, *, #7391, .F. ) ;
#18412=CARTESIAN_POINT ( 'NONE',  ( 120.8198241863519797, 55.00000000000014211, -10.00000000000000000 ) ) ;
#18413=CYLINDRICAL_SURFACE ( 'NONE', #6112, 5.000000000000000000 ) ;
#18414=DIRECTION ( 'NONE',  ( 0.000000000000000000, 0.000000000000000000, -1.000000000000000000 ) ) ;
#18415=EDGE_CURVE ( 'NONE', #6416, #13933, #8491, .T. ) ;
#18416=CARTESIAN_POINT ( 'NONE',  ( 200.4449143864723055, 36.33671875108394289, -13.14518615778179900 ) ) ;
#18418=CARTESIAN_POINT ( 'NONE',  ( 200.3654965680425732, 54.48174559707338460, -15.00000000000000355 ) ) ;
#18423=CARTESIAN_POINT ( 'NONE',  ( 200.6228728715778686, 40.05742187716786873, -13.57481594606304753 ) ) ;
#18425=CARTESIAN_POINT ( 'NONE',  ( 143.1451861577818079, 37.82500000108392868, -5.444914386472297529 ) ) ;
#18426=CARTESIAN_POINT ( 'NONE',  ( 13.14518615778179722, 36.33671875108393579, 5.444914386472293977 ) ) ;
#18427=CARTESIAN_POINT ( 'NONE',  ( 3.755639919285892248, 31.58960996655074993, -13.14518615778179544 ) ) ;
#18432=VERTEX_POINT ( 'NONE', #14690 ) ;
#18437=CARTESIAN_POINT ( 'NONE',  ( 74.29505027212704249, 36.08867187608392868, 9.295050272127046043 ) ) ;
#18438=CARTESIAN_POINT ( 'NONE',  ( -9.598844408820454532, 38.81718750216787583, 9.598844408820459861 ) ) ;
#18439=EDGE_CURVE ( 'NONE', #144, #13739, #22556, .T. ) ;
#18440=B_SPLINE_CURVE_WITH_KNOTS ( 'NONE', 3,
 ( #410, #17360, #8949, #17215, #17640, #23779, #8668, #25920, #9094, #15347, #17788, #6394, #24062, #6806, #13201, #19640, #26491, #21935 ),
 .UNSPECIFIED., .F., .F.,
 ( 4, 2, 2, 2, 2, 2, 2, 2, 4 ),
 ( 0.000000000000000000, 0.004618502246277245149, 0.006927753369415865989, 0.009237004492554486829, 0.01039163005412375301, 0.01154625561569302093, 0.01385550673883156371, 0.01616475786197010128, 0.01847400898510864406 ),
 .UNSPECIFIED. ) ;
#18442=CARTESIAN_POINT ( 'NONE',  ( 204.1801758136480203, 50.00000000000000000, 9.999999999999946709 ) ) ;
#18449=VECTOR ( 'NONE', #20597, 1000.000000000000000 ) ;
#18452=ORIENTED_EDGE ( 'NONE', *, *, #14367, .F. ) ;
#18457=CARTESIAN_POINT ( 'NONE',  ( 195.0000000000000000, 35.39414062608393863, 13.14518615778179544 ) ) ;
#18458=ORIENTED_EDGE ( 'NONE', *, *, #12606, .F. ) ;
#18460=CARTESIAN_POINT ( 'NONE',  ( 8.211314015175984693, 50.68678854790367438, -14.99999999999861799 ) ) ;
#18461=CARTESIAN_POINT ( 'NONE',  ( 191.8834079195341928, 53.90895096933309816, 14.99999999999995026 ) ) ;
#18462=CARTESIAN_POINT ( 'NONE',  ( 130.0000000000000000, 39.31328125216787583, -13.57481594606304576 ) ) ;
#18463=CARTESIAN_POINT ( 'NONE',  ( 65.00000000000000000, 36.00000000000000000, -7.517135062566165128E-15 ) ) ;
#18465=CARTESIAN_POINT ( 'NONE',  ( 73.39593874129975859, 54.99999999495008041, 14.99999999999997691 ) ) ;
#18472=CARTESIAN_POINT ( 'NONE',  ( 139.5988444088204687, 38.22187500216787015, 9.598844408820456309 ) ) ;
#18473=CARTESIAN_POINT ( 'NONE',  ( 74.29505027212704249, 33.31054687608394005, -9.295050272127046043 ) ) ;
#18474=LINE ( 'NONE', #11889, #10875 ) ;
#18476=CARTESIAN_POINT ( 'NONE',  ( 1.137167824540872951, 35.99999999999998579, 13.09590655363602707 ) ) ;
#18479=DIRECTION ( 'NONE',  ( 0.000000000000000000, 0.000000000000000000, 1.000000000000000000 ) ) ;
#18481=CARTESIAN_POINT ( 'NONE',  ( 143.5748159460630404, 35.79101562499999289, 5.622872871577869525 ) ) ;
#18482=ORIENTED_EDGE ( 'NONE', *, *, #440, .F. ) ;
#18483=CARTESIAN_POINT ( 'NONE',  ( 99.99999999999995737, 85.00000000000000000, -1.387778780781445676E-14 ) ) ;
#18487=CARTESIAN_POINT ( 'NONE',  ( 116.8548138422182063, 38.32109375108394289, -5.444914386472297529 ) ) ;
#18488=CARTESIAN_POINT ( 'NONE',  ( 78.57481594606304043, 32.02070312716787015, -5.622872871577873077 ) ) ;
#18492=CARTESIAN_POINT ( 'NONE',  ( 5.444914386472297529, 39.51171875108392584, -13.14518615778179900 ) ) ;
#18496=PLANE ( 'NONE',  #3904 ) ;
#18497=CARTESIAN_POINT ( 'NONE',  ( 65.00000000000000000, 36.00000000000000000, -11.57481594606305109 ) ) ;
#18498=VECTOR ( 'NONE', #21279, 1000.000000000000000 ) ;
#18503=DIRECTION ( 'NONE',  ( 0.000000000000000000, 0.000000000000000000, -1.000000000000000000 ) ) ;
#18510=CARTESIAN_POINT ( 'NONE',  ( 51.85481384221819923, 31.77265625108393365, -5.444914386472297529 ) ) ;
#18516=CARTESIAN_POINT ( 'NONE',  ( -5.622872871577873077, 33.70742187500000142, -13.57481594606304753 ) ) ;
#18518=CARTESIAN_POINT ( 'NONE',  ( 143.1451861577818079, 33.95546875108393436, 5.444914386472293977 ) ) ;
#18519=ORIENTED_EDGE ( 'NONE', *, *, #17489, .T. ) ;
#18521=CARTESIAN_POINT ( 'NONE',  ( 195.0000000000000000, 36.43593749999999432, 13.57481594606304576 ) ) ;
#18522=CARTESIAN_POINT ( 'NONE',  ( 101.8468681455906903, 81.75000000136560629, 4.458734124999987891 ) ) ;
#18523=AXIS2_PLACEMENT_3D ( 'NONE', #21356, #10216, #6375 ) ;
#18525=CARTESIAN_POINT ( 'NONE',  ( 116.4251840539369596, 38.61874999999999147, 0.000000000000000000 ) ) ;
#18527=CARTESIAN_POINT ( 'NONE',  ( 208.1451861577817795, 39.51171875108392584, 5.444914386472293977 ) ) ;
#18528=CARTESIAN_POINT ( 'NONE',  ( 13.57481594606304931, 39.06523437716786873, 5.622872871577869525 ) ) ;
#18531=ORIENTED_EDGE ( 'NONE', *, *, #8798, .F. ) ;
#18533=CARTESIAN_POINT ( 'NONE',  ( 189.3771271284221314, 32.51679687716787726, 13.57481594606304753 ) ) ;
#18538=CARTESIAN_POINT ( 'NONE',  ( 97.92893218813445344, 80.31250000273119838, 4.999999999999948486 ) ) ;
#18540=CARTESIAN_POINT ( 'NONE',  ( 74.59884440882045453, 32.56640625000000000, 9.598844408820456309 ) ) ;
#18543=CARTESIAN_POINT ( 'NONE',  ( 116.9416181435491211, 36.00000000000000711, 1.569311539113940501 ) ) ;
#18551=CARTESIAN_POINT ( 'NONE',  ( -5.444914386472297529, 34.25312500108393010, -13.14518615778179900 ) ) ;
#18553=DIRECTION ( 'NONE',  ( -0.000000000000000000, 1.000000000000000000, -0.000000000000000000 ) ) ;
#18555=AXIS2_PLACEMENT_3D ( 'NONE', #15022, #23742, #8065 ) ;
#18556=CARTESIAN_POINT ( 'NONE',  ( -5.622872871577873966, 37.67617187499999432, -13.57481594606304753 ) ) ;
#18557=CARTESIAN_POINT ( 'NONE',  ( 208.1451861577818079, 33.01289062608393010, -1.609821015232357215E-15 ) ) ;
#18558=EDGE_LOOP ( 'NONE', ( #24091, #20193, #17722, #28132 ) ) ;
#18559=( BOUNDED_CURVE ( )  B_SPLINE_CURVE ( 2, ( #22091, #14085, #20525, #22945, #22805, #3273, #3406, #11942, #7246 ),
 .UNSPECIFIED., .F., .F. ) 
 B_SPLINE_CURVE_WITH_KNOTS ( ( 3, 2, 2, 2, 3 ),
 ( 0.3541666666666666852, 0.3645833333333332593, 0.3749999999999998890, 0.3854166666666665741, 0.3958333333333331483 ),
 .UNSPECIFIED. ) 
 CURVE ( )  GEOMETRIC_REPRESENTATION_ITEM ( )  RATIONAL_B_SPLINE_CURVE ( ( 1.000000000000000000, 0.9238795325112867385, 1.000000000000000000, 0.9238795325112867385, 1.000000000000000000, 0.9238795325112867385, 1.000000000000000000, 0.9238795325112879597, 0.9999999999999987788 ) ) 
 REPRESENTATION_ITEM ( '' )  );
#18561=CARTESIAN_POINT ( 'NONE',  ( 197.1699565831061420, 49.99999999883939950, -13.43548448457871558 ) ) ;
#18567=CARTESIAN_POINT ( 'NONE',  ( 185.4011555911795313, 40.20625000216787726, -9.598844408820458085 ) ) ;
#18568=DIRECTION ( 'NONE',  ( 0.000000000000000000, 0.000000000000000000, 1.000000000000000000 ) ) ;
#18570=CARTESIAN_POINT ( 'NONE',  ( 5.444914386472302859, 36.23750000108393721, 13.14518615778179189 ) ) ;
#18571=CARTESIAN_POINT ( 'NONE',  ( 5.444914386472297529, 33.16171875108393152, -13.14518615778179900 ) ) ;
#18574=EDGE_CURVE ( 'NONE', #15719, #25242, #21712, .T. ) ;
#18575=CARTESIAN_POINT ( 'NONE',  ( -5.622872871577965448, 37.27929687716785878, 13.57481594606295161 ) ) ;
#18578=CARTESIAN_POINT ( 'NONE',  ( 103.1528011352953342, 84.06250000136560629, 3.152801135295355106 ) ) ;
#18586=EDGE_CURVE ( 'NONE', #18339, #20261, #9156, .T. ) ;
#18589=VERTEX_POINT ( 'NONE', #26249 ) ;
#18590=CARTESIAN_POINT ( 'NONE',  ( 195.0000000000000000, 37.32890625216786873, 13.57481594606304576 ) ) ;
#18591=CARTESIAN_POINT ( 'NONE',  ( 74.29505027212704249, 37.87460937608393863, 9.295050272127046043 ) ) ;
#18593=AXIS2_PLACEMENT_3D ( 'NONE', #24494, #4839, #7233 ) ;
#18594=CARTESIAN_POINT ( 'NONE',  ( 198.7556399192858976, 31.78804746655075419, -13.14518615778179544 ) ) ;
#18595=VERTEX_POINT ( 'NONE', #6709 ) ;
#18597=EDGE_CURVE ( 'NONE', #3340, #3050, #1198, .T. ) ;
#18598=CARTESIAN_POINT ( 'NONE',  ( 3.114697745540293106, 53.90847045361019241, -15.00000000000000000 ) ) ;
#18600=CARTESIAN_POINT ( 'NONE',  ( 202.6165253254807794, 54.91574374957784954, 14.99999999999994493 ) ) ;
#18602=CARTESIAN_POINT ( 'NONE',  ( 116.4251840539369596, 36.38632812716788578, 5.622872871577880183 ) ) ;
#18605=CARTESIAN_POINT ( 'NONE',  ( 208.1451861577818079, 37.18007812608393436, -1.609821015232357215E-15 ) ) ;
#18606=ORIENTED_EDGE ( 'NONE', *, *, #5162, .F. ) ;
#18611=CARTESIAN_POINT ( 'NONE',  ( 99.99999999999995737, 83.68750000136560629, 4.458734124999988779 ) ) ;
#18612=DIRECTION ( 'NONE',  ( -1.000000000000000000, -0.000000000000000000, -0.000000000000000000 ) ) ;
#18614=CARTESIAN_POINT ( 'NONE',  ( -9.598844408820454532, 38.71796874999999716, 9.598844408820459861 ) ) ;
#18615=VECTOR ( 'NONE', #20956, 1000.000000000000000 ) ;
#18618=CARTESIAN_POINT ( 'NONE',  ( 130.0000000000000000, 34.45156249999999432, -13.57481594606304576 ) ) ;
#18619=ORIENTED_EDGE ( 'NONE', *, *, #16850, .T. ) ;
#18624=APPLICATION_CONTEXT ( 'automotive_design' ) ;
#18626=CARTESIAN_POINT ( 'NONE',  ( 143.1451861577818079, 40.30546875108393579, 5.444914386472293977 ) ) ;
#18627=CARTESIAN_POINT ( 'NONE',  ( 51.85481384221819923, 39.71015625108393010, -5.444914386472297529 ) ) ;
#18628=EDGE_CURVE ( 'NONE', #26813, #7460, #7973, .T. ) ;
#18629=CARTESIAN_POINT ( 'NONE',  ( 59.43094144809686696, 36.00000000000000000, 11.91493531101255954 ) ) ;
#18630=CARTESIAN_POINT ( 'NONE',  ( -5.444914386472299306, 38.32109375108394289, 13.14518615778179722 ) ) ;
#18635=CARTESIAN_POINT ( 'NONE',  ( 99.99999999999995737, 82.87500000273119838, -5.000000000000018652 ) ) ;
#18639=CARTESIAN_POINT ( 'NONE',  ( 130.3745404134768648, 36.00000000000000000, -13.51869779562199447 ) ) ;
#18640=CARTESIAN_POINT ( 'NONE',  ( 195.0000000000000000, 39.71015625216787015, 13.57481594606304576 ) ) ;
#18650=CARTESIAN_POINT ( 'NONE',  ( 95.54126587499995082, 82.50000000136560629, 1.846868145590724986 ) ) ;
#18651=CARTESIAN_POINT ( 'NONE',  ( 51.85481384221819923, 40.70234375108393721, -5.444914386472297529 ) ) ;
#18656=CARTESIAN_POINT ( 'NONE',  ( -15.00000000000000355, 75.00000000000000000, -14.99999999999999822 ) ) ;
#18658=CARTESIAN_POINT ( 'NONE',  ( 139.2950502721270425, 35.49335937608393721, 9.295050272127046043 ) ) ;
#18660=CARTESIAN_POINT ( 'NONE',  ( 2.493653234604083739E-15, 38.91640625216786731, 13.57481594606304576 ) ) ;
#18661=CARTESIAN_POINT ( 'NONE',  ( 70.62287287157793969, 38.46992187716787726, -13.57481594606299247 ) ) ;
#18662=CARTESIAN_POINT ( 'NONE',  ( 101.8468681455906903, 83.75000000136560629, 4.458734124999987891 ) ) ;
#18663=CARTESIAN_POINT ( 'NONE',  ( 130.0000000000000000, 38.76757812608393294, -13.14518615778179544 ) ) ;
#18665=CARTESIAN_POINT ( 'NONE',  ( 208.5748159460630688, 37.47773437500001137, -5.622872871577873966 ) ) ;
#18667=CARTESIAN_POINT ( 'NONE',  ( -13.57481594606304753, 37.87460937716787868, -5.622872871577873077 ) ) ;
#18668=VERTEX_POINT ( 'NONE', #11830 ) ;
#18669=CIRCLE ( 'NONE', #24580, 13.57481594606304398 ) ;
#18671=ORIENTED_EDGE ( 'NONE', *, *, #6192, .F. ) ;
#18672=CARTESIAN_POINT ( 'NONE',  ( 12.07727640983618400, 35.99999999999999289, -6.197985357348143154 ) ) ;
#18673=CARTESIAN_POINT ( 'NONE',  ( 181.4251840539369596, 31.57421875216786944, 0.000000000000000000 ) ) ;
#18676=CARTESIAN_POINT ( 'NONE',  ( 139.2950502721270425, 38.66835937608393436, -9.295050272127046043 ) ) ;
#18677=CARTESIAN_POINT ( 'NONE',  ( 99.99999999999995737, 80.37500000273119838, 4.999999999999990230 ) ) ;
#18678=LINE ( 'NONE', #12228, #19977 ) ;
#18681=CARTESIAN_POINT ( 'NONE',  ( 181.4251840539369596, 40.99999999999999289, 0.000000000000000000 ) ) ;
#18688=CARTESIAN_POINT ( 'NONE',  ( 74.18017581364799184, 55.00000000000000000, -14.99999999999999822 ) ) ;
#18690=CARTESIAN_POINT ( 'NONE',  ( -8.049105076161786076E-16, 32.61601562608393579, -13.14518615778179544 ) ) ;
#18691=ORIENTED_EDGE ( 'NONE', *, *, #17865, .T. ) ;
#18692=CARTESIAN_POINT ( 'NONE',  ( 98.15313185440925281, 81.87500000136559208, 4.458734124999987891 ) ) ;
#18694=CARTESIAN_POINT ( 'NONE',  ( 208.1451861577817795, 33.85625000108393579, -5.444914386472297529 ) ) ;
#18695=EDGE_LOOP ( 'NONE', ( #974, #19924, #27770, #5728 ) ) ;
#18696=CARTESIAN_POINT ( 'NONE',  ( 191.0201855541805855, 50.00000000123257848, -13.01613927312581787 ) ) ;
#18701=CARTESIAN_POINT ( 'NONE',  ( 189.3771271284221598, 38.56914062716787583, -13.57481594606310260 ) ) ;
#18703=CARTESIAN_POINT ( 'NONE',  ( -8.049105076161786076E-16, 37.37851562608393863, -13.14518615778179544 ) ) ;
#18704=CARTESIAN_POINT ( 'NONE',  ( -9.295050272127046043, 33.31054687608393294, -9.295050272127046043 ) ) ;
#18707=CARTESIAN_POINT ( 'NONE',  ( -5.622872871577873966, 36.98164062716787015, -13.57481594606304753 ) ) ;
#18711=EDGE_CURVE ( 'NONE', #24077, #19327, #7542, .T. ) ;
#18712=CARTESIAN_POINT ( 'NONE',  ( 99.99999999999995737, 82.93750000136560629, 4.458734124999988779 ) ) ;
#18716=CARTESIAN_POINT ( 'NONE',  ( 65.71976059610913978, 53.51499872091922327, 14.99999999999997513 ) ) ;
#18717=ORIENTED_EDGE ( 'NONE', *, *, #10096, .F. ) ;
#18724=CARTESIAN_POINT ( 'NONE',  ( 124.3771271284220745, 39.36289062716787157, -13.57481594606297293 ) ) ;
#18727=CARTESIAN_POINT ( 'NONE',  ( 70.44491438647229131, 37.03125000108393294, 13.14518615778179189 ) ) ;
#18729=ADVANCED_FACE ( 'NONE', ( #893 ), #11683, .T. ) ;
#18730=CARTESIAN_POINT ( 'NONE',  ( 94.99999999999995737, 85.00000000000000000, -1.387778780781445676E-14 ) ) ;
#18734=CARTESIAN_POINT ( 'NONE',  ( 135.6228728715778686, 36.88242187716787157, -13.57481594606304753 ) ) ;
#18735=CARTESIAN_POINT ( 'NONE',  ( 139.5988444088204687, 37.42812500216787441, 9.598844408820456309 ) ) ;
#18739=CARTESIAN_POINT ( 'NONE',  ( 185.7049497278729575, 36.88242187608393152, 9.295050272127047819 ) ) ;
#18740=ADVANCED_FACE ( 'NONE', ( #6851 ), #5019, .T. ) ;
#18744=CARTESIAN_POINT ( 'NONE',  ( 116.6399989480775901, 40.87597656304196647, 0.000000000000000000 ) ) ;
#18746=CARTESIAN_POINT ( 'NONE',  ( 96.84719886470459471, 83.31250000136560629, -3.152801135295383084 ) ) ;
#18748=( NAMED_UNIT ( * ) SI_UNIT ( $, .STERADIAN. ) SOLID_ANGLE_UNIT ( ) );
#18750=CARTESIAN_POINT ( 'NONE',  ( 94.99999999999995737, 81.06250000000001421, 2.071067811865466624 ) ) ;
#18751=FACE_OUTER_BOUND ( 'NONE', #14553, .T. ) ;
#18754=ORIENTED_EDGE ( 'NONE', *, *, #17301, .T. ) ;
#18760=CARTESIAN_POINT ( 'NONE',  ( 130.0000000000000000, 40.55351562608393579, -13.14518615778179544 ) ) ;
#18761=CARTESIAN_POINT ( 'NONE',  ( 74.29505027212704249, 37.08085937608393579, -9.295050272127046043 ) ) ;
#18762=( BOUNDED_SURFACE ( )  B_SPLINE_SURFACE ( 3, 2, ( 
 ( #26756, #5228, #11471 ),
 ( #13893, #13611, #3089 ),
 ( #22619, #7198, #20333 ),
 ( #11756, #22188, #24464 ),
 ( #5372, #18041, #5513 ),
 ( #820, #7345, #675 ),
 ( #14039, #1103, #5088 ),
 ( #9488, #20481, #15758 ),
 ( #20618, #16036, #9770 ),
 ( #2939, #15893, #24748 ),
 ( #22334, #7489, #25030 ),
 ( #7637, #24610, #3227 ),
 ( #11610, #27042, #7061 ),
 ( #961, #20051, #16185 ),
 ( #9630, #16332, #24891 ),
 ( #11894, #2668, #18335 ),
 ( #17904, #11329, #529 ),
 ( #9210, #26614, #4947 ),
 ( #17013, #20756, #23036 ),
 ( #14180, #16466, #19017 ) ),
 .UNSPECIFIED., .F., .F., .F. ) 
 B_SPLINE_SURFACE_WITH_KNOTS ( ( 4, 2, 2, 2, 2, 2, 2, 2, 2, 4 ),
 ( 3, 3 ),
 ( 0.009073803551359458167, 0.01139250602759181441, 0.01371120850382416892, 0.01602991098005652343, 0.01834861345628887794, 0.01950796469440505693, 0.02066731593252123245, 0.02298601840875359043, 0.02530472088498594493, 0.02762342336121829944 ),
 ( 0.000000000000000000, 1.000000000000000000 ),
 .UNSPECIFIED. ) 
 GEOMETRIC_REPRESENTATION_ITEM ( )  RATIONAL_B_SPLINE_SURFACE ( (
 ( 1.000000000000000000, 0.7071067811865470176, 1.000000000000000000),
 ( 1.000000000000000000, 0.7344871497829198459, 1.000000000000000000),
 ( 1.000000000000000000, 0.7612510203318438862, 1.000000000000000000),
 ( 1.000000000000000000, 0.8116663633844432013, 1.000000000000000000),
 ( 1.000000000000000000, 0.8353358059752060694, 1.000000000000000000),
 ( 1.000000000000000000, 0.8764699612585808985, 1.000000000000000000),
 ( 1.000000000000000000, 0.8939017358719159034, 1.000000000000000000),
 ( 1.000000000000000000, 0.9185314935647115320, 1.000000000000000000),
 ( 1.000000000000000000, 0.9256439951239472386, 1.000000000000000000),
 ( 1.000000000000000000, 0.9261623622476506945, 1.000000000000000000),
 ( 1.000000000000000000, 0.9246301385979278642, 1.000000000000000000),
 ( 1.000000000000000000, 0.9183304321347580679, 1.000000000000000000),
 ( 1.000000000000000000, 0.9135987334168627072, 1.000000000000000000),
 ( 1.000000000000000000, 0.8954110486039240646, 1.000000000000000000),
 ( 1.000000000000000000, 0.8779877431164836432, 1.000000000000000000),
 ( 1.000000000000000000, 0.8366182664708666783, 1.000000000000000000),
 ( 1.000000000000000000, 0.8126941604017877685, 1.000000000000000000),
 ( 1.000000000000000000, 0.7617527316303357443, 1.000000000000000000),
 ( 1.000000000000000000, 0.7347103785793935860, 1.000000000000000000),
 ( 1.000000000000000000, 0.7071067811865462405, 1.000000000000000000) ) ) 
 REPRESENTATION_ITEM ( '' )  SURFACE ( )  );
#18763=DIRECTION ( 'NONE',  ( 0.000000000000000000, 0.000000000000000000, -1.000000000000000000 ) ) ;
#18764=CARTESIAN_POINT ( 'NONE',  ( 5.444914386472297529, 36.33671875108394289, -13.14518615778179900 ) ) ;
#18767=CARTESIAN_POINT ( 'NONE',  ( 94.99999999999995737, 82.06250000000001421, 2.071067811865466624 ) ) ;
#18770=CARTESIAN_POINT ( 'NONE',  ( 181.6399989480775901, 40.42949218912590936, 0.000000000000000000 ) ) ;
#18777=ORIENTED_EDGE ( 'NONE', *, *, #6047, .T. ) ;
#18778=CYLINDRICAL_SURFACE ( 'NONE', #9333, 13.57481594606304398 ) ;
#18782=CARTESIAN_POINT ( 'NONE',  ( 94.99999999999995737, 80.00000000000000000, -1.387778780781445676E-14 ) ) ;
#18783=CARTESIAN_POINT ( 'NONE',  ( 104.4587341249999639, 80.93750000136559208, -1.442382525525748735E-14 ) ) ;
#18784=CARTESIAN_POINT ( 'NONE',  ( 70.44491438647230552, 39.71015625108393010, -13.14518615778179900 ) ) ;
#18786=CARTESIAN_POINT ( 'NONE',  ( -13.36000105192242060, 40.42949218912590936, 0.000000000000000000 ) ) ;
#18790=CARTESIAN_POINT ( 'NONE',  ( 124.5550856135277087, 33.45937500108394147, -13.14518615778179900 ) ) ;
#18795=CARTESIAN_POINT ( 'NONE',  ( 139.2950502721270425, 38.46992187608393010, 9.295050272127046043 ) ) ;
#18796=CARTESIAN_POINT ( 'NONE',  ( 70.62287287157788285, 37.37851562716787157, 13.57481594606304576 ) ) ;
#18798=CARTESIAN_POINT ( 'NONE',  ( 13.57481594606304576, 39.11484375216787157, -1.662435489736055892E-15 ) ) ;
#18802=VERTEX_POINT ( 'NONE', #15687 ) ;
#18804=CARTESIAN_POINT ( 'NONE',  ( 208.5748159460630120, 32.71523437716787441, 5.622872871577869525 ) ) ;
#18807=CARTESIAN_POINT ( 'NONE',  ( 143.1451861577818079, 39.36289062608393152, -1.609821015232357215E-15 ) ) ;
#18808=CARTESIAN_POINT ( 'NONE',  ( 3.755639919285892248, 31.78804746655075419, -13.14518615778179544 ) ) ;
#18812=CARTESIAN_POINT ( 'NONE',  ( 189.3771271284221314, 37.97382812499999716, 13.57481594606304753 ) ) ;
#18816=CARTESIAN_POINT ( 'NONE',  ( 185.4011555911795313, 36.93203124999999432, -9.598844408820458085 ) ) ;
#18820=CARTESIAN_POINT ( 'NONE',  ( 208.5748159460630688, 39.75976562499999289, 5.622872871577868636 ) ) ;
#18822=CARTESIAN_POINT ( 'NONE',  ( 13.57481594606304931, 40.55351562499998863, 5.622872871577869525 ) ) ;
#18823=VERTEX_POINT ( 'NONE', #22263 ) ;
#18824=CARTESIAN_POINT ( 'NONE',  ( 104.4587341249999781, 81.25000000136560629, -1.846868145590750299 ) ) ;
#18825=DIRECTION ( 'NONE',  ( -0.000000000000000000, 1.000000000000000000, -0.000000000000000000 ) ) ;
#18828=CARTESIAN_POINT ( 'NONE',  ( 196.9473259220809780, 51.47162402671693116, -15.00000000000000178 ) ) ;
#18834=CARTESIAN_POINT ( 'NONE',  ( 204.5988444088204403, 40.00781250216787299, -9.598844408820458085 ) ) ;
#18837=CARTESIAN_POINT ( 'NONE',  ( 139.2950502721270425, 38.86679687608393863, -9.295050272127046043 ) ) ;
#18838=CARTESIAN_POINT ( 'NONE',  ( -9.295050272127044266, 40.05742187608393579, 9.295050272127047819 ) ) ;
#18839=ORIENTED_EDGE ( 'NONE', *, *, #7861, .T. ) ;
#18840=CARTESIAN_POINT ( 'NONE',  ( 70.62287287157786864, 39.16445312499999432, -13.57481594606304753 ) ) ;
#18841=CARTESIAN_POINT ( 'NONE',  ( 65.00000000000000000, 39.71015625216787015, 13.57481594606304576 ) ) ;
#18845=CARTESIAN_POINT ( 'NONE',  ( 104.4587341249999781, 82.12500000136560629, 1.846868145590721655 ) ) ;
#18847=CARTESIAN_POINT ( 'NONE',  ( -13.14518615778179900, 39.90859375108394147, -5.444914386472297529 ) ) ;
#18848=CARTESIAN_POINT ( 'NONE',  ( 63.39472812342341967, 53.60388944777321285, 14.99999999999998224 ) ) ;
#18849=ORIENTED_EDGE ( 'NONE', *, *, #160, .T. ) ;
#18856=EDGE_LOOP ( 'NONE', ( #17620, #23852, #11317, #4055, #18619, #24288, #21714, #27939, #25571, #27997, #27454, #6312, #27916, #15761, #4274, #10945, #28112 ) ) ;
#18857=CARTESIAN_POINT ( 'NONE',  ( 51.85481384221821344, 37.62656250108393152, 5.444914386472304635 ) ) ;
#18858=LINE ( 'NONE', #25423, #7790 ) ;
#18859=DIRECTION ( 'NONE',  ( 1.000000000000000000, 0.000000000000000000, -0.000000000000000000 ) ) ;
#18862=VECTOR ( 'NONE', #11977, 1000.000000000000000 ) ;
#18863=CARTESIAN_POINT ( 'NONE',  ( -8.754898953240607185, 50.00000000000000000, -10.39041163856195027 ) ) ;
#18864=CARTESIAN_POINT ( 'NONE',  ( 135.6228728715778686, 35.29492187716788720, -13.57481594606304753 ) ) ;
#18866=( BOUNDED_CURVE ( )  B_SPLINE_CURVE ( 2, ( #3643, #28002, #25155, #14725, #23580, #21305, #27585, #1927, #19012 ),
 .UNSPECIFIED., .F., .T. ) 
 B_SPLINE_CURVE_WITH_KNOTS ( ( 3, 2, 2, 2, 3 ),
 ( 0.02083333333333358892, 0.03125000000000020123, 0.04166666666666681007, 0.05208333333333342585, 0.06250000000000004163 ),
 .UNSPECIFIED. ) 
 CURVE ( )  GEOMETRIC_REPRESENTATION_ITEM ( )  RATIONAL_B_SPLINE_CURVE ( ( 0.9999999999999981126, 0.9238795325112886259, 1.000000000000000000, 0.9238795325112867385, 1.000000000000000000, 0.9238795325112867385, 1.000000000000000000, 0.9238795325112864054, 1.000000000000000222 ) ) 
 REPRESENTATION_ITEM ( '' )  );
#18869=CARTESIAN_POINT ( 'NONE',  ( 208.1451861577818079, 36.38632812608393863, -1.609821015232357215E-15 ) ) ;
#18870=ORIENTED_EDGE ( 'NONE', *, *, #9309, .T. ) ;
#18875=CARTESIAN_POINT ( 'NONE',  ( 181.8548138422182205, 40.50390625108394005, -5.444914386472297529 ) ) ;
#18878=AXIS2_PLACEMENT_3D ( 'NONE', #363, #17172, #21747 ) ;
#18879=CARTESIAN_POINT ( 'NONE',  ( 1.685511649082866548, 35.99999999999997868, 13.05727741351675597 ) ) ;
#18881=CARTESIAN_POINT ( 'NONE',  ( 143.5748159460630404, 32.71523437500000142, -5.622872871577873077 ) ) ;
#18882=ORIENTED_EDGE ( 'NONE', *, *, #17489, .F. ) ;
#18887=CARTESIAN_POINT ( 'NONE',  ( 130.0000000000000000, 38.56914062608393579, 13.14518615778179544 ) ) ;
#18888=CARTESIAN_POINT ( 'NONE',  ( 74.29505027212704249, 37.67617187608393436, 9.295050272127046043 ) ) ;
#18890=DIRECTION ( 'NONE',  ( -0.000000000000000000, 1.000000000000000000, -0.000000000000000000 ) ) ;
#18891=CARTESIAN_POINT ( 'NONE',  ( 13.14518615778179900, 34.55078125108393294, 5.444914386472293977 ) ) ;
#18892=CARTESIAN_POINT ( 'NONE',  ( 192.1079374786958738, 36.00000000000001421, -13.15766692561456708 ) ) ;
#18896=DIRECTION ( 'NONE',  ( 0.000000000000000000, 0.000000000000000000, 1.000000000000000000 ) ) ;
#18897=CIRCLE ( 'NONE', #24359, 11.57481594606304398 ) ;
#18898=CARTESIAN_POINT ( 'NONE',  ( 99.99999999999995737, 85.00000000000000000, -1.387778780781445676E-14 ) ) ;
#18899=CARTESIAN_POINT ( 'NONE',  ( -5.444914386472299306, 38.32109375108394289, 13.14518615778179722 ) ) ;
#18900=CARTESIAN_POINT ( 'NONE',  ( 133.8295627579928748, 36.00000000000000000, 12.63428651647566170 ) ) ;
#18902=EDGE_CURVE ( 'NONE', #8752, #18933, #21645, .T. ) ;
#18905=CARTESIAN_POINT ( 'NONE',  ( -8.312177448680279460E-16, 37.72578125216787726, -13.57481594606304576 ) ) ;
#18909=ORIENTED_EDGE ( 'NONE', *, *, #10229, .T. ) ;
#18910=CARTESIAN_POINT ( 'NONE',  ( 130.0000000000000000, 40.80156249999999574, -13.57481594606304576 ) ) ;
#18913=EDGE_CURVE ( 'NONE', #5976, #12843, #26192, .T. ) ;
#18916=CARTESIAN_POINT ( 'NONE',  ( 104.4587341249999781, 81.87500000136559208, 1.846868145590721655 ) ) ;
#18917=CARTESIAN_POINT ( 'NONE',  ( 74.29505027212704249, 37.08085937608393579, 9.295050272127046043 ) ) ;
#18921=CARTESIAN_POINT ( 'NONE',  ( 65.00000000000000000, 38.91640625216786731, 13.57481594606304576 ) ) ;
#18923=CARTESIAN_POINT ( 'NONE',  ( 116.4251840539369454, 40.95039062499999005, -5.622872871577873077 ) ) ;
#18926=( BOUNDED_CURVE ( )  B_SPLINE_CURVE ( 2, ( #23164, #10592, #19300, #8184, #27999, #1508, #27443, #4195, #16876 ),
 .UNSPECIFIED., .F., .T. ) 
 B_SPLINE_CURVE_WITH_KNOTS ( ( 3, 2, 2, 2, 3 ),
 ( 0.1500000000000001332, 0.1750000000000001554, 0.2000000000000001776, 0.2250000000000001998, 0.2500000000000002220 ),
 .UNSPECIFIED. ) 
 CURVE ( )  GEOMETRIC_REPRESENTATION_ITEM ( )  RATIONAL_B_SPLINE_CURVE ( ( 0.9999999999999995559, 0.9238795325112871826, 1.000000000000000000, 0.9238795325112867385, 1.000000000000000000, 0.9238795325112867385, 1.000000000000000000, 0.9238795325112860723, 1.000000000000000666 ) ) 
 REPRESENTATION_ITEM ( '' )  );
#18928=CARTESIAN_POINT ( 'NONE',  ( 96.84719886470459471, 81.31250000136559208, -3.152801135295383084 ) ) ;
#18929=CARTESIAN_POINT ( 'NONE',  ( 120.7049497278729575, 39.85898437608393152, 9.295050272127047819 ) ) ;
#18930=CARTESIAN_POINT ( 'NONE',  ( 51.42518405393695957, 37.87460937716787868, -5.622872871577873077 ) ) ;
#18932=CARTESIAN_POINT ( 'NONE',  ( 13.57481594606304753, 35.98945312716787015, -5.622872871577873077 ) ) ;
#18933=VERTEX_POINT ( 'NONE', #5860 ) ;
#18937=CARTESIAN_POINT ( 'NONE',  ( 181.8548138422182205, 36.58476562608393579, 0.000000000000000000 ) ) ;
#18938=CARTESIAN_POINT ( 'NONE',  ( 13.57481594606304576, 36.73359375216787015, -1.662435489736055892E-15 ) ) ;
#18940=CARTESIAN_POINT ( 'NONE',  ( 116.8548138422182205, 38.91640625108393436, -5.444914386472297529 ) ) ;
#18941=CARTESIAN_POINT ( 'NONE',  ( 94.99999999999995737, 80.06250000273119838, -2.071067811865491493 ) ) ;
#18942=FACE_OUTER_BOUND ( 'NONE', #15746, .T. ) ;
#18943=DIRECTION ( 'NONE',  ( -0.000000000000000000, 1.000000000000000000, -0.000000000000000000 ) ) ;
#18946=CARTESIAN_POINT ( 'NONE',  ( 185.4011555911795313, 37.72578124999999005, -9.598844408820458085 ) ) ;
#18949=CARTESIAN_POINT ( 'NONE',  ( 59.55508561352770158, 39.61093750108393152, -13.14518615778179900 ) ) ;
#18955=CARTESIAN_POINT ( 'NONE',  ( 13.57481594606304576, 38.22187499999999716, -1.662435489736055892E-15 ) ) ;
#18956=PLANE ( 'NONE',  #15305 ) ;
#18958=CARTESIAN_POINT ( 'NONE',  ( 101.8468681455906903, 84.37500000136562051, -4.458734125000016313 ) ) ;
#18959=( BOUNDED_CURVE ( )  B_SPLINE_CURVE ( 2, ( #19569, #21296, #4326, #25986, #8311, #23571, #21152, #10585, #17142 ),
 .UNSPECIFIED., .F., .T. ) 
 B_SPLINE_CURVE_WITH_KNOTS ( ( 3, 2, 2, 2, 3 ),
 ( 0.4500000000000003997, 0.4750000000000003664, 0.5000000000000004441, 0.5250000000000004663, 0.5500000000000004885 ),
 .UNSPECIFIED. ) 
 CURVE ( )  GEOMETRIC_REPRESENTATION_ITEM ( )  RATIONAL_B_SPLINE_CURVE ( ( 0.9999999999999987788, 0.9238795325112879597, 1.000000000000000000, 0.9238795325112867385, 1.000000000000000000, 0.9238795325112867385, 1.000000000000000000, 0.9238795325112854062, 1.000000000000001332 ) ) 
 REPRESENTATION_ITEM ( '' )  );
#18961=ORIENTED_EDGE ( 'NONE', *, *, #25699, .T. ) ;
#18962=( BOUNDED_CURVE ( )  B_SPLINE_CURVE ( 2, ( #22924, #10334, #12054, #20780, #3384 ),
 .UNSPECIFIED., .F., .F. ) 
 B_SPLINE_CURVE_WITH_KNOTS ( ( 3, 2, 3 ),
 ( 0.000000000000000000, 0.01041666666666679446, 0.02083333333333358892 ),
 .UNSPECIFIED. ) 
 CURVE ( )  GEOMETRIC_REPRESENTATION_ITEM ( )  RATIONAL_B_SPLINE_CURVE ( ( 1.000000000000000000, 0.9238795325112867385, 1.000000000000000000, 0.9238795325112848511, 1.000000000000001776 ) ) 
 REPRESENTATION_ITEM ( '' )  );
#18970=CYLINDRICAL_SURFACE ( 'NONE', #21331, 11.57481594606304398 ) ;
#18974=CARTESIAN_POINT ( 'NONE',  ( 139.2950502721270425, 40.45429687608393721, -9.295050272127046043 ) ) ;
#18975=CARTESIAN_POINT ( 'NONE',  ( 9.295050272127047819, 33.70742187608393436, 9.295050272127046043 ) ) ;
#18977=CARTESIAN_POINT ( 'NONE',  ( 74.59884440882045453, 38.12265624999999858, 9.598844408820456309 ) ) ;
#18979=CARTESIAN_POINT ( 'NONE',  ( 204.0314404224550628, 36.00000000000000000, 9.765766397118353481 ) ) ;
#18983=CARTESIAN_POINT ( 'NONE',  ( 101.8468681455907046, 84.00000000136560629, 4.458734124999987891 ) ) ;
#18985=CARTESIAN_POINT ( 'NONE',  ( 9.295050272127047819, 39.46210937608393721, 9.295050272127046043 ) ) ;
#18986=CARTESIAN_POINT ( 'NONE',  ( 55.81982418635200816, 55.00000000000000000, 14.99999999999998401 ) ) ;
#18987=ORIENTED_EDGE ( 'NONE', *, *, #1899, .F. ) ;
#18992=CARTESIAN_POINT ( 'NONE',  ( 204.2950502721270425, 36.28710937608393294, 9.295050272127046043 ) ) ;
#18994=CARTESIAN_POINT ( 'NONE',  ( 120.4011555911795455, 39.41250000216787441, -9.598844408820458085 ) ) ;
#18996=CARTESIAN_POINT ( 'NONE',  ( 70.44491438647229131, 39.41250000108393436, 13.14518615778179189 ) ) ;
#18998=CARTESIAN_POINT ( 'NONE',  ( 208.1451861577818079, 32.41757812608393863, -1.609821015232357215E-15 ) ) ;
#18999=EDGE_LOOP ( 'NONE', ( #25833, #1593, #18531, #21393 ) ) ;
#19001=CARTESIAN_POINT ( 'NONE',  ( 143.5748159460630688, 36.73359375216787015, -1.662435489736055892E-15 ) ) ;
#19003=CARTESIAN_POINT ( 'NONE',  ( 124.3771271284221314, 35.39414062716787157, -13.57481594606304753 ) ) ;
#19004=CARTESIAN_POINT ( 'NONE',  ( 51.85481384221820633, 39.21406250108392300, 5.444914386472304635 ) ) ;
#19006=CARTESIAN_POINT ( 'NONE',  ( 189.5550856135277229, 38.22187500108393010, -13.14518615778179900 ) ) ;
#19007=VERTEX_POINT ( 'NONE', #14530 ) ;
#19008=VERTEX_POINT ( 'NONE', #18688 ) ;
#19012=CARTESIAN_POINT ( 'NONE',  ( 65.00000000000000000, 39.71015625216787015, 13.57481594606304576 ) ) ;
#19016=CARTESIAN_POINT ( 'NONE',  ( 12.07727640983618400, 35.99999999999999289, -6.197985357348143154 ) ) ;
#19017=CARTESIAN_POINT ( 'NONE',  ( 9.180175813648018490, 55.00000000000000711, 14.99999999999999289 ) ) ;
#19018=CARTESIAN_POINT ( 'NONE',  ( 116.4251840539369596, 32.26874999999999716, 0.000000000000000000 ) ) ;
#19019=AXIS2_PLACEMENT_3D ( 'NONE', #18483, #27190, #16335 ) ;
#19020=ORIENTED_EDGE ( 'NONE', *, *, #24118, .T. ) ;
#19025=CARTESIAN_POINT ( 'NONE',  ( 143.1451861577818079, 38.81718750108393579, -5.444914386472297529 ) ) ;
#19026=CARTESIAN_POINT ( 'NONE',  ( 74.29505027212704249, 38.46992187608393010, 9.295050272127046043 ) ) ;
#19027=CARTESIAN_POINT ( 'NONE',  ( 185.7049497278729575, 39.26367187608393294, 9.295050272127047819 ) ) ;
#19029=CARTESIAN_POINT ( 'NONE',  ( -8.049105076161786076E-16, 34.79882812608393294, -13.14518615778179544 ) ) ;
#19032=CARTESIAN_POINT ( 'NONE',  ( -15.00000000000000355, 55.00000000000000000, -14.99999999999999822 ) ) ;
#19033=CARTESIAN_POINT ( 'NONE',  ( 65.00000000000000000, -7.395377635281828788, -13.57481594606305109 ) ) ;
#19035=CARTESIAN_POINT ( 'NONE',  ( 9.295050272127047819, 37.67617187608393436, 9.295050272127046043 ) ) ;
#19036=CARTESIAN_POINT ( 'NONE',  ( 142.0095733385115864, 36.00000000000000000, 5.901833544881823990 ) ) ;
#19038=AXIS2_PLACEMENT_3D ( 'NONE', #9119, #6973, #15668 ) ;
#19042=CARTESIAN_POINT ( 'NONE',  ( -13.57481594606304576, 40.30546875216787583, 0.000000000000000000 ) ) ;
#19043=CIRCLE ( 'NONE', #6755, 5.000000000000000888 ) ;
#19051=CARTESIAN_POINT ( 'NONE',  ( 189.3771271284222735, 36.18789062716787441, -13.57481594606318254 ) ) ;
#19052=CARTESIAN_POINT ( 'NONE',  ( 101.8468681455906903, 81.12500000136559208, -4.458734125000016313 ) ) ;
#19053=CARTESIAN_POINT ( 'NONE',  ( 74.29505027212704249, 38.66835937608393436, 9.295050272127046043 ) ) ;
#19055=CARTESIAN_POINT ( 'NONE',  ( -5.444914386472297529, 40.40468750108393436, -13.14518615778179722 ) ) ;
#19056=ORIENTED_EDGE ( 'NONE', *, *, #18628, .T. ) ;
#19059=CARTESIAN_POINT ( 'NONE',  ( 130.0000000000000000, 39.21406249999999716, -13.57481594606304576 ) ) ;
#19061=CARTESIAN_POINT ( 'NONE',  ( 139.5988444088204403, 39.11484374999999858, -9.598844408820458085 ) ) ;
#19063=EDGE_CURVE ( 'NONE', #25247, #10395, #3819, .T. ) ;
#19065=CARTESIAN_POINT ( 'NONE',  ( 95.54126587499995082, 80.50000000136560629, 1.846868145590724986 ) ) ;
#19066=FACE_OUTER_BOUND ( 'NONE', #16334, .T. ) ;
#19067=CARTESIAN_POINT ( 'NONE',  ( 78.57481594606305464, 38.32109375216786873, -1.662435489736055892E-15 ) ) ;
#19071=CARTESIAN_POINT ( 'NONE',  ( -8.312177448680279460E-16, 36.13828125216787157, -13.57481594606304576 ) ) ;
#19072=ORIENTED_EDGE ( 'NONE', *, *, #22375, .T. ) ;
#19073=CIRCLE ( 'NONE', #3177, 5.000000000000000000 ) ;
#19077=CARTESIAN_POINT ( 'NONE',  ( 189.5550856135277229, 38.32109375108394289, 13.14518615778179722 ) ) ;
#19079=CARTESIAN_POINT ( 'NONE',  ( 116.8548138422182205, 36.53515625108393294, -5.444914386472297529 ) ) ;
#19080=CARTESIAN_POINT ( 'NONE',  ( 130.0000000000000000, 52.00000000000000711, -11.57481594606305997 ) ) ;
#19083=LINE ( 'NONE', #23924, #27564 ) ;
#19085=CARTESIAN_POINT ( 'NONE',  ( 204.5988444088204687, 38.12265624999999858, 9.598844408820456309 ) ) ;
#19087=FACE_OUTER_BOUND ( 'NONE', #6202, .T. ) ;
#19089=CARTESIAN_POINT ( 'NONE',  ( 59.55508561352770158, 38.02343750108394005, -13.14518615778179900 ) ) ;
#19094=DIRECTION ( 'NONE',  ( 0.000000000000000000, -1.000000000000000000, 0.000000000000000000 ) ) ;
#19095=CARTESIAN_POINT ( 'NONE',  ( 5.622872871577878406, 40.45429687500001137, 13.57481594606304576 ) ) ;
#19096=CARTESIAN_POINT ( 'NONE',  ( 51.42518405393695957, 40.65273437608393436, 0.000000000000000000 ) ) ;
#19097=EDGE_LOOP ( 'NONE', ( #12331, #1018, #16414, #23628, #8039 ) ) ;
#19098=CARTESIAN_POINT ( 'NONE',  ( 96.84719886470459471, 82.56250000136559208, -3.152801135295383084 ) ) ;
#19101=ORIENTED_EDGE ( 'NONE', *, *, #151, .F. ) ;
#19102=EDGE_CURVE ( 'NONE', #747, #4145, #3438, .T. ) ;
#19104=CARTESIAN_POINT ( 'NONE',  ( 200.6228728715777834, 37.37851562716787157, 13.57481594606313813 ) ) ;
#19105=CARTESIAN_POINT ( 'NONE',  ( 65.00000000000000000, 34.20351562608394147, -13.14518615778179544 ) ) ;
#19109=VERTEX_POINT ( 'NONE', #24682 ) ;
#19112=CARTESIAN_POINT ( 'NONE',  ( 204.5988444088204403, 36.83281250216787583, -9.598844408820458085 ) ) ;
#19113=EDGE_CURVE ( 'NONE', #26902, #17678, #11156, .T. ) ;
#19115=DIRECTION ( 'NONE',  ( 0.000000000000000000, 1.000000000000000000, 0.000000000000000000 ) ) ;
#19116=CARTESIAN_POINT ( 'NONE',  ( 201.0859442159868138, 54.65299103241510181, 14.99999999999994671 ) ) ;
#19117=CARTESIAN_POINT ( 'NONE',  ( 135.4449143864723339, 40.50390625108394005, -13.14518615778179722 ) ) ;
#19118=CARTESIAN_POINT ( 'NONE',  ( 13.14518615778179900, 39.51171875108392584, 5.444914386472293977 ) ) ;
#19121=CARTESIAN_POINT ( 'NONE',  ( 70.62287287157788285, 38.07304687499998863, 13.57481594606304576 ) ) ;
#19123=CARTESIAN_POINT ( 'NONE',  ( 198.8295627579930454, 36.00000000000000000, 12.63428651647560841 ) ) ;
#19127=( BOUNDED_CURVE ( )  B_SPLINE_CURVE ( 2, ( #10930, #2271, #15494, #4685, #10652, #19360, #9517, #27065, #7516 ),
 .UNSPECIFIED., .F., .F. ) 
 B_SPLINE_CURVE_WITH_KNOTS ( ( 3, 2, 2, 2, 3 ),
 ( 0.1041666666666664909, 0.1145833333333332732, 0.1250000000000000833, 0.1354166666666668517, 0.1458333333333336757 ),
 .UNSPECIFIED. ) 
 CURVE ( )  GEOMETRIC_REPRESENTATION_ITEM ( )  RATIONAL_B_SPLINE_CURVE ( ( 1.000000000000001332, 0.9238795325112854062, 1.000000000000000000, 0.9238795325112867385, 1.000000000000000000, 0.9238795325112867385, 1.000000000000000000, 0.9238795325112842960, 1.000000000000002442 ) ) 
 REPRESENTATION_ITEM ( '' )  );
#19128=CARTESIAN_POINT ( 'NONE',  ( 95.54126587499996504, 83.75000000136560629, 1.846868145590724986 ) ) ;
#19129=CARTESIAN_POINT ( 'NONE',  ( -9.295050272127044266, 39.26367187608393294, 9.295050272127047819 ) ) ;
#19131=CARTESIAN_POINT ( 'NONE',  ( 181.4251840539369596, 38.56914062499999574, -5.622872871577872189 ) ) ;
#19132=EDGE_LOOP ( 'NONE', ( #25800, #1601, #17443, #8447 ) ) ;
#19134=LINE ( 'NONE', #27840, #7044 ) ;
#19136=CARTESIAN_POINT ( 'NONE',  ( 94.99999999999995737, 83.06250000273119838, -2.071067811865491048 ) ) ;
#19138=AXIS2_PLACEMENT_3D ( 'NONE', #20852, #16422, #12265 ) ;
#19141=CARTESIAN_POINT ( 'NONE',  ( 65.00000000000000000, 38.56914062608393579, 13.14518615778179544 ) ) ;
#19142=CYLINDRICAL_SURFACE ( 'NONE', #23915, 13.57481594606304398 ) ;
#19146=CARTESIAN_POINT ( 'NONE',  ( -6.085944215997575846, 54.65299103241510181, -15.00000000000000000 ) ) ;
#19148=CARTESIAN_POINT ( 'NONE',  ( 143.5748159460630688, 35.14609375216787157, -1.662435489736055892E-15 ) ) ;
#19150=CARTESIAN_POINT ( 'NONE',  ( 78.14518615778179367, 39.61093750108393863, -5.444914386472297529 ) ) ;
#19152=AXIS2_PLACEMENT_3D ( 'NONE', #1491, #5485, #1630 ) ;
#19153=CARTESIAN_POINT ( 'NONE',  ( 185.7049497278729575, 36.08867187608393579, 9.295050272127047819 ) ) ;
#19158=CARTESIAN_POINT ( 'NONE',  ( -8.312177448680279460E-16, 40.00781250000000000, -13.57481594606304576 ) ) ;
#19159=CARTESIAN_POINT ( 'NONE',  ( 104.4587341249999781, 84.00000000136560629, -1.846868145590750521 ) ) ;
#19161=CARTESIAN_POINT ( 'NONE',  ( 139.5988444088204403, 40.00781250216787299, -9.598844408820458085 ) ) ;
#19162=AXIS2_PLACEMENT_3D ( 'NONE', #1367, #8037, #1229 ) ;
#19166=CARTESIAN_POINT ( 'NONE',  ( 214.9999999999999716, 50.00000000000000000, 9.999999999999946709 ) ) ;
#19167=ORIENTED_EDGE ( 'NONE', *, *, #16850, .F. ) ;
#19168=( BOUNDED_CURVE ( )  B_SPLINE_CURVE ( 2, ( #17358, #28199, #1982, #121, #14648, #15200, #1712, #26054, #6392 ),
 .UNSPECIFIED., .F., .T. ) 
 B_SPLINE_CURVE_WITH_KNOTS ( ( 3, 2, 2, 2, 3 ),
 ( 0.2291666666666665741, 0.2395833333333332316, 0.2499999999999998335, 0.2604166666666665186, 0.2708333333333330928 ),
 .UNSPECIFIED. ) 
 CURVE ( )  GEOMETRIC_REPRESENTATION_ITEM ( )  RATIONAL_B_SPLINE_CURVE ( ( 1.000000000000000666, 0.9238795325112861834, 1.000000000000000000, 0.9238795325112867385, 1.000000000000000000, 0.9238795325112867385, 1.000000000000000000, 0.9238795325112884038, 0.9999999999999983347 ) ) 
 REPRESENTATION_ITEM ( '' )  );
#19172=CARTESIAN_POINT ( 'NONE',  ( 139.2950502721270425, 37.27929687608394005, -9.295050272127046043 ) ) ;
#19173=CARTESIAN_POINT ( 'NONE',  ( 59.55508561352770158, 36.43593750108392726, -13.14518615778179900 ) ) ;
#19174=CARTESIAN_POINT ( 'NONE',  ( 195.0000000000000000, 38.96601562608393721, -13.14518615778179544 ) ) ;
#19175=CARTESIAN_POINT ( 'NONE',  ( 52.00051176980939260, 36.00000000000000000, 1.999176114741853638 ) ) ;
#19176=CARTESIAN_POINT ( 'NONE',  ( 2.414731522848535132E-15, 36.78320312608393294, 13.14518615778179544 ) ) ;
#19177=CARTESIAN_POINT ( 'NONE',  ( 128.1856446454164598, 51.46618445021834987, -14.99999999999965716 ) ) ;
#19178=CARTESIAN_POINT ( 'NONE',  ( 191.8638263786528171, 36.00000000000002842, 12.79489613812767068 ) ) ;
#19179=CARTESIAN_POINT ( 'NONE',  ( 0.000000000000000000, -7.395377635281828788, 0.000000000000000000 ) ) ;
#19180=ADVANCED_FACE ( 'NONE', ( #26973 ), #745, .F. ) ;
#19181=CARTESIAN_POINT ( 'NONE',  ( -8.049105076161786076E-16, 38.76757812608393294, -13.14518615778179544 ) ) ;
#19182=CARTESIAN_POINT ( 'NONE',  ( 8.392215291638386532, 54.99999999999999289, 14.99999999999999645 ) ) ;
#19196=CARTESIAN_POINT ( 'NONE',  ( 99.99999999999995737, 81.68750000136559208, 4.458734124999988779 ) ) ;
#19197=CARTESIAN_POINT ( 'NONE',  ( 74.29505027212704249, 38.07304687608393579, -9.295050272127046043 ) ) ;
#19199=FACE_OUTER_BOUND ( 'NONE', #17242, .T. ) ;
#19202=CARTESIAN_POINT ( 'NONE',  ( 139.1801758136479918, 55.00000000000000000, -9.999999999999998224 ) ) ;
#19204=CARTESIAN_POINT ( 'NONE',  ( 116.4251840539369596, 40.25585937499999289, 5.622872871577880183 ) ) ;
#19206=FACE_OUTER_BOUND ( 'NONE', #15667, .T. ) ;
#19209=CARTESIAN_POINT ( 'NONE',  ( 135.4449143864723055, 39.51171875108392584, -13.14518615778179900 ) ) ;
#19210=CARTESIAN_POINT ( 'NONE',  ( 55.40115559117954547, 35.64218750216787868, 9.598844408820459861 ) ) ;
#19212=CARTESIAN_POINT ( 'NONE',  ( 5.622872871577878406, 35.79101562716787299, 13.57481594606304576 ) ) ;
#19216=CARTESIAN_POINT ( 'NONE',  ( 200.4449143864723055, 38.71796875108393721, -13.14518615778179900 ) ) ;
#19217=EDGE_CURVE ( 'NONE', #1696, #18432, #24959, .T. ) ;
#19218=CARTESIAN_POINT ( 'NONE',  ( -20.00000000000000355, 55.00000000000000000, -9.999999999999998224 ) ) ;
#19220=CARTESIAN_POINT ( 'NONE',  ( 135.4449143864723339, 36.83281250108392868, 13.14518615778179189 ) ) ;
#19227=CARTESIAN_POINT ( 'NONE',  ( 200.6228728715778686, 38.37070312499999147, -13.57481594606304753 ) ) ;
#19231=CARTESIAN_POINT ( 'NONE',  ( 55.70494972787295751, 39.06523437608392868, 9.295050272127047819 ) ) ;
#19236=CARTESIAN_POINT ( 'NONE',  ( 5.622872871577871301, 40.75195312500000711, -13.57481594606304753 ) ) ;
#19237=CARTESIAN_POINT ( 'NONE',  ( 9.180175813647991845, 55.00000000000000000, -14.99999999999999822 ) ) ;
#19240=CARTESIAN_POINT ( 'NONE',  ( 95.54126587499995082, 82.75000000136560629, 1.846868145590724986 ) ) ;
#19243=VECTOR ( 'NONE', #10796, 1000.000000000000000 ) ;
#19245=CARTESIAN_POINT ( 'NONE',  ( 55.70494972787295751, 34.50117187608393721, 9.295050272127047819 ) ) ;
#19252=CARTESIAN_POINT ( 'NONE',  ( 204.5988444088204403, 39.21406250216787015, -9.598844408820458085 ) ) ;
#19255=EDGE_CURVE ( 'NONE', #1369, #2793, #2072, .T. ) ;
#19256=CARTESIAN_POINT ( 'NONE',  ( 3.100818213308542287E-15, 52.00000000000000711, 12.99999999999999645 ) ) ;
#19257=CARTESIAN_POINT ( 'NONE',  ( 201.8735082435670449, 51.14166184781640112, 15.00000000000191669 ) ) ;
#19258=CARTESIAN_POINT ( 'NONE',  ( 120.7049497278729575, 39.26367187608393294, 9.295050272127047819 ) ) ;
#19259=CARTESIAN_POINT ( 'NONE',  ( -8.049105076161786076E-16, 37.37851562608393863, -13.14518615778179544 ) ) ;
#19261=CARTESIAN_POINT ( 'NONE',  ( 143.1451861577818079, 33.80664062608393294, -1.609821015232357215E-15 ) ) ;
#19262=CARTESIAN_POINT ( 'NONE',  ( 51.42518405393695957, 38.61874999999999147, 0.000000000000000000 ) ) ;
#19263=CARTESIAN_POINT ( 'NONE',  ( 51.42518405393695957, 39.46210937716787726, -5.622872871577872189 ) ) ;
#19273=CARTESIAN_POINT ( 'NONE',  ( 9.295050272127046043, 39.66054687608393436, -9.295050272127046043 ) ) ;
#19276=ORIENTED_EDGE ( 'NONE', *, *, #6013, .T. ) ;
#19279=CYLINDRICAL_SURFACE ( 'NONE', #11173, 13.57481594606304398 ) ;
#19282=CARTESIAN_POINT ( 'NONE',  ( 208.1451861577817795, 39.31328125108392868, 5.444914386472293977 ) ) ;
#19286=CARTESIAN_POINT ( 'NONE',  ( 130.0000000000000000, 40.00781250000000000, -13.57481594606304576 ) ) ;
#19288=ORIENTED_EDGE ( 'NONE', *, *, #8641, .T. ) ;
#19291=CARTESIAN_POINT ( 'NONE',  ( 120.4011555911795455, 34.05468750216788010, 9.598844408820459861 ) ) ;
#19292=( BOUNDED_CURVE ( )  B_SPLINE_CURVE ( 2, ( #1206, #1480, #1758, #27283, #16571, #19131, #16715, #12135, #6029 ),
 .UNSPECIFIED., .F., .F. ) 
 B_SPLINE_CURVE_WITH_KNOTS ( ( 3, 2, 2, 2, 3 ),
 ( 0.2291666666666665741, 0.2395833333333332316, 0.2499999999999998335, 0.2604166666666665186, 0.2708333333333330928 ),
 .UNSPECIFIED. ) 
 CURVE ( )  GEOMETRIC_REPRESENTATION_ITEM ( )  RATIONAL_B_SPLINE_CURVE ( ( 1.000000000000000666, 0.9238795325112861834, 1.000000000000000000, 0.9238795325112867385, 1.000000000000000000, 0.9238795325112867385, 1.000000000000000000, 0.9238795325112884038, 0.9999999999999983347 ) ) 
 REPRESENTATION_ITEM ( '' )  );
#19293=CARTESIAN_POINT ( 'NONE',  ( 65.00000000000000000, 40.55351562608393579, -13.14518615778179544 ) ) ;
#19294=ADVANCED_FACE ( 'NONE', ( #10529, #10245 ), #14393, .F. ) ;
#19295=CARTESIAN_POINT ( 'NONE',  ( 204.2950502721270425, 33.31054687608394005, -9.295050272127046043 ) ) ;
#19297=EDGE_LOOP ( 'NONE', ( #3978, #7116, #7578, #1828 ) ) ;
#19300=CARTESIAN_POINT ( 'NONE',  ( 96.46446609406721961, 84.12500000000000000, 3.535533905932727539 ) ) ;
#19302=CARTESIAN_POINT ( 'NONE',  ( 104.4587341249999781, 80.87500000136560629, 1.846868145590721655 ) ) ;
#19303=DIRECTION ( 'NONE',  ( -0.000000000000000000, 1.000000000000000000, -0.000000000000000000 ) ) ;
#19307=CARTESIAN_POINT ( 'NONE',  ( 195.0000000000000000, 39.75976562608394005, -13.14518615778179544 ) ) ;
#19308=CARTESIAN_POINT ( 'NONE',  ( 130.0000000000000000, 32.07031249999999289, -13.57481594606304576 ) ) ;
#19313=CARTESIAN_POINT ( 'NONE',  ( 130.0000000000000000, 37.37851562608393863, -13.14518615778179544 ) ) ;
#19314=CARTESIAN_POINT ( 'NONE',  ( 78.14518615778179367, 36.18789062608393436, -1.609821015232357215E-15 ) ) ;
#19315=CARTESIAN_POINT ( 'NONE',  ( 204.2950502721270425, 32.11992187608393579, 9.295050272127046043 ) ) ;
#19317=CARTESIAN_POINT ( 'NONE',  ( 13.14518615778179900, 35.44375000108393436, -5.444914386472297529 ) ) ;
#19318=CARTESIAN_POINT ( 'NONE',  ( 123.1264917564389236, 51.14166184780616931, -15.00000000000458300 ) ) ;
#19319=CARTESIAN_POINT ( 'NONE',  ( 187.9316343120018189, 35.99999999999998579, 11.09140360074139586 ) ) ;
#19321=CARTESIAN_POINT ( 'NONE',  ( 9.295050272127046043, 39.46210937608393010, -9.295050272127046043 ) ) ;
#19324=CARTESIAN_POINT ( 'NONE',  ( 62.83004341689117922, 49.99999999883938528, 13.43548448457802991 ) ) ;
#19326=CARTESIAN_POINT ( 'NONE',  ( 78.40642364673431075, 35.99999999999999289, 1.227293221036817483 ) ) ;
#19327=VERTEX_POINT ( 'NONE', #8540 ) ;
#19333=CARTESIAN_POINT ( 'NONE',  ( 96.84719886470459471, 82.56250000136559208, -3.152801135295383084 ) ) ;
#19334=CARTESIAN_POINT ( 'NONE',  ( 55.70494972787295751, 37.67617187608393436, 9.295050272127047819 ) ) ;
#19335=( BOUNDED_CURVE ( )  B_SPLINE_CURVE ( 2, ( #24769, #18356, #11920, #16632, #27063, #27208, #20641, #22923, #7513 ),
 .UNSPECIFIED., .F., .F. ) 
 B_SPLINE_CURVE_WITH_KNOTS ( ( 3, 2, 2, 2, 3 ),
 ( 0.1458333333333336757, 0.1562500000000002776, 0.1666666666666669072, 0.1770833333333335369, 0.1875000000000001388 ),
 .UNSPECIFIED. ) 
 CURVE ( )  GEOMETRIC_REPRESENTATION_ITEM ( )  RATIONAL_B_SPLINE_CURVE ( ( 0.9999999999999975575, 0.9238795325112891810, 1.000000000000000000, 0.9238795325112867385, 1.000000000000000000, 0.9238795325112867385, 1.000000000000000000, 0.9238795325112857393, 1.000000000000001110 ) ) 
 REPRESENTATION_ITEM ( '' )  );
#19341=CARTESIAN_POINT ( 'NONE',  ( 135.4449143864723055, 32.56640625108394005, -13.14518615778179900 ) ) ;
#19342=ORIENTED_EDGE ( 'NONE', *, *, #23880, .F. ) ;
#19346=CARTESIAN_POINT ( 'NONE',  ( 95.54126587499995082, 80.37500000136562051, -1.846868145590750077 ) ) ;
#19347=CARTESIAN_POINT ( 'NONE',  ( 135.4449143864723055, 37.92421875108392726, -13.14518615778179900 ) ) ;
#19348=CARTESIAN_POINT ( 'NONE',  ( 65.00000000000000000, 37.72578125216787726, -13.57481594606304576 ) ) ;
#19351=CARTESIAN_POINT ( 'NONE',  ( 13.57481594606304576, 36.73359375216787015, -1.662435489736055892E-15 ) ) ;
#19354=CARTESIAN_POINT ( 'NONE',  ( 189.5550856135277229, 38.81718750108393579, -13.14518615778179900 ) ) ;
#19355=VECTOR ( 'NONE', #12105, 1000.000000000000000 ) ;
#19358=DIRECTION ( 'NONE',  ( -0.000000000000000000, 1.000000000000000000, -0.000000000000000000 ) ) ;
#19360=CARTESIAN_POINT ( 'NONE',  ( 208.5748159460630688, 39.06523437716786873, 5.622872871577868636 ) ) ;
#19364=CARTESIAN_POINT ( 'NONE',  ( 189.3771271284221314, 39.26367187499999289, -13.57481594606304753 ) ) ;
#19367=CARTESIAN_POINT ( 'NONE',  ( 74.29505027212704249, 39.46210937608393010, -9.295050272127046043 ) ) ;
#19373=CARTESIAN_POINT ( 'NONE',  ( 13.57481594606304753, 38.27148437500000711, -5.622872871577873077 ) ) ;
#19374=CARTESIAN_POINT ( 'NONE',  ( 135.4449143864723055, 39.71015625108393010, -13.14518615778179900 ) ) ;
#19376=CARTESIAN_POINT ( 'NONE',  ( 99.99999999999995737, 83.75000000000000000, -5.000000000000018652 ) ) ;
#19380=FACE_OUTER_BOUND ( 'NONE', #16956, .T. ) ;
#19381=CARTESIAN_POINT ( 'NONE',  ( 51.85481384221820633, 33.60820312608393579, 0.000000000000000000 ) ) ;
#19385=ORIENTED_EDGE ( 'NONE', *, *, #8274, .F. ) ;
#19386=CARTESIAN_POINT ( 'NONE',  ( 94.99999999999995737, 82.12500000273119838, -1.387778780781445676E-14 ) ) ;
#19388=CARTESIAN_POINT ( 'NONE',  ( 185.4011555911795313, 37.82500000216787583, -9.598844408820458085 ) ) ;
#19390=CARTESIAN_POINT ( 'NONE',  ( 74.59884440882045453, 36.03906250216787299, -9.598844408820458085 ) ) ;
#19392=CARTESIAN_POINT ( 'NONE',  ( 130.0000000000000000, 40.55351562608393579, -13.14518615778179544 ) ) ;
#19393=VERTEX_POINT ( 'NONE', #7984 ) ;
#19394=CARTESIAN_POINT ( 'NONE',  ( -9.295050272127044266, 38.46992187608393721, 9.295050272127047819 ) ) ;
#19395=CARTESIAN_POINT ( 'NONE',  ( 116.8548138422182063, 34.15390625108393863, -5.444914386472297529 ) ) ;
#19396=CARTESIAN_POINT ( 'NONE',  ( 70.62287287157788285, 38.86679687499999858, 13.57481594606304576 ) ) ;
#19399=DIRECTION ( 'NONE',  ( 0.000000000000000000, 0.000000000000000000, 1.000000000000000000 ) ) ;
#19403=DIRECTION ( 'NONE',  ( -0.000000000000000000, -1.000000000000000000, -0.000000000000000000 ) ) ;
#19406=CARTESIAN_POINT ( 'NONE',  ( 5.444914386472297529, 39.71015625108393010, -13.14518615778179900 ) ) ;
#19411=EDGE_CURVE ( 'NONE', #19690, #20676, #15448, .T. ) ;
#19415=CARTESIAN_POINT ( 'NONE',  ( 204.2950502721270425, 37.87460937608393152, -9.295050272127046043 ) ) ;
#19416=ORIENTED_EDGE ( 'NONE', *, *, #12410, .T. ) ;
#19417=FACE_OUTER_BOUND ( 'NONE', #23436, .T. ) ;
#19419=CARTESIAN_POINT ( 'NONE',  ( -15.00000000000000355, 80.00000000000000000, -10.00000000000000000 ) ) ;
#19427=CARTESIAN_POINT ( 'NONE',  ( 139.5988444088204687, 33.45937500216787441, 9.598844408820456309 ) ) ;
#19429=VECTOR ( 'NONE', #10142, 1000.000000000000000 ) ;
#19430=CARTESIAN_POINT ( 'NONE',  ( 74.29505027212704249, 39.66054687608393436, -9.295050272127046043 ) ) ;
#19432=CARTESIAN_POINT ( 'NONE',  ( 181.8548138422181921, 34.45156250108394147, 5.444914386472304635 ) ) ;
#19433=ORIENTED_EDGE ( 'NONE', *, *, #27563, .F. ) ;
#19438=CARTESIAN_POINT ( 'NONE',  ( 70.44491438647229131, 39.51171875108393294, -13.14518615778179722 ) ) ;
#19440=CARTESIAN_POINT ( 'NONE',  ( 98.15313185440923860, 79.62500000136560629, 4.458734124999987891 ) ) ;
#19441=CARTESIAN_POINT ( 'NONE',  ( 208.1451861577818079, 39.31328125108392868, 5.444914386472293977 ) ) ;
#19444=CARTESIAN_POINT ( 'NONE',  ( 65.00000000000000000, -7.395377635281828788, -7.517135062566165128E-15 ) ) ;
#19445=CARTESIAN_POINT ( 'NONE',  ( 204.2950502721270425, 40.45429687608393721, -9.295050272127046043 ) ) ;
#19452=CARTESIAN_POINT ( 'NONE',  ( 139.2950502721270425, 36.28710937608393294, 9.295050272127046043 ) ) ;
#19454=CARTESIAN_POINT ( 'NONE',  ( 51.85481384221820633, 32.61601562608393579, 0.000000000000000000 ) ) ;
#19455=EDGE_CURVE ( 'NONE', #26410, #11953, #17511, .T. ) ;
#19456=CARTESIAN_POINT ( 'NONE',  ( 200.4449143864723055, 37.82500000108392868, 13.14518615778179189 ) ) ;
#19458=CARTESIAN_POINT ( 'NONE',  ( 2.414731522848535132E-15, 33.60820312608392868, 13.14518615778179544 ) ) ;
#19459=CARTESIAN_POINT ( 'NONE',  ( 136.1610621748488938, 51.27996893916987631, -15.00000000000069278 ) ) ;
#19464=CARTESIAN_POINT ( 'NONE',  ( 13.14518615778179544, 37.77539062608393294, -1.609821015232357215E-15 ) ) ;
#19472=CARTESIAN_POINT ( 'NONE',  ( 59.37712712842216689, 38.07304687716787583, 13.57481594606308128 ) ) ;
#19474=CARTESIAN_POINT ( 'NONE',  ( 124.3771271284219893, 38.86679687716787868, 13.57481594606290720 ) ) ;
#19475=CARTESIAN_POINT ( 'NONE',  ( 99.99999999999995737, 80.43750000136559208, -4.458734125000016313 ) ) ;
#19476=CARTESIAN_POINT ( 'NONE',  ( 70.44491438647230552, 35.44375000108393436, 13.14518615778179189 ) ) ;
#19478=CARTESIAN_POINT ( 'NONE',  ( 13.14518615778179722, 39.41250000108393436, -5.444914386472297529 ) ) ;
#19482=CARTESIAN_POINT ( 'NONE',  ( 102.0710678118654045, 82.31250000000002842, 5.000000000000019540 ) ) ;
#19483=CARTESIAN_POINT ( 'NONE',  ( 130.0000000000000000, 39.21406249999999716, -13.57481594606304576 ) ) ;
#19484=ORIENTED_EDGE ( 'NONE', *, *, #6021, .F. ) ;
#19485=EDGE_CURVE ( 'NONE', #11153, #2183, #8450, .T. ) ;
#19489=CARTESIAN_POINT ( 'NONE',  ( 124.5550856135277087, 35.93984375108392726, 13.14518615778179722 ) ) ;
#19490=CARTESIAN_POINT ( 'NONE',  ( 59.37712712842213136, 32.51679687716787726, 13.57481594606304753 ) ) ;
#19491=CARTESIAN_POINT ( 'NONE',  ( 104.9999999999999716, 83.43750000000001421, 2.071067811865462627 ) ) ;
#19492=CARTESIAN_POINT ( 'NONE',  ( -9.598844408820454532, 35.64218750216787868, 9.598844408820459861 ) ) ;
#19495=ORIENTED_EDGE ( 'NONE', *, *, #18902, .F. ) ;
#19497=CARTESIAN_POINT ( 'NONE',  ( 181.8548138422182205, 38.96601562608393721, 0.000000000000000000 ) ) ;
#19499=CARTESIAN_POINT ( 'NONE',  ( 135.9085077471930276, 36.04503594658366694, 12.68159279706107334 ) ) ;
#19501=( BOUNDED_CURVE ( )  B_SPLINE_CURVE ( 2, ( #5787, #5368, #18614, #18333, #27040, #24746, #20616, #25158, #27320 ),
 .UNSPECIFIED., .F., .F. ) 
 B_SPLINE_CURVE_WITH_KNOTS ( ( 3, 2, 2, 2, 3 ),
 ( 0.2291666666666665741, 0.2395833333333332316, 0.2499999999999998335, 0.2604166666666665186, 0.2708333333333330928 ),
 .UNSPECIFIED. ) 
 CURVE ( )  GEOMETRIC_REPRESENTATION_ITEM ( )  RATIONAL_B_SPLINE_CURVE ( ( 1.000000000000000666, 0.9238795325112861834, 1.000000000000000000, 0.9238795325112867385, 1.000000000000000000, 0.9238795325112867385, 1.000000000000000000, 0.9238795325112884038, 0.9999999999999983347 ) ) 
 REPRESENTATION_ITEM ( '' )  );
#19502=CARTESIAN_POINT ( 'NONE',  ( 55.81982418635200105, 55.00000000000014211, -9.999999999999998224 ) ) ;
#19505=CARTESIAN_POINT ( 'NONE',  ( 195.0000000000000000, 38.42031249999999432, -13.57481594606304576 ) ) ;
#19508=CARTESIAN_POINT ( 'NONE',  ( 189.3771271284221314, 36.08867187500000284, -13.57481594606304753 ) ) ;
#19509=CARTESIAN_POINT ( 'NONE',  ( 55.40115559117954547, 40.10703124999999147, -9.598844408820458085 ) ) ;
#19511=CARTESIAN_POINT ( 'NONE',  ( 55.70494972787295751, 39.66054687608393436, -9.295050272127046043 ) ) ;
#19513=DIRECTION ( 'NONE',  ( 0.000000000000000000, 0.000000000000000000, 1.000000000000000000 ) ) ;
#19516=CARTESIAN_POINT ( 'NONE',  ( -13.57481594606304576, 37.08085937499999574, 5.622872871577880183 ) ) ;
#19517=CARTESIAN_POINT ( 'NONE',  ( 116.8548138422182063, 40.70234375108393721, -5.444914386472297529 ) ) ;
#19518=CIRCLE ( 'NONE', #23166, 5.000000000000000888 ) ;
#19520=CARTESIAN_POINT ( 'NONE',  ( 94.99999999999995737, 84.93750000000001421, -2.071067811865491048 ) ) ;
#19525=CARTESIAN_POINT ( 'NONE',  ( 70.44491438647230552, 35.74140625108393721, -13.14518615778179900 ) ) ;
#19529=ORIENTED_EDGE ( 'NONE', *, *, #13642, .T. ) ;
#19532=CARTESIAN_POINT ( 'NONE',  ( 189.3771271284221314, 38.86679687716788578, 13.57481594606304753 ) ) ;
#19534=CARTESIAN_POINT ( 'NONE',  ( -9.180175813647991845, 55.00000000000000000, -14.99999999999999822 ) ) ;
#19535=CARTESIAN_POINT ( 'NONE',  ( 193.0526740779191357, 51.47162402671692405, 15.00000000000193090 ) ) ;
#19536=CARTESIAN_POINT ( 'NONE',  ( 120.7049497278729575, 36.68398437608393436, -9.295050272127046043 ) ) ;
#19538=CARTESIAN_POINT ( 'NONE',  ( 13.14518615778179900, 38.71796875108393721, 5.444914386472293977 ) ) ;
#19540=CARTESIAN_POINT ( 'NONE',  ( 120.7049497278729575, 33.31054687608393294, -9.295050272127046043 ) ) ;
#19541=CARTESIAN_POINT ( 'NONE',  ( 65.00000000000000000, 34.05468749999999289, 13.57481594606304576 ) ) ;
#19542=CARTESIAN_POINT ( 'NONE',  ( 5.622872871577912157, 38.17226562716787441, 13.57481594606301023 ) ) ;
#19543=AXIS2_PLACEMENT_3D ( 'NONE', #4730, #10833, #17543 ) ;
#19545=CARTESIAN_POINT ( 'NONE',  ( 99.99999999999995737, 83.87500000273119838, -5.000000000000018652 ) ) ;
#19548=CARTESIAN_POINT ( 'NONE',  ( 99.99999999999995737, 85.00000000000000000, -1.387778780781445676E-14 ) ) ;
#19551=CARTESIAN_POINT ( 'NONE',  ( 13.14518615778179900, 38.02343750108395426, -5.444914386472297529 ) ) ;
#19555=CARTESIAN_POINT ( 'NONE',  ( 116.4251840539369596, 37.08085937716787583, -5.622872871577872189 ) ) ;
#19557=CARTESIAN_POINT ( 'NONE',  ( 185.7049497278729575, 40.45429687608393721, -9.295050272127046043 ) ) ;
#19562=ORIENTED_EDGE ( 'NONE', *, *, #12437, .F. ) ;
#19566=CARTESIAN_POINT ( 'NONE',  ( 143.1451861577818079, 39.36289062608393152, -1.609821015232357215E-15 ) ) ;
#19567=CARTESIAN_POINT ( 'NONE',  ( -13.14518615778179544, 40.75195312608393294, 0.000000000000000000 ) ) ;
#19569=CARTESIAN_POINT ( 'NONE',  ( 99.99999999999995737, 81.87500000273119838, -5.000000000000018652 ) ) ;
#19570=EDGE_CURVE ( 'NONE', #26178, #6416, #8682, .T. ) ;
#19571=SPHERICAL_SURFACE ( 'NONE', #10441, 5.000000000000000000 ) ;
#19572=CARTESIAN_POINT ( 'NONE',  ( 200.4449143864723055, 34.15390625108393863, -13.14518615778179900 ) ) ;
#19573=ORIENTED_EDGE ( 'NONE', *, *, #20104, .T. ) ;
#19575=ORIENTED_EDGE ( 'NONE', *, *, #618, .F. ) ;
#19578=CARTESIAN_POINT ( 'NONE',  ( 51.85481384221821344, 39.01562500108393294, 5.444914386472304635 ) ) ;
#19579=CARTESIAN_POINT ( 'NONE',  ( 95.54126587499996504, 80.37500000136563472, -1.846868145590750077 ) ) ;
#19580=CARTESIAN_POINT ( 'NONE',  ( 204.2950502721270425, 40.05742187608392868, 9.295050272127046043 ) ) ;
#19584=DIRECTION ( 'NONE',  ( -0.000000000000000000, -1.000000000000000000, -0.000000000000000000 ) ) ;
#19587=EDGE_CURVE ( 'NONE', #5192, #12549, #7989, .T. ) ;
#19592=CARTESIAN_POINT ( 'NONE',  ( 130.0000000000000000, 34.99726562608393721, -13.14518615778179544 ) ) ;
#19593=CARTESIAN_POINT ( 'NONE',  ( 65.00000000000000000, 32.81445312608393294, 13.14518615778179544 ) ) ;
#19594=CARTESIAN_POINT ( 'NONE',  ( 208.1451861577817795, 37.13046875108393863, 5.444914386472293977 ) ) ;
#19596=CARTESIAN_POINT ( 'NONE',  ( 126.9553905430760636, 53.89089363584123049, -14.99999999999999822 ) ) ;
#19597=CARTESIAN_POINT ( 'NONE',  ( 195.0000000000000000, 39.71015625216787015, 13.57481594606304576 ) ) ;
#19599=DIRECTION ( 'NONE',  ( 0.000000000000000000, -1.000000000000000000, 0.000000000000000000 ) ) ;
#19601=CARTESIAN_POINT ( 'NONE',  ( 13.14518615778179900, 33.85625000108393579, -5.444914386472297529 ) ) ;
#19602=CARTESIAN_POINT ( 'NONE',  ( 99.99999999999995737, 82.75000000000000000, -5.000000000000018652 ) ) ;
#19603=CARTESIAN_POINT ( 'NONE',  ( 99.99999999999995737, 79.87500000273119838, -5.000000000000018652 ) ) ;
#19605=EDGE_LOOP ( 'NONE', ( #4792, #9773, #5342, #1844 ) ) ;
#19610=CARTESIAN_POINT ( 'NONE',  ( 51.42518405393695957, 37.92421875216787441, 0.000000000000000000 ) ) ;
#19611=EDGE_CURVE ( 'NONE', #9045, #3560, #23462, .T. ) ;
#19614=CARTESIAN_POINT ( 'NONE',  ( 104.4587341249999781, 80.25000000136559208, -1.846868145590750299 ) ) ;
#19615=CARTESIAN_POINT ( 'NONE',  ( 70.44491438647230552, 34.15390625108393863, -13.14518615778179900 ) ) ;
#19617=DIRECTION ( 'NONE',  ( -0.000000000000000000, 1.000000000000000000, -0.000000000000000000 ) ) ;
#19618=VERTEX_POINT ( 'NONE', #708 ) ;
#19619=DIRECTION ( 'NONE',  ( -1.000000000000000000, 0.000000000000000000, 0.000000000000000000 ) ) ;
#19622=CARTESIAN_POINT ( 'NONE',  ( 116.4251840539369596, 37.03124999999999289, 0.000000000000000000 ) ) ;
#19624=VERTEX_POINT ( 'NONE', #11794 ) ;
#19629=CARTESIAN_POINT ( 'NONE',  ( 124.5550856135277087, 35.64218750108392442, -13.14518615778179900 ) ) ;
#19630=CARTESIAN_POINT ( 'NONE',  ( 59.37712712842213136, 33.31054687716787299, 13.57481594606304753 ) ) ;
#19632=CARTESIAN_POINT ( 'NONE',  ( -9.598844408820454532, 32.46718750216787441, 9.598844408820459861 ) ) ;
#19634=DIRECTION ( 'NONE',  ( -1.000000000000000000, 0.000000000000000000, 0.000000000000000000 ) ) ;
#19635=CARTESIAN_POINT ( 'NONE',  ( 208.1451861577817795, 35.34453125108392868, 5.444914386472293977 ) ) ;
#19640=CARTESIAN_POINT ( 'NONE',  ( 137.6165253254808363, 54.91574374957785665, 14.99999999999996447 ) ) ;
#19642=CARTESIAN_POINT ( 'NONE',  ( 143.5748159460630688, 38.17226562499999432, 5.622872871577868636 ) ) ;
#19645=CARTESIAN_POINT ( 'NONE',  ( 181.4251840539369596, 35.39414062499999147, -5.622872871577873077 ) ) ;
#19646=EDGE_CURVE ( 'NONE', #21223, #11873, #16718, .T. ) ;
#19649=CARTESIAN_POINT ( 'NONE',  ( 51.85481384221819923, 35.74140625108393721, -5.444914386472297529 ) ) ;
#19654=CARTESIAN_POINT ( 'NONE',  ( 13.57481594606304753, 35.09648437499998863, -5.622872871577873077 ) ) ;
#19655=CARTESIAN_POINT ( 'NONE',  ( 130.0000000000000000, 37.37851562608393863, -13.14518615778179544 ) ) ;
#19658=CARTESIAN_POINT ( 'NONE',  ( 98.15313185440925281, 79.87500000136559208, 4.458734124999987891 ) ) ;
#19659=CARTESIAN_POINT ( 'NONE',  ( 94.99999999999995737, 84.12500000273119838, -1.387778780781445676E-14 ) ) ;
#19661=CARTESIAN_POINT ( 'NONE',  ( 63.72886122875935655, 36.00000000000000000, -13.43002483374384504 ) ) ;
#19664=CARTESIAN_POINT ( 'NONE',  ( 51.85481384221820633, 35.98945312608393721, 0.000000000000000000 ) ) ;
#19665=VERTEX_POINT ( 'NONE', #16224 ) ;
#19668=ORIENTED_EDGE ( 'NONE', *, *, #27980, .F. ) ;
#19670=( BOUNDED_SURFACE ( )  B_SPLINE_SURFACE ( 3, 2, ( 
 ( #13280, #19863, #15288 ),
 ( #26138, #19720, #206 ),
 ( #8890, #350, #12995 ),
 ( #66, #21735, #8748 ),
 ( #6604, #24006, #4483 ),
 ( #13139, #3872, #2159 ),
 ( #10548, #4291, #12950 ),
 ( #6149, #19535, #24340 ),
 ( #15094, #23399, #16838 ),
 ( #8144, #21684, #25535 ),
 ( #26091, #10820, #8559 ),
 ( #6015, #8701, #12534 ),
 ( #28096, #14678, #17250 ),
 ( #27823, #21262, #17 ),
 ( #27957, #8413, #25667 ),
 ( #1744, #10409, #12681 ),
 ( #6943, #19257, #19116 ),
 ( #17392, #15639, #14814 ),
 ( #13486, #17103, #8277 ),
 ( #16968, #23539, #4015 ) ),
 .UNSPECIFIED., .F., .F., .F. ) 
 B_SPLINE_SURFACE_WITH_KNOTS ( ( 4, 2, 2, 2, 2, 2, 2, 2, 2, 4 ),
 ( 3, 3 ),
 ( 0.009073803551359451228, 0.01139250602759180747, 0.01371120850382416198, 0.01602991098005651649, 0.01834861345628887100, 0.01950796469440504999, 0.02066731593252122551, 0.02298601840875358349, 0.02530472088498593800, 0.02762342336121829250 ),
 ( 0.000000000000000000, 1.000000000000000000 ),
 .UNSPECIFIED. ) 
 GEOMETRIC_REPRESENTATION_ITEM ( )  RATIONAL_B_SPLINE_SURFACE ( (
 ( 1.000000000000000000, 0.7071067811865473507, 1.000000000000000000),
 ( 1.000000000000000000, 0.7344871497831124696, 1.000000000000000000),
 ( 1.000000000000000000, 0.7612510203315875357, 1.000000000000000000),
 ( 1.000000000000000000, 0.8116663633846998849, 1.000000000000000000),
 ( 1.000000000000000000, 0.8353358059748190456, 1.000000000000000000),
 ( 1.000000000000000000, 0.8764699612589672562, 1.000000000000000000),
 ( 1.000000000000000000, 0.8939017358720030559, 1.000000000000000000),
 ( 1.000000000000000000, 0.9185314935646274881, 1.000000000000000000),
 ( 1.000000000000000000, 0.9256439951239916475, 1.000000000000000000),
 ( 1.000000000000000000, 0.9261623622476302664, 1.000000000000000000),
 ( 1.000000000000000000, 0.9246301385979290854, 1.000000000000000000),
 ( 1.000000000000000000, 0.9183304321347592891, 1.000000000000000000),
 ( 1.000000000000000000, 0.9135987334167980922, 1.000000000000000000),
 ( 1.000000000000000000, 0.8954110486040549599, 1.000000000000000000),
 ( 1.000000000000000000, 0.8779877431160497681, 1.000000000000000000),
 ( 1.000000000000000000, 0.8366182664713029959, 1.000000000000000000),
 ( 1.000000000000000000, 0.8126941604021775678, 1.000000000000000000),
 ( 1.000000000000000000, 0.7617527316299470552, 1.000000000000000000),
 ( 1.000000000000000000, 0.7347103785796862407, 1.000000000000000000),
 ( 1.000000000000000000, 0.7071067811865470176, 1.000000000000000000) ) ) 
 REPRESENTATION_ITEM ( '' )  SURFACE ( )  );
#19672=CARTESIAN_POINT ( 'NONE',  ( 208.5748159460630120, 35.98945312716787015, -5.622872871577873077 ) ) ;
#19674=CARTESIAN_POINT ( 'NONE',  ( 51.63999894807758295, 40.87597656304196647, 0.000000000000000000 ) ) ;
#19675=CARTESIAN_POINT ( 'NONE',  ( 143.1451861577818363, 37.22968750108394431, -5.444914386472297529 ) ) ;
#19677=CARTESIAN_POINT ( 'NONE',  ( -8.049105076161786076E-16, 38.96601562608393721, -13.14518615778179544 ) ) ;
#19678=CARTESIAN_POINT ( 'NONE',  ( 139.2950502721270425, 35.49335937608393010, -9.295050272127046043 ) ) ;
#19679=CARTESIAN_POINT ( 'NONE',  ( 65.00000000000000000, 33.65781249999999147, -13.57481594606304576 ) ) ;
#19680=CARTESIAN_POINT ( 'NONE',  ( 13.57481594606304753, 38.37070312716787157, -5.622872871577873966 ) ) ;
#19686=CARTESIAN_POINT ( 'NONE',  ( 99.99999999999995737, 79.93750000136559208, 4.458734124999988779 ) ) ;
#19688=CARTESIAN_POINT ( 'NONE',  ( -9.295050272127046043, 37.47773437608393010, -9.295050272127046043 ) ) ;
#19690=VERTEX_POINT ( 'NONE', #22937 ) ;
#19695=CARTESIAN_POINT ( 'NONE',  ( 195.0000000000000000, 38.76757812608393294, -13.14518615778179544 ) ) ;
#19697=CARTESIAN_POINT ( 'NONE',  ( 139.1801758136479918, 55.00000000000000000, 14.99999999999996270 ) ) ;
#19705=CARTESIAN_POINT ( 'NONE',  ( 116.4251840539369596, 31.62382812716787228, 5.622872871577880183 ) ) ;
#19706=CARTESIAN_POINT ( 'NONE',  ( 5.444914386472297529, 39.71015625108393010, -13.14518615778179722 ) ) ;
#19709=CARTESIAN_POINT ( 'NONE',  ( 78.14518615778179367, 37.92421875108392726, 5.444914386472293977 ) ) ;
#19711=CARTESIAN_POINT ( 'NONE',  ( 189.5550856135277229, 35.34453125108393579, 13.14518615778179722 ) ) ;
#19712=ORIENTED_EDGE ( 'NONE', *, *, #1669, .T. ) ;
#19716=CARTESIAN_POINT ( 'NONE',  ( 78.14518615778180788, 40.20625000108393010, -5.444914386472297529 ) ) ;
#19717=CARTESIAN_POINT ( 'NONE',  ( 103.1528011352953342, 80.06250000136559208, -3.152801135295383084 ) ) ;
#19718=CARTESIAN_POINT ( 'NONE',  ( 195.0000000000000000, 38.76757812608393294, -13.14518615778179544 ) ) ;
#19720=CARTESIAN_POINT ( 'NONE',  ( 186.2273907538555591, 50.37415326815735028, 15.00000000000776978 ) ) ;
#19722=CARTESIAN_POINT ( 'NONE',  ( 204.2950502721270425, 40.25585937608393294, 9.295050272127046043 ) ) ;
#19725=AXIS2_PLACEMENT_3D ( 'NONE', #9366, #18060, #26775 ) ;
#19729=CARTESIAN_POINT ( 'NONE',  ( 116.8548138422182063, 36.83281250108393579, 5.444914386472304635 ) ) ;
#19730=CARTESIAN_POINT ( 'NONE',  ( 65.00000000000000000, 34.40195312608393152, 13.14518615778179544 ) ) ;
#19731=CARTESIAN_POINT ( 'NONE',  ( 208.1451861577818079, 37.97382812608393721, -1.609821015232357215E-15 ) ) ;
#19733=EDGE_LOOP ( 'NONE', ( #2776, #27996, #13943, #25706 ) ) ;
#19734=CARTESIAN_POINT ( 'NONE',  ( 64.40674429744949236, 36.00000000000001421, 13.13889047851772851 ) ) ;
#19735=CARTESIAN_POINT ( 'NONE',  ( -5.444914386472299306, 32.76484375108393010, 13.14518615778179722 ) ) ;
#19736=CARTESIAN_POINT ( 'NONE',  ( 129.2761280619777153, 53.51529642094997286, -15.00000000000000000 ) ) ;
#19737=CARTESIAN_POINT ( 'NONE',  ( -20.00000000000000000, 55.00000000000000000, 10.00000000000000178 ) ) ;
#19738=CARTESIAN_POINT ( 'NONE',  ( 120.4011555911795455, 39.61093750216787868, 9.598844408820459861 ) ) ;
#19740=CARTESIAN_POINT ( 'NONE',  ( 197.1298106584279992, 36.02027164734404607, -13.57481594606306174 ) ) ;
#19742=CARTESIAN_POINT ( 'NONE',  ( 61.13607473487752486, 54.10645156200381223, 14.99999999999998401 ) ) ;
#19743=( NAMED_UNIT ( * ) PLANE_ANGLE_UNIT ( ) SI_UNIT ( $, .RADIAN. ) );
#19749=CARTESIAN_POINT ( 'NONE',  ( 132.0246277255328664, 50.00000000050972915, 13.43320860980955089 ) ) ;
#19751=DIRECTION ( 'NONE',  ( 1.000000000000000000, 0.000000000000000000, -2.385244779468110248E-16 ) ) ;
#19752=CARTESIAN_POINT ( 'NONE',  ( 95.54126587499996504, 81.68750000136559208, -1.387778780781445676E-14 ) ) ;
#19753=CARTESIAN_POINT ( 'NONE',  ( 59.55508561352770158, 36.63437500108393152, -13.14518615778179900 ) ) ;
#19754=EDGE_CURVE ( 'NONE', #2330, #16552, #2990, .T. ) ;
#19756=CARTESIAN_POINT ( 'NONE',  ( -13.14518615778179189, 37.42812500108393436, 5.444914386472304635 ) ) ;
#19758=CARTESIAN_POINT ( 'NONE',  ( 116.4251840539369596, 36.23749999999999005, 0.000000000000000000 ) ) ;
#19759=CARTESIAN_POINT ( 'NONE',  ( 103.5355339059327093, 82.62500000000000000, -3.535533905932755072 ) ) ;
#19760=CARTESIAN_POINT ( 'NONE',  ( 135.6228728715778971, 36.48554687499999716, 13.57481594606304576 ) ) ;
#19761=ORIENTED_EDGE ( 'NONE', *, *, #4466, .T. ) ;
#19765=CARTESIAN_POINT ( 'NONE',  ( 130.0000000000000000, 37.18007812608393436, -13.14518615778179544 ) ) ;
#19766=EDGE_CURVE ( 'NONE', #7806, #3638, #1635, .T. ) ;
#19767=CARTESIAN_POINT ( 'NONE',  ( 59.37712712842213136, 35.39414062716787157, -13.57481594606304753 ) ) ;
#19771=CARTESIAN_POINT ( 'NONE',  ( -13.57481594606304753, 33.11210937716786873, -5.622872871577873077 ) ) ;
#19775=CARTESIAN_POINT ( 'NONE',  ( 185.7049497278729575, 34.30273437608393294, 9.295050272127047819 ) ) ;
#19777=EDGE_CURVE ( 'NONE', #15169, #22062, #14821, .T. ) ;
#19779=CARTESIAN_POINT ( 'NONE',  ( 195.0000000000000000, 38.81718749999999574, 13.57481594606304576 ) ) ;
#19782=CARTESIAN_POINT ( 'NONE',  ( -8.312177448680279460E-16, 36.03906250000000000, -13.57481594606304576 ) ) ;
#19788=CARTESIAN_POINT ( 'NONE',  ( 208.5748159460630688, 35.04687499999999289, -1.662435489736055892E-15 ) ) ;
#19789=DIRECTION ( 'NONE',  ( -0.000000000000000000, 1.000000000000000000, -0.000000000000000000 ) ) ;
#19791=CARTESIAN_POINT ( 'NONE',  ( 51.85481384221820633, 35.84062500108394289, 5.444914386472304635 ) ) ;
#19794=DIRECTION ( 'NONE',  ( 0.000000000000000000, 0.000000000000000000, -1.000000000000000000 ) ) ;
#19795=CARTESIAN_POINT ( 'NONE',  ( -5.622872871577873077, 36.38632812499999858, 13.57481594606304753 ) ) ;
#19796=CARTESIAN_POINT ( 'NONE',  ( 143.1451861577818079, 36.33671875108394289, 5.444914386472293977 ) ) ;
#19797=EDGE_LOOP ( 'NONE', ( #26617, #26809, #23116, #4006 ) ) ;
#19799=CARTESIAN_POINT ( 'NONE',  ( 95.54126587499995082, 80.62500000136559208, -1.846868145590750077 ) ) ;
#19800=VECTOR ( 'NONE', #18890, 1000.000000000000000 ) ;
#19801=CARTESIAN_POINT ( 'NONE',  ( 102.0710678118654329, 80.43750000273119838, 4.999999999999989342 ) ) ;
#19803=CARTESIAN_POINT ( 'NONE',  ( 51.89752917827804168, 36.00000000000001421, -1.608626461598229085 ) ) ;
#19806=CARTESIAN_POINT ( 'NONE',  ( 59.55508561352770158, 32.96328125108393436, 13.14518615778179722 ) ) ;
#19811=VERTEX_POINT ( 'NONE', #10769 ) ;
#19815=CARTESIAN_POINT ( 'NONE',  ( 185.4011555911795313, 35.44375000216787441, -9.598844408820458085 ) ) ;
#19816=ORIENTED_EDGE ( 'NONE', *, *, #6824, .F. ) ;
#19819=CARTESIAN_POINT ( 'NONE',  ( 143.1451861577818079, 37.18007812608393436, -1.609821015232357215E-15 ) ) ;
#19820=CARTESIAN_POINT ( 'NONE',  ( -9.295050272127046043, 35.09648437608393579, -9.295050272127046043 ) ) ;
#19821=CARTESIAN_POINT ( 'NONE',  ( 143.1451861577818079, 36.13828125108393863, 5.444914386472293977 ) ) ;
#19822=CARTESIAN_POINT ( 'NONE',  ( 78.57481594606304043, 35.79101562499999289, 5.622872871577869525 ) ) ;
#19825=DIRECTION ( 'NONE',  ( -0.000000000000000000, 1.000000000000000000, -0.000000000000000000 ) ) ;
#19831=CARTESIAN_POINT ( 'NONE',  ( 9.295050272127046043, 38.07304687608393579, -9.295050272127046043 ) ) ;
#19838=CARTESIAN_POINT ( 'NONE',  ( 208.1451861577818079, 39.36289062608393152, -1.609821015232357215E-15 ) ) ;
#19840=CARTESIAN_POINT ( 'NONE',  ( 9.598844408820456309, 40.00781250216787299, -9.598844408820458085 ) ) ;
#19842=ORIENTED_EDGE ( 'NONE', *, *, #14023, .T. ) ;
#19847=CARTESIAN_POINT ( 'NONE',  ( 143.5748159460630688, 31.97109375216787441, -1.662435489736055892E-15 ) ) ;
#19850=CARTESIAN_POINT ( 'NONE',  ( 65.00000000000000000, 36.58476562608393579, -13.14518615778179544 ) ) ;
#19851=CARTESIAN_POINT ( 'NONE',  ( 66.13876811710015602, 50.00000000043813486, -13.56816686242498982 ) ) ;
#19852=CARTESIAN_POINT ( 'NONE',  ( 195.0000000000000000, 40.80156249999999574, -13.57481594606304576 ) ) ;
#19853=CARTESIAN_POINT ( 'NONE',  ( 75.56308295035979938, 36.00000000000000000, 8.196709705857863071 ) ) ;
#19859=CARTESIAN_POINT ( 'NONE',  ( 59.55508561352770158, 39.90859375108392726, 13.14518615778179722 ) ) ;
#19860=CARTESIAN_POINT ( 'NONE',  ( 65.00000000000000000, 36.53515625216787299, 13.57481594606304576 ) ) ;
#19861=CARTESIAN_POINT ( 'NONE',  ( 195.0000000000000000, 39.16445312608392726, 13.14518615778179544 ) ) ;
#19863=CARTESIAN_POINT ( 'NONE',  ( 185.8198241863519797, 50.00000000000000711, 14.99999999999995204 ) ) ;
#19865=CARTESIAN_POINT ( 'NONE',  ( 0.000000000000000000, 80.00000000000000000, 0.000000000000000000 ) ) ;
#19866=CARTESIAN_POINT ( 'NONE',  ( 70.62287287157774074, 39.66054687500000142, 13.57481594606318076 ) ) ;
#19869=EDGE_LOOP ( 'NONE', ( #25743, #17375, #14231, #21422, #20238, #21760 ) ) ;
#19873=CARTESIAN_POINT ( 'NONE',  ( 116.8548138422182063, 32.86406250108393579, 5.444914386472304635 ) ) ;
#19874=CARTESIAN_POINT ( 'NONE',  ( 78.14518615778179367, 34.65000000108393152, -5.444914386472297529 ) ) ;
#19875=CARTESIAN_POINT ( 'NONE',  ( 204.2950502721270425, 38.86679687608393863, -9.295050272127046043 ) ) ;
#19879=CARTESIAN_POINT ( 'NONE',  ( 13.14518615778179900, 32.16953125108393152, 5.444914386472293977 ) ) ;
#19883=CARTESIAN_POINT ( 'NONE',  ( 139.5988444088204687, 39.80937500216786873, 9.598844408820456309 ) ) ;
#19887=CARTESIAN_POINT ( 'NONE',  ( 56.73140267161080885, 50.00000000054374993, 10.78867689284317066 ) ) ;
#19889=EDGE_CURVE ( 'NONE', #444, #10089, #22134, .T. ) ;
#19890=FILL_AREA_STYLE ('',( #24735 ) ) ;
#19895=CARTESIAN_POINT ( 'NONE',  ( 127.8300434168938580, 49.99999999883939950, 13.43548448457867828 ) ) ;
#19897=CARTESIAN_POINT ( 'NONE',  ( 219.9999999999999716, 55.00000000000000000, 14.99999999999994316 ) ) ;
#19898=CARTESIAN_POINT ( 'NONE',  ( 101.8468681455906903, 82.37500000136562051, -4.458734125000016313 ) ) ;
#19899=CARTESIAN_POINT ( 'NONE',  ( 78.14518615778179367, 36.38632812608393863, -1.609821015232357215E-15 ) ) ;
#19901=CARTESIAN_POINT ( 'NONE',  ( 5.444914386472297529, 36.33671875108393579, -13.14518615778179722 ) ) ;
#19907=CARTESIAN_POINT ( 'NONE',  ( 120.4011555911795455, 38.51953124999999289, -9.598844408820458085 ) ) ;
#19914=CARTESIAN_POINT ( 'NONE',  ( 143.1451861577818079, 35.39414062608393152, -1.609821015232357215E-15 ) ) ;
#19915=CARTESIAN_POINT ( 'NONE',  ( 51.42518405393695957, 33.21132812716787441, 5.622872871577880183 ) ) ;
#19917=CARTESIAN_POINT ( 'NONE',  ( 5.622872871577878406, 32.61601562716786873, 13.57481594606304576 ) ) ;
#19920=ADVANCED_FACE ( 'NONE', ( #15180 ), #17192, .F. ) ;
#19921=CARTESIAN_POINT ( 'NONE',  ( 181.8548138422181921, 34.94765625108392726, -5.444914386472297529 ) ) ;
#19923=CARTESIAN_POINT ( 'NONE',  ( 99.99999999999995737, 81.75000000000000000, -5.000000000000018652 ) ) ;
#19924=ORIENTED_EDGE ( 'NONE', *, *, #20278, .T. ) ;
#19925=CARTESIAN_POINT ( 'NONE',  ( 189.3771271284221029, 40.35507812499999147, 13.57481594606302444 ) ) ;
#19926=CARTESIAN_POINT ( 'NONE',  ( 120.4011555911795455, 36.23750000216787726, -9.598844408820458085 ) ) ;
#19933=CARTESIAN_POINT ( 'NONE',  ( 189.3771271284221314, 33.21132812499999432, 13.57481594606304753 ) ) ;
#19935=CARTESIAN_POINT ( 'NONE',  ( 59.37712712842210294, 40.35507812499999147, 13.57481594606302444 ) ) ;
#19937=CARTESIAN_POINT ( 'NONE',  ( 65.00000000000000000, 36.38632812608393152, -13.14518615778179544 ) ) ;
#19938=ADVANCED_FACE ( 'NONE', ( #23899 ), #15616, .T. ) ;
#19942=CARTESIAN_POINT ( 'NONE',  ( -9.598844408820454532, 36.33671874999999574, 9.598844408820459861 ) ) ;
#19943=CARTESIAN_POINT ( 'NONE',  ( 135.4449143864723055, 38.91640625108393436, -13.14518615778179900 ) ) ;
#19946=CARTESIAN_POINT ( 'NONE',  ( 99.99999999999995737, 82.75000000000000000, -5.000000000000018652 ) ) ;
#19947=LINE ( 'NONE', #425, #23034 ) ;
#19948=CARTESIAN_POINT ( 'NONE',  ( 99.99999999999995737, 83.87500000273119838, -5.000000000000018652 ) ) ;
#19950=DIRECTION ( 'NONE',  ( 0.000000000000000000, 0.000000000000000000, 1.000000000000000000 ) ) ;
#19951=VECTOR ( 'NONE', #20859, 1000.000000000000000 ) ;
#19954=CARTESIAN_POINT ( 'NONE',  ( 59.55508561352770158, 31.87187500108393223, -13.14518615778179900 ) ) ;
#19957=LINE ( 'NONE', #20239, #22256 ) ;
#19961=CARTESIAN_POINT ( 'NONE',  ( 181.4251840539369596, 34.69960937716787441, -5.622872871577873077 ) ) ;
#19962=( BOUNDED_CURVE ( )  B_SPLINE_CURVE ( 2, ( #25105, #26835, #9849, #12110, #11546, #16409, #14116, #18556, #20838 ),
 .UNSPECIFIED., .F., .T. ) 
 B_SPLINE_CURVE_WITH_KNOTS ( ( 3, 2, 2, 2, 3 ),
 ( 0.3125000000000002220, 0.3229166666666668517, 0.3333333333333334259, 0.3437500000000000555, 0.3541666666666666852 ),
 .UNSPECIFIED. ) 
 CURVE ( )  GEOMETRIC_REPRESENTATION_ITEM ( )  RATIONAL_B_SPLINE_CURVE ( ( 0.9999999999999983347, 0.9238795325112884038, 1.000000000000000000, 0.9238795325112867385, 1.000000000000000000, 0.9238795325112867385, 1.000000000000000000, 0.9238795325112867385, 1.000000000000000000 ) ) 
 REPRESENTATION_ITEM ( '' )  );
#19964=CARTESIAN_POINT ( 'NONE',  ( -8.312177448680279460E-16, 40.80156249999999574, -13.57481594606304576 ) ) ;
#19966=CARTESIAN_POINT ( 'NONE',  ( 124.5550856135277087, 37.72578125108394431, 13.14518615778179722 ) ) ;
#19967=CARTESIAN_POINT ( 'NONE',  ( 5.444914386472302859, 34.65000000108393863, 13.14518615778179189 ) ) ;
#19968=CARTESIAN_POINT ( 'NONE',  ( 124.5550856135277087, 32.76484375108393010, 13.14518615778179722 ) ) ;
#19969=CARTESIAN_POINT ( 'NONE',  ( 70.62287287157786864, 35.19570312499999432, -13.57481594606304753 ) ) ;
#19971=AXIS2_PLACEMENT_3D ( 'NONE', #19202, #3549, #25615 ) ;
#19972=VECTOR ( 'NONE', #24869, 1000.000000000000000 ) ;
#19974=DIRECTION ( 'NONE',  ( -1.000000000000000000, 0.000000000000000000, 7.228014483236696740E-18 ) ) ;
#19977=VECTOR ( 'NONE', #7839, 1000.000000000000000 ) ;
#19979=CARTESIAN_POINT ( 'NONE',  ( 65.00000000000000000, 50.00000000000000000, -7.517135062566165128E-15 ) ) ;
#19981=CARTESIAN_POINT ( 'NONE',  ( 13.14518615778179544, 35.59257812608393579, -1.609821015232357215E-15 ) ) ;
#19982=EDGE_CURVE ( 'NONE', #2100, #12289, #6716, .T. ) ;
#19984=VERTEX_POINT ( 'NONE', #21770 ) ;
#19988=CARTESIAN_POINT ( 'NONE',  ( 189.5550856135277229, 36.43593750108392726, -13.14518615778179900 ) ) ;
#19997=VECTOR ( 'NONE', #11258, 1000.000000000000000 ) ;
#19998=CARTESIAN_POINT ( 'NONE',  ( 143.5748159460630404, 32.02070312716787015, -5.622872871577873077 ) ) ;
#19999=DIRECTION ( 'NONE',  ( 0.000000000000000000, 0.000000000000000000, 1.000000000000000000 ) ) ;
#20001=CARTESIAN_POINT ( 'NONE',  ( 59.55508561352770158, 36.63437500108393152, -13.14518615778179900 ) ) ;
#20002=CARTESIAN_POINT ( 'NONE',  ( 73.75833439235653088, 50.00000000000000000, -10.38725784494184445 ) ) ;
#20004=CARTESIAN_POINT ( 'NONE',  ( 181.8548138422182205, 32.02070312608393010, 0.000000000000000000 ) ) ;
#20005=ADVANCED_FACE ( 'NONE', ( #27041 ), #13892, .T. ) ;
#20006=FACE_OUTER_BOUND ( 'NONE', #15743, .T. ) ;
#20012=CARTESIAN_POINT ( 'NONE',  ( 208.1451861577818079, 39.36289062608393152, -1.609821015232357215E-15 ) ) ;
#20017=CARTESIAN_POINT ( 'NONE',  ( 195.0000000000000000, 36.58476562608393579, -13.14518615778179544 ) ) ;
#20019=ORIENTED_EDGE ( 'NONE', *, *, #2565, .F. ) ;
#20022=ORIENTED_EDGE ( 'NONE', *, *, #7333, .F. ) ;
#20023=CARTESIAN_POINT ( 'NONE',  ( 143.1451861577818079, 32.46718750108393436, -5.444914386472297529 ) ) ;
#20024=CARTESIAN_POINT ( 'NONE',  ( 70.44491438647230552, 32.86406250108392868, 13.14518615778179189 ) ) ;
#20026=CARTESIAN_POINT ( 'NONE',  ( 195.0000000000000000, 36.18789062608393436, 13.14518615778179544 ) ) ;
#20029=CARTESIAN_POINT ( 'NONE',  ( -5.444914386472297529, 33.26093750108393721, -13.14518615778179900 ) ) ;
#20030=CARTESIAN_POINT ( 'NONE',  ( 121.2451010467541010, 50.00000000000000000, -10.39041163855918981 ) ) ;
#20031=CARTESIAN_POINT ( 'NONE',  ( 135.6228728715778971, 39.75976562716787299, 13.57481594606304576 ) ) ;
#20035=CARTESIAN_POINT ( 'NONE',  ( 204.2950502721270425, 39.66054687608393436, -9.295050272127046043 ) ) ;
#20042=CARTESIAN_POINT ( 'NONE',  ( 138.7548989532463395, 50.00000000000000000, 10.39041163855194050 ) ) ;
#20044=CARTESIAN_POINT ( 'NONE',  ( -5.622872871578011633, 38.86679687716787868, 13.57481594606290720 ) ) ;
#20045=CARTESIAN_POINT ( 'NONE',  ( -12.37587840034927744, 36.00000000000000000, 4.513979326318477980 ) ) ;
#20046=CARTESIAN_POINT ( 'NONE',  ( 74.29505027212704249, 35.49335937608393721, 9.295050272127046043 ) ) ;
#20047=CARTESIAN_POINT ( 'NONE',  ( 181.4251840539369596, 37.77539062499998579, -5.622872871577872189 ) ) ;
#20048=CARTESIAN_POINT ( 'NONE',  ( 13.14518615778179544, 39.36289062608393152, -1.609821015232357215E-15 ) ) ;
#20051=CARTESIAN_POINT ( 'NONE',  ( 3.636496246807550126, 51.46815297079190543, 14.99999999999999467 ) ) ;
#20053=CARTESIAN_POINT ( 'NONE',  ( 116.4251840539369596, 37.87460937499999147, 5.622872871577880183 ) ) ;
#20054=ORIENTED_EDGE ( 'NONE', *, *, #11427, .T. ) ;
#20055=DIRECTION ( 'NONE',  ( 1.000000000000000000, 0.000000000000000000, -1.156482317317871478E-16 ) ) ;
#20059=CARTESIAN_POINT ( 'NONE',  ( 120.7049497278729575, 31.92148437608393508, 9.295050272127047819 ) ) ;
#20060=CARTESIAN_POINT ( 'NONE',  ( 55.40115559117954547, 34.05468750216788010, 9.598844408820459861 ) ) ;
#20063=CARTESIAN_POINT ( 'NONE',  ( 55.40115559117954547, 37.22968750216787726, 9.598844408820459861 ) ) ;
#20064=CARTESIAN_POINT ( 'NONE',  ( 2.493653234604083739E-15, 33.36015625216786873, 13.57481594606304576 ) ) ;
#20066=CARTESIAN_POINT ( 'NONE',  ( 97.92893218813449607, 84.81250000000000000, -5.000000000000020428 ) ) ;
#20067=AXIS2_PLACEMENT_3D ( 'NONE', #3947, #14613, #20778 ) ;
#20069=CARTESIAN_POINT ( 'NONE',  ( 204.2950502721270425, 32.91367187608393152, 9.295050272127046043 ) ) ;
#20070=DIRECTION ( 'NONE',  ( 0.000000000000000000, 0.000000000000000000, 1.000000000000000000 ) ) ;
#20073=DIRECTION ( 'NONE',  ( -0.000000000000000000, 1.000000000000000000, -0.000000000000000000 ) ) ;
#20077=CARTESIAN_POINT ( 'NONE',  ( 65.00000000000000000, -7.395377635281828788, 11.57481594606303688 ) ) ;
#20080=CARTESIAN_POINT ( 'NONE',  ( 189.3771271284221314, 34.00507812499999716, 13.57481594606304753 ) ) ;
#20081=VECTOR ( 'NONE', #19358, 1000.000000000000000 ) ;
#20085=CARTESIAN_POINT ( 'NONE',  ( 65.00000000000000000, 36.78320312608393294, 13.14518615778179544 ) ) ;
#20089=CARTESIAN_POINT ( 'NONE',  ( -13.57481594606304576, 35.44374999999999432, 0.000000000000000000 ) ) ;
#20090=CARTESIAN_POINT ( 'NONE',  ( 124.5550856135277087, 37.72578125108395142, 13.14518615778179722 ) ) ;
#20092=CARTESIAN_POINT ( 'NONE',  ( 102.0710678118654329, 80.68750000000001421, -5.000000000000018652 ) ) ;
#20095=CARTESIAN_POINT ( 'NONE',  ( 103.5355339059327093, 81.75000000273119838, -3.535533905932755072 ) ) ;
#20100=CARTESIAN_POINT ( 'NONE',  ( 78.14518615778179367, 32.41757812608393863, -1.609821015232357215E-15 ) ) ;
#20102=DIRECTION ( 'NONE',  ( -0.000000000000000000, 1.000000000000000000, -0.000000000000000000 ) ) ;
#20104=EDGE_CURVE ( 'NONE', #27809, #9474, #13749, .T. ) ;
#20105=EDGE_LOOP ( 'NONE', ( #19020, #14196 ) ) ;
#20107=CARTESIAN_POINT ( 'NONE',  ( 181.4251840539369596, 33.11210937716786873, -5.622872871577873077 ) ) ;
#20111=CARTESIAN_POINT ( 'NONE',  ( 0.000000000000000000, -7.395377635281828788, 13.57481594606304398 ) ) ;
#20112=CARTESIAN_POINT ( 'NONE',  ( -13.14518615778179189, 33.65781250108393152, 5.444914386472304635 ) ) ;
#20113=CARTESIAN_POINT ( 'NONE',  ( 135.4449143864723055, 32.07031250108393294, 13.14518615778179189 ) ) ;
#20114=CARTESIAN_POINT ( 'NONE',  ( 70.62287287157788285, 33.31054687499999289, 13.57481594606304576 ) ) ;
#20115=CARTESIAN_POINT ( 'NONE',  ( -20.00000000000000355, 80.00000000000000000, -14.99999999999999822 ) ) ;
#20117=CARTESIAN_POINT ( 'NONE',  ( 95.54126587499996504, 84.43750000136560629, -1.387778780781445676E-14 ) ) ;
#20123=CARTESIAN_POINT ( 'NONE',  ( -13.14518615778179544, 36.78320312608393294, 0.000000000000000000 ) ) ;
#20124=ORIENTED_EDGE ( 'NONE', *, *, #26766, .F. ) ;
#20126=CARTESIAN_POINT ( 'NONE',  ( 96.46446615806316061, 80.00000000000000000, -3.535533969928681852 ) ) ;
#20128=CARTESIAN_POINT ( 'NONE',  ( 200.4449143864723055, 36.03906250108394005, 13.14518615778179189 ) ) ;
#20130=EDGE_LOOP ( 'NONE', ( #21284, #3677, #17460, #13071 ) ) ;
#20132=CARTESIAN_POINT ( 'NONE',  ( 185.8198241863519513, 55.00000000000000000, -15.00000000000000000 ) ) ;
#20134=VERTEX_POINT ( 'NONE', #819 ) ;
#20139=CARTESIAN_POINT ( 'NONE',  ( 139.2950502721270425, 36.88242187608393152, 9.295050272127046043 ) ) ;
#20141=CARTESIAN_POINT ( 'NONE',  ( -13.14518615778179900, 36.53515625108392584, -5.444914386472297529 ) ) ;
#20143=CARTESIAN_POINT ( 'NONE',  ( 70.44491438647230552, 38.12265625108393152, -13.14518615778179900 ) ) ;
#20144=CARTESIAN_POINT ( 'NONE',  ( 56.24510104675918853, 50.00000000000000000, -10.39041163855703864 ) ) ;
#20146=VECTOR ( 'NONE', #27209, 1000.000000000000000 ) ;
#20147=CARTESIAN_POINT ( 'NONE',  ( 204.2950502721270425, 32.51679687608393721, -9.295050272127046043 ) ) ;
#20149=CARTESIAN_POINT ( 'NONE',  ( 77.89215161363580364, 36.00000000000001421, -4.169510824906851987 ) ) ;
#20153=DIRECTION ( 'NONE',  ( -1.000000000000000000, 0.000000000000000000, 7.228014483236696740E-18 ) ) ;
#20155=ORIENTED_EDGE ( 'NONE', *, *, #20539, .T. ) ;
#20158=CARTESIAN_POINT ( 'NONE',  ( 189.5550856135277229, 39.01562500108394005, -13.14518615778179722 ) ) ;
#20160=VERTEX_POINT ( 'NONE', #9487 ) ;
#20164=CARTESIAN_POINT ( 'NONE',  ( 143.1451861577818079, 34.05468750108394005, -5.444914386472297529 ) ) ;
#20165=CARTESIAN_POINT ( 'NONE',  ( 59.55508561352770158, 31.67343750108393863, -13.14518615778179900 ) ) ;
#20166=AXIS2_PLACEMENT_3D ( 'NONE', #3327, #12696, #25681 ) ;
#20167=CARTESIAN_POINT ( 'NONE',  ( 200.4449143864723055, 33.85625000108393579, 13.14518615778179189 ) ) ;
#20170=CARTESIAN_POINT ( 'NONE',  ( 1.947325922083074978, 51.47162402671164472, -14.99999999999802114 ) ) ;
#20173=DIRECTION ( 'NONE',  ( 0.000000000000000000, 0.000000000000000000, -1.000000000000000000 ) ) ;
#20177=EDGE_LOOP ( 'NONE', ( #23522, #18849, #26217, #18717 ) ) ;
#20182=CARTESIAN_POINT ( 'NONE',  ( 195.0000000000000000, 39.31328125216787583, -13.57481594606304576 ) ) ;
#20184=CARTESIAN_POINT ( 'NONE',  ( -12.05655202970026885, 36.00000000000000000, 5.307619621752119876 ) ) ;
#20185=CYLINDRICAL_SURFACE ( 'NONE', #26257, 5.000000000000000000 ) ;
#20188=CARTESIAN_POINT ( 'NONE',  ( 13.14518615778179722, 38.61875000108392442, -5.444914386472297529 ) ) ;
#20190=CARTESIAN_POINT ( 'NONE',  ( 195.0000000000000000, 39.61093749999999147, 13.57481594606304576 ) ) ;
#20192=CARTESIAN_POINT ( 'NONE',  ( 135.6228728715778686, 38.37070312499999147, -13.57481594606304753 ) ) ;
#20193=ORIENTED_EDGE ( 'NONE', *, *, #15778, .T. ) ;
#20198=CARTESIAN_POINT ( 'NONE',  ( 116.8548138422182063, 33.45937500108392726, 5.444914386472304635 ) ) ;
#20199=CARTESIAN_POINT ( 'NONE',  ( 70.44491438647230552, 39.21406250108392300, 13.14518615778179189 ) ) ;
#20200=CARTESIAN_POINT ( 'NONE',  ( 13.57481594606304576, 31.97109375216787441, -1.662435489736055892E-15 ) ) ;
#20204=CARTESIAN_POINT ( 'NONE',  ( 189.5550856135277229, 33.55859375108393294, 13.14518615778179722 ) ) ;
#20208=CARTESIAN_POINT ( 'NONE',  ( -15.00000000000000355, 55.00000000000000000, -9.999999999999998224 ) ) ;
#20214=( BOUNDED_CURVE ( )  B_SPLINE_CURVE ( 2, ( #27230, #7826, #5273, #18665, #23082, #9678, #11659, #18238, #9950 ),
 .UNSPECIFIED., .F., .F. ) 
 B_SPLINE_CURVE_WITH_KNOTS ( ( 3, 2, 2, 2, 3 ),
 ( 0.3541666666666666852, 0.3645833333333332593, 0.3749999999999998890, 0.3854166666666665741, 0.3958333333333331483 ),
 .UNSPECIFIED. ) 
 CURVE ( )  GEOMETRIC_REPRESENTATION_ITEM ( )  RATIONAL_B_SPLINE_CURVE ( ( 1.000000000000000000, 0.9238795325112867385, 1.000000000000000000, 0.9238795325112867385, 1.000000000000000000, 0.9238795325112867385, 1.000000000000000000, 0.9238795325112879597, 0.9999999999999987788 ) ) 
 REPRESENTATION_ITEM ( '' )  );
#20219=CARTESIAN_POINT ( 'NONE',  ( 9.598844408820456309, 36.73359374999999716, -9.598844408820458085 ) ) ;
#20220=CARTESIAN_POINT ( 'NONE',  ( 104.4587341249999781, 83.87500000136560629, 1.846868145590721655 ) ) ;
#20221=CARTESIAN_POINT ( 'NONE',  ( 55.70494972787295751, 33.31054687608393294, -9.295050272127046043 ) ) ;
#20224=LINE ( 'NONE', #22364, #12724 ) ;
#20227=SPHERICAL_SURFACE ( 'NONE', #1769, 5.000000000000000000 ) ;
#20228=CARTESIAN_POINT ( 'NONE',  ( 120.7049497278729575, 36.88242187608393152, 9.295050272127047819 ) ) ;
#20230=LINE ( 'NONE', #15935, #1372 ) ;
#20232=CARTESIAN_POINT ( 'NONE',  ( 103.1528011352953342, 82.81250000136560629, 3.152801135295355106 ) ) ;
#20235=VECTOR ( 'NONE', #2605, 999.9999999999998863 ) ;
#20237=CARTESIAN_POINT ( 'NONE',  ( 51.85481384221820633, 32.02070312608393010, 0.000000000000000000 ) ) ;
#20238=ORIENTED_EDGE ( 'NONE', *, *, #1788, .T. ) ;
#20239=CARTESIAN_POINT ( 'NONE',  ( 0.000000000000000000, -7.395377635281828788, 13.57481594606304398 ) ) ;
#20241=EDGE_LOOP ( 'NONE', ( #15423, #20443, #24503, #16383, #15554, #2146, #14858, #362, #18519, #11269, #21642, #18870, #24377, #753 ) ) ;
#20243=CARTESIAN_POINT ( 'NONE',  ( 195.0000000000000000, 34.55078125216787299, -13.57481594606304576 ) ) ;
#20246=CARTESIAN_POINT ( 'NONE',  ( -13.14518615778179900, 33.55859375108393294, -5.444914386472297529 ) ) ;
#20250=DIRECTION ( 'NONE',  ( 1.000000000000000000, 0.000000000000000000, -0.000000000000000000 ) ) ;
#20252=CARTESIAN_POINT ( 'NONE',  ( 195.0000000000000000, -7.395377635281828788, 13.57481594606302266 ) ) ;
#20260=CARTESIAN_POINT ( 'NONE',  ( 5.444914386472302859, 34.65000000108393863, 13.14518615778179189 ) ) ;
#20261=VERTEX_POINT ( 'NONE', #1102 ) ;
#20262=CARTESIAN_POINT ( 'NONE',  ( 116.4251840539369596, 37.03124999999999289, 0.000000000000000000 ) ) ;
#20265=CYLINDRICAL_SURFACE ( 'NONE', #21593, 5.000000000000004441 ) ;
#20266=CARTESIAN_POINT ( 'NONE',  ( 204.2950502721270425, 36.88242187608393152, 9.295050272127046043 ) ) ;
#20272=AXIS2_PLACEMENT_3D ( 'NONE', #28063, #4258, #12503 ) ;
#20275=CARTESIAN_POINT ( 'NONE',  ( 139.2950502721270425, 38.66835937608393436, -9.295050272127046043 ) ) ;
#20276=CARTESIAN_POINT ( 'NONE',  ( -13.14518615778179544, 38.37070312608393152, 0.000000000000000000 ) ) ;
#20277=CARTESIAN_POINT ( 'NONE',  ( 2.414731522848535132E-15, 34.40195312608393152, 13.14518615778179544 ) ) ;
#20278=EDGE_CURVE ( 'NONE', #13933, #13505, #22333, .T. ) ;
#20280=VECTOR ( 'NONE', #13212, 1000.000000000000000 ) ;
#20282=CARTESIAN_POINT ( 'NONE',  ( 208.1451861577818079, 32.41757812608393863, -1.609821015232357215E-15 ) ) ;
#20284=CARTESIAN_POINT ( 'NONE',  ( 67.23232715533710291, 35.99999999999999289, 12.98409812936893104 ) ) ;
#20289=CARTESIAN_POINT ( 'NONE',  ( 59.55508561352770158, 37.52734375108393294, 13.14518615778179722 ) ) ;
#20292=ORIENTED_EDGE ( 'NONE', *, *, #3063, .T. ) ;
#20293=EDGE_CURVE ( 'NONE', #4709, #26902, #4092, .T. ) ;
#20297=CARTESIAN_POINT ( 'NONE',  ( 208.1451861577818079, 37.18007812608393436, -1.609821015232357215E-15 ) ) ;
#20299=ADVANCED_FACE ( 'NONE', ( #18751 ), #25159, .T. ) ;
#20303=AXIS2_PLACEMENT_3D ( 'NONE', #5227, #14038, #3088 ) ;
#20305=CARTESIAN_POINT ( 'NONE',  ( 135.4449143864723055, 32.56640625108394005, -13.14518615778179900 ) ) ;
#20307=CARTESIAN_POINT ( 'NONE',  ( 181.8548138422181921, 33.55859375108393294, -5.444914386472297529 ) ) ;
#20312=CARTESIAN_POINT ( 'NONE',  ( 143.5748159460630404, 36.68398437716788152, 5.622872871577869525 ) ) ;
#20316=CARTESIAN_POINT ( 'NONE',  ( 74.18017581364802027, 55.00000000000001421, 14.99999999999997691 ) ) ;
#20317=EDGE_CURVE ( 'NONE', #1074, #15490, #25579, .T. ) ;
#20324=CARTESIAN_POINT ( 'NONE',  ( 200.6228728715777834, 38.37070312499999858, -13.57481594606313990 ) ) ;
#20327=CARTESIAN_POINT ( 'NONE',  ( 68.75563991928589758, 31.78804746655075419, -13.14518615778179544 ) ) ;
#20330=CARTESIAN_POINT ( 'NONE',  ( 2.414731522848535132E-15, 37.57695312608392868, 13.14518615778179544 ) ) ;
#20333=CARTESIAN_POINT ( 'NONE',  ( -7.636241067998421173, 54.91786508990982441, 14.99999999999999822 ) ) ;
#20335=CARTESIAN_POINT ( 'NONE',  ( 124.3771271284221314, 34.50117187499999005, -13.57481594606304753 ) ) ;
#20338=ORIENTED_EDGE ( 'NONE', *, *, #17196, .T. ) ;
#20342=AXIS2_PLACEMENT_3D ( 'NONE', #17961, #4719, #879 ) ;
#20344=CARTESIAN_POINT ( 'NONE',  ( 135.4449143864723055, 34.74921875108394431, -13.14518615778179900 ) ) ;
#20345=CARTESIAN_POINT ( 'NONE',  ( 59.55508561352770158, 39.11484375108394573, 13.14518615778179722 ) ) ;
#20346=CARTESIAN_POINT ( 'NONE',  ( 65.00000000000000000, 37.32890625216786873, 13.57481594606304576 ) ) ;
#20347=CARTESIAN_POINT ( 'NONE',  ( 5.444914386472297529, 38.71796875108393721, -13.14518615778179900 ) ) ;
#20353=CARTESIAN_POINT ( 'NONE',  ( 208.1451861577817795, 32.26875000108393721, -5.444914386472297529 ) ) ;
#20354=CARTESIAN_POINT ( 'NONE',  ( 195.0000000000000000, -7.395377635281828788, -2.255140518769849538E-14 ) ) ;
#20356=CARTESIAN_POINT ( 'NONE',  ( 200.6228728715779255, 38.86679687500001279, 13.57481594606301023 ) ) ;
#20357=CARTESIAN_POINT ( 'NONE',  ( 116.4251840539369738, 36.38632812716788578, 5.622872871577880183 ) ) ;
#20364=CARTESIAN_POINT ( 'NONE',  ( 208.5748159460630120, 32.61601562499999574, 5.622872871577869525 ) ) ;
#20367=CARTESIAN_POINT ( 'NONE',  ( 130.0000000000000000, 50.00000000000000000, -1.503427012513233026E-14 ) ) ;
#20368=FACE_OUTER_BOUND ( 'NONE', #13654, .T. ) ;
#20369=CARTESIAN_POINT ( 'NONE',  ( 78.14518615778179367, 32.96328125108393436, 5.444914386472293977 ) ) ;
#20374=CARTESIAN_POINT ( 'NONE',  ( 13.57481594606304931, 32.61601562499999574, 5.622872871577869525 ) ) ;
#20375=CARTESIAN_POINT ( 'NONE',  ( 124.5550856135277087, 35.04687500108393294, -13.14518615778179900 ) ) ;
#20377=CARTESIAN_POINT ( 'NONE',  ( 104.9999999999999716, 80.50000000000000000, -1.449011120738813565E-14 ) ) ;
#20379=CARTESIAN_POINT ( 'NONE',  ( 102.0710678118654329, 79.43750000273119838, 4.999999999999989342 ) ) ;
#20381=CARTESIAN_POINT ( 'NONE',  ( 74.59884440882045453, 39.01562500216787299, 9.598844408820456309 ) ) ;
#20383=CARTESIAN_POINT ( 'NONE',  ( 59.55508561352770158, 32.16953125108393152, 13.14518615778179722 ) ) ;
#20384=CARTESIAN_POINT ( 'NONE',  ( -5.622872871577873077, 37.77539062716788010, -13.57481594606304753 ) ) ;
#20385=VERTEX_POINT ( 'NONE', #10874 ) ;
#20386=CARTESIAN_POINT ( 'NONE',  ( 198.0892609137967497, 36.00000000000000000, -13.21136010216380718 ) ) ;
#20390=CARTESIAN_POINT ( 'NONE',  ( 181.4251840539369596, 32.31835937716786589, -5.622872871577873077 ) ) ;
#20395=DIRECTION ( 'NONE',  ( 0.000000000000000000, 0.000000000000000000, -1.000000000000000000 ) ) ;
#20396=CARTESIAN_POINT ( 'NONE',  ( -13.14518615778179544, 35.19570312608393436, 0.000000000000000000 ) ) ;
#20397=CARTESIAN_POINT ( 'NONE',  ( 143.1451861577818079, 33.01289062608393010, -1.609821015232357215E-15 ) ) ;
#20408=CARTESIAN_POINT ( 'NONE',  ( -20.00000000000000000, 55.00000000000000000, 15.00000000000000178 ) ) ;
#20409=CARTESIAN_POINT ( 'NONE',  ( -13.14518615778179900, 32.76484375108393010, -5.444914386472297529 ) ) ;
#20414=CARTESIAN_POINT ( 'NONE',  ( 200.4449143864723055, 36.83281250108392868, 13.14518615778179189 ) ) ;
#20416=CARTESIAN_POINT ( 'NONE',  ( 202.6362410680037272, 54.91786508990981019, -15.00000000000000355 ) ) ;
#20423=DIRECTION ( 'NONE',  ( -1.000000000000000000, 0.000000000000000000, 2.385244779468110248E-16 ) ) ;
#20425=CIRCLE ( 'NONE', #13557, 13.57481594606304398 ) ;
#20426=CARTESIAN_POINT ( 'NONE',  ( 139.2950502721270425, 37.87460937608393152, -9.295050272127046043 ) ) ;
#20427=CARTESIAN_POINT ( 'NONE',  ( -9.295050272127044266, 39.26367187608393294, 9.295050272127047819 ) ) ;
#20428=CARTESIAN_POINT ( 'NONE',  ( -5.444914386472299306, 35.14609375108393152, 13.14518615778179722 ) ) ;
#20431=CARTESIAN_POINT ( 'NONE',  ( 60.14150070953499494, 49.99999999891522862, -12.70434618648778446 ) ) ;
#20434=LINE ( 'NONE', #916, #27170 ) ;
#20435=( BOUNDED_CURVE ( )  B_SPLINE_CURVE ( 2, ( #5649, #10038, #24889, #18750, #27450, #1101, #25299, #14454, #23171 ),
 .UNSPECIFIED., .F., .F. ) 
 B_SPLINE_CURVE_WITH_KNOTS ( ( 3, 2, 2, 2, 3 ),
 ( 0.7500000000000006661, 0.7750000000000006883, 0.8000000000000007105, 0.8250000000000007327, 0.8500000000000007550 ),
 .UNSPECIFIED. ) 
 CURVE ( )  GEOMETRIC_REPRESENTATION_ITEM ( )  RATIONAL_B_SPLINE_CURVE ( ( 0.9999999999999980016, 0.9238795325112887369, 1.000000000000000000, 0.9238795325112867385, 1.000000000000000000, 0.9238795325112867385, 1.000000000000000000, 0.9238795325112844070, 1.000000000000002442 ) ) 
 REPRESENTATION_ITEM ( '' )  );
#20438=CARTESIAN_POINT ( 'NONE',  ( 65.00000000000000000, 37.18007812608393436, -13.14518615778179544 ) ) ;
#20440=CARTESIAN_POINT ( 'NONE',  ( 200.4449143864723055, 37.13046875108393152, -13.14518615778179722 ) ) ;
#20443=ORIENTED_EDGE ( 'NONE', *, *, #112, .T. ) ;
#20446=CARTESIAN_POINT ( 'NONE',  ( 208.1451861577818079, 39.56132812608393579, -1.609821015232357215E-15 ) ) ;
#20451=ORIENTED_EDGE ( 'NONE', *, *, #23264, .T. ) ;
#20452=CARTESIAN_POINT ( 'NONE',  ( 130.0000000000000000, 34.20351562608394147, -13.14518615778179544 ) ) ;
#20453=CARTESIAN_POINT ( 'NONE',  ( 130.0000000000000000, 36.93203125216787441, -13.57481594606304576 ) ) ;
#20454=CARTESIAN_POINT ( 'NONE',  ( 208.1451861577818079, 33.21132812608393436, -1.609821015232357215E-15 ) ) ;
#20459=CARTESIAN_POINT ( 'NONE',  ( 120.4011555911795455, 37.82500000216787583, -9.598844408820458085 ) ) ;
#20461=ADVANCED_FACE ( 'NONE', ( #26287, #15005 ), #4201, .F. ) ;
#20464=CARTESIAN_POINT ( 'NONE',  ( 67.02462772553560910, 50.00000000050971494, 13.43320860980923115 ) ) ;
#20466=ORIENTED_EDGE ( 'NONE', *, *, #5336, .F. ) ;
#20471=CARTESIAN_POINT ( 'NONE',  ( 1.464337720320554093, 36.00000000000002842, -13.46163418879032037 ) ) ;
#20474=AXIS2_PLACEMENT_3D ( 'NONE', #18115, #7275, #2736 ) ;
#20475=ADVANCED_FACE ( 'NONE', ( #8749 ), #4065, .T. ) ;
#20477=CARTESIAN_POINT ( 'NONE',  ( 65.00000000000000000, 32.61601562608393579, -13.14518615778179544 ) ) ;
#20478=CARTESIAN_POINT ( 'NONE',  ( 195.0000000000000000, 38.02343749999999289, 13.57481594606304576 ) ) ;
#20479=CARTESIAN_POINT ( 'NONE',  ( 9.598844408820456309, 40.70234374999999716, -9.598844408820458085 ) ) ;
#20481=CARTESIAN_POINT ( 'NONE',  ( -1.947325922082419059, 51.47162402670901571, 14.99999999999934452 ) ) ;
#20483=CARTESIAN_POINT ( 'NONE',  ( 139.5988444088204403, 33.55859375000000000, -9.598844408820458085 ) ) ;
#20489=CARTESIAN_POINT ( 'NONE',  ( 124.5550856135277087, 34.84843750108393579, -13.14518615778179900 ) ) ;
#20490=CARTESIAN_POINT ( 'NONE',  ( 78.14518615778179367, 40.10703125108393152, 5.444914386472293977 ) ) ;
#20491=CARTESIAN_POINT ( 'NONE',  ( 99.99999999999995737, 80.25000000000000000, 4.999999999999990230 ) ) ;
#20492=CARTESIAN_POINT ( 'NONE',  ( -9.295050272127046043, 37.27929687608393294, -9.295050272127046043 ) ) ;
#20495=CARTESIAN_POINT ( 'NONE',  ( 214.9999999999999716, 80.00000000000000000, -10.00000000000000000 ) ) ;
#20498=CARTESIAN_POINT ( 'NONE',  ( 189.5550856135277229, 31.67343750108393863, -13.14518615778179900 ) ) ;
#20500=LINE ( 'NONE', #14199, #1426 ) ;
#20501=ADVANCED_FACE ( 'NONE', ( #21589 ), #21452, .T. ) ;
#20502=CARTESIAN_POINT ( 'NONE',  ( -20.00000000000000355, 55.00000000000000000, -9.999999999999998224 ) ) ;
#20510=EDGE_CURVE ( 'NONE', #778, #7715, #21877, .T. ) ;
#20514=CARTESIAN_POINT ( 'NONE',  ( 51.85481384221820633, 33.45937500108392726, 5.444914386472304635 ) ) ;
#20518=CARTESIAN_POINT ( 'NONE',  ( -13.57481594606304576, 34.64999999999999147, 0.000000000000000000 ) ) ;
#20520=CARTESIAN_POINT ( 'NONE',  ( 143.1451861577818079, 33.16171875108393863, 5.444914386472293977 ) ) ;
#20521=B_SPLINE_CURVE_WITH_KNOTS ( 'NONE', 3,
 ( #21053, #3672, #1537, #8068, #18900, #1122, #5670, #23053, #3802, #12334, #27205, #16763, #5534, #5390, #14335, #12186, #16487, #19036, #5808, #12050, #5943, #7931, #7510, #25465, #14611, #10329, #14060, #20776, #20915, #10058, #23328 ),
 .UNSPECIFIED., .F., .F.,
 ( 4, 2, 2, 2, 2, 2, 2, 2, 2, 2, 1, 2, 2, 2, 2, 4 ),
 ( 9.214435701904187837E-16, 0.001647793485001483246, 0.003295586970002045354, 0.004943380455002607463, 0.005767277197502887649, 0.006591173940003168703, 0.008238967425003728209, 0.009886760910004286848, 0.01318234788000540413, 0.01483014136500596276, 0.01647793485000652314, 0.01812572833500708178, 0.01977352182000764041, 0.02306910879000876116, 0.02471690227500931286, 0.02636469576000986109 ),
 .UNSPECIFIED. ) ;
#20522=ORIENTED_EDGE ( 'NONE', *, *, #27226, .F. ) ;
#20525=CARTESIAN_POINT ( 'NONE',  ( 204.5988444088204403, 36.83281250216787583, -9.598844408820458085 ) ) ;
#20526=CARTESIAN_POINT ( 'NONE',  ( 95.54126587499996504, 83.43750000136560629, -1.387778780781445676E-14 ) ) ;
#20528=CARTESIAN_POINT ( 'NONE',  ( 51.42518405393695957, 38.71796875216787726, 0.000000000000000000 ) ) ;
#20530=CARTESIAN_POINT ( 'NONE',  ( 204.2950502721270425, 40.25585937608393294, 9.295050272127046043 ) ) ;
#20531=CARTESIAN_POINT ( 'NONE',  ( 13.57481594606304753, 39.95820312716787726, -5.622872871577873077 ) ) ;
#20533=CARTESIAN_POINT ( 'NONE',  ( 182.1404900439225116, 36.00000000000000711, -3.245221471866913010 ) ) ;
#20537=CARTESIAN_POINT ( 'NONE',  ( 198.8783854107797424, 31.34156310770110565, -13.57481594606304931 ) ) ;
#20539=EDGE_CURVE ( 'NONE', #17753, #15719, #15268, .T. ) ;
#20542=CARTESIAN_POINT ( 'NONE',  ( -8.049105076161786076E-16, 31.82226562608393650, -13.14518615778179544 ) ) ;
#20543=CARTESIAN_POINT ( 'NONE',  ( 143.1451861577818079, 32.16953125108393152, 5.444914386472293977 ) ) ;
#20547=DIRECTION ( 'NONE',  ( 0.000000000000000000, -0.000000000000000000, 1.000000000000000000 ) ) ;
#20549=CARTESIAN_POINT ( 'NONE',  ( 51.85481384221819923, 40.50390625108394005, -5.444914386472297529 ) ) ;
#20556=CARTESIAN_POINT ( 'NONE',  ( -13.14518615778179544, 33.60820312608393579, 0.000000000000000000 ) ) ;
#20561=CARTESIAN_POINT ( 'NONE',  ( 200.4449143864723055, 34.74921875108394431, -13.14518615778179900 ) ) ;
#20564=CARTESIAN_POINT ( 'NONE',  ( 199.5715916325254966, 51.44262710531793203, -14.99999999999869083 ) ) ;
#20570=CARTESIAN_POINT ( 'NONE',  ( 139.2950502721270425, 37.08085937608393579, -9.295050272127046043 ) ) ;
#20571=CARTESIAN_POINT ( 'NONE',  ( -5.444914386472299306, 38.51953125108393294, 13.14518615778179722 ) ) ;
#20572=CARTESIAN_POINT ( 'NONE',  ( -13.14518615778179900, 40.70234375108393721, -5.444914386472297529 ) ) ;
#20574=LINE ( 'NONE', #22991, #26453 ) ;
#20579=CARTESIAN_POINT ( 'NONE',  ( 59.55508561352770158, 36.43593750108394147, -13.14518615778179722 ) ) ;
#20580=CARTESIAN_POINT ( 'NONE',  ( 195.0000000000000000, 37.72578125216787726, -13.57481594606304576 ) ) ;
#20581=CARTESIAN_POINT ( 'NONE',  ( 65.00000000000000000, 38.42031249999999432, -13.57481594606304576 ) ) ;
#20582=CARTESIAN_POINT ( 'NONE',  ( 189.5550856135277229, 37.22968750108394431, -13.14518615778179722 ) ) ;
#20587=CARTESIAN_POINT ( 'NONE',  ( 189.5550856135277229, 37.42812500108394147, -13.14518615778179722 ) ) ;
#20595=CARTESIAN_POINT ( 'NONE',  ( 181.8548138422181921, 33.65781250108393152, 5.444914386472304635 ) ) ;
#20596=ORIENTED_EDGE ( 'NONE', *, *, #21552, .T. ) ;
#20597=DIRECTION ( 'NONE',  ( -0.000000000000000000, 1.000000000000000000, -0.000000000000000000 ) ) ;
#20598=CARTESIAN_POINT ( 'NONE',  ( 9.180175813647991845, 50.00000000000000000, -9.999999999999996447 ) ) ;
#20599=PLANE ( 'NONE',  #17168 ) ;
#20600=CARTESIAN_POINT ( 'NONE',  ( 116.4251840539369596, 37.18007812716787441, 5.622872871577880183 ) ) ;
#20604=CARTESIAN_POINT ( 'NONE',  ( 204.2950502721270425, 40.45429687608393721, -9.295050272127046043 ) ) ;
#20612=CARTESIAN_POINT ( 'NONE',  ( -7.778504368121734736, 35.99999999999997868, 10.60546543669443231 ) ) ;
#20613=CARTESIAN_POINT ( 'NONE',  ( 74.59884440882045453, 37.42812500216787441, 9.598844408820456309 ) ) ;
#20616=CARTESIAN_POINT ( 'NONE',  ( -9.598844408820458085, 38.51953124999999289, -9.598844408820458085 ) ) ;
#20618=CARTESIAN_POINT ( 'NONE',  ( -1.138768117105833477, 50.00000000043849013, 13.56816686242529357 ) ) ;
#20619=CARTESIAN_POINT ( 'NONE',  ( 135.6228728715778971, 35.69179687499999432, 13.57481594606304576 ) ) ;
#20621=ORIENTED_EDGE ( 'NONE', *, *, #22413, .T. ) ;
#20622=FACE_BOUND ( 'NONE', #5124, .T. ) ;
#20628=CARTESIAN_POINT ( 'NONE',  ( 130.0000000000000000, 33.21132812608393436, -13.14518615778179544 ) ) ;
#20629=CARTESIAN_POINT ( 'NONE',  ( 51.85481384221819923, 38.91640625108393436, -5.444914386472297529 ) ) ;
#20631=CARTESIAN_POINT ( 'NONE',  ( 9.598844408820459861, 37.42812500216787441, 9.598844408820456309 ) ) ;
#20632=CARTESIAN_POINT ( 'NONE',  ( -5.444914386472297529, 38.02343750108394005, -13.14518615778179900 ) ) ;
#20634=CYLINDRICAL_SURFACE ( 'NONE', #10754, 4.999999999999999112 ) ;
#20637=CARTESIAN_POINT ( 'NONE',  ( 99.99999999999995737, 81.37500000273119838, 4.999999999999990230 ) ) ;
#20641=CARTESIAN_POINT ( 'NONE',  ( 185.4011555911795313, 39.31328124999999574, -9.598844408820458085 ) ) ;
#20644=CARTESIAN_POINT ( 'NONE',  ( 95.54126587499996504, 79.43750000136559208, -1.387778780781445676E-14 ) ) ;
#20649=CARTESIAN_POINT ( 'NONE',  ( 204.5988444088204403, 32.76484374999999716, -9.598844408820458085 ) ) ;
#20651=CARTESIAN_POINT ( 'NONE',  ( 2.493653234604083739E-15, 36.43593749999999432, 13.57481594606304576 ) ) ;
#20653=CARTESIAN_POINT ( 'NONE',  ( 65.00000000000000000, 32.81445312608393294, 13.14518615778179544 ) ) ;
#20658=CARTESIAN_POINT ( 'NONE',  ( -5.622872871577873077, 34.00507812499999716, 13.57481594606304753 ) ) ;
#20660=CARTESIAN_POINT ( 'NONE',  ( 143.1451861577818079, 34.00507812608393721, -1.609821015232357215E-15 ) ) ;
#20665=CARTESIAN_POINT ( 'NONE',  ( 103.1528011352953342, 81.81250000136559208, 3.152801135295355106 ) ) ;
#20667=CARTESIAN_POINT ( 'NONE',  ( 120.4011555911795455, 38.71796874999999716, 9.598844408820459861 ) ) ;
#20671=CARTESIAN_POINT ( 'NONE',  ( 208.1451861577818079, 40.35507812608393863, -1.609821015232357215E-15 ) ) ;
#20672=CARTESIAN_POINT ( 'NONE',  ( -8.312177448680279460E-16, 40.10703125216787157, -13.57481594606304576 ) ) ;
#20676=VERTEX_POINT ( 'NONE', #24571 ) ;
#20678=CARTESIAN_POINT ( 'NONE',  ( 208.1451861577817795, 39.31328125108392868, 5.444914386472293977 ) ) ;
#20682=CARTESIAN_POINT ( 'NONE',  ( 9.295050272127046043, 32.51679687608393721, -9.295050272127046043 ) ) ;
#20683=CARTESIAN_POINT ( 'NONE',  ( 143.5748159460630688, 37.42812499999999432, -1.662435489736055892E-15 ) ) ;
#20688=CARTESIAN_POINT ( 'NONE',  ( 117.2616098421445230, 35.99999999999998579, 3.273369733618576305 ) ) ;
#20690=CARTESIAN_POINT ( 'NONE',  ( 0.000000000000000000, -7.395377635281828788, 13.57481594606304398 ) ) ;
#20696=CARTESIAN_POINT ( 'NONE',  ( 5.444914386472302859, 33.85625000108393579, 13.14518615778179189 ) ) ;
#20697=ORIENTED_EDGE ( 'NONE', *, *, #21846, .F. ) ;
#20698=LINE ( 'NONE', #26976, #17274 ) ;
#20700=ADVANCED_FACE ( 'NONE', ( #8021 ), #23284, .T. ) ;
#20702=EDGE_CURVE ( 'NONE', #19327, #23304, #5618, .T. ) ;
#20703=CARTESIAN_POINT ( 'NONE',  ( 204.2950502721270425, 32.91367187608393152, 9.295050272127046043 ) ) ;
#20704=ORIENTED_EDGE ( 'NONE', *, *, #769, .T. ) ;
#20705=CARTESIAN_POINT ( 'NONE',  ( 190.4951129136680947, 51.44650206076642007, -14.99999999999734968 ) ) ;
#20707=ORIENTED_EDGE ( 'NONE', *, *, #1899, .T. ) ;
#20710=CARTESIAN_POINT ( 'NONE',  ( 185.4011555911795313, 39.41250000216787441, -9.598844408820458085 ) ) ;
#20712=CARTESIAN_POINT ( 'NONE',  ( 116.8548138422182063, 38.91640625108393436, -5.444914386472297529 ) ) ;
#20713=CARTESIAN_POINT ( 'NONE',  ( 2.414731522848535132E-15, 36.98164062608393721, 13.14518615778179544 ) ) ;
#20714=CARTESIAN_POINT ( 'NONE',  ( 9.295050272127047819, 40.25585937608393294, 9.295050272127046043 ) ) ;
#20717=CARTESIAN_POINT ( 'NONE',  ( 70.62287287157778337, 38.07304687499999574, 13.57481594606313813 ) ) ;
#20721=CARTESIAN_POINT ( 'NONE',  ( 99.99999999999995737, 84.43750000136560629, -4.458734125000016313 ) ) ;
#20724=ORIENTED_EDGE ( 'NONE', *, *, #1041, .F. ) ;
#20731=CARTESIAN_POINT ( 'NONE',  ( 130.0000000000000000, 39.31328125216787583, -13.57481594606304576 ) ) ;
#20733=ORIENTED_EDGE ( 'NONE', *, *, #4785, .F. ) ;
#20734=CARTESIAN_POINT ( 'NONE',  ( 185.4011555911795313, 37.03125000216787299, -9.598844408820458085 ) ) ;
#20735=CARTESIAN_POINT ( 'NONE',  ( 2.493653234604083739E-15, 36.53515625216787299, 13.57481594606304576 ) ) ;
#20736=CARTESIAN_POINT ( 'NONE',  ( 185.7049497278729575, 34.30273437608393294, -9.295050272127046043 ) ) ;
#20739=CARTESIAN_POINT ( 'NONE',  ( 1.602533130612657564, 53.60343507248209249, -15.00000000000000000 ) ) ;
#20740=AXIS2_PLACEMENT_3D ( 'NONE', #16626, #3670, #12332 ) ;
#20741=CARTESIAN_POINT ( 'NONE',  ( 139.5988444088204687, 36.63437500216787157, 9.598844408820456309 ) ) ;
#20745=CARTESIAN_POINT ( 'NONE',  ( 200.4449143864723055, 37.03125000108393294, 13.14518615778179189 ) ) ;
#20746=ORIENTED_EDGE ( 'NONE', *, *, #15588, .T. ) ;
#20747=VECTOR ( 'NONE', #17149, 1000.000000000000227 ) ;
#20750=CARTESIAN_POINT ( 'NONE',  ( -11.69037824551319460, 35.99999999999998579, -6.307928093363390332 ) ) ;
#20752=CARTESIAN_POINT ( 'NONE',  ( 51.42518405393695957, 40.99999999999999289, 0.000000000000000000 ) ) ;
#20754=CARTESIAN_POINT ( 'NONE',  ( -13.57481594606304398, 39.56132812716787583, 5.622872871577880183 ) ) ;
#20755=CARTESIAN_POINT ( 'NONE',  ( 13.04200858114998418, 36.00000000000000711, -3.640726557253423756 ) ) ;
#20756=CARTESIAN_POINT ( 'NONE',  ( 8.769389672083836018, 50.37710889402394088, 14.99999999999737277 ) ) ;
#20757=CARTESIAN_POINT ( 'NONE',  ( 124.3771271284221314, 35.29492187500000000, -13.57481594606304753 ) ) ;
#20764=CARTESIAN_POINT ( 'NONE',  ( 130.0000000000000000, 38.17226562608394147, -13.14518615778179544 ) ) ;
#20765=CARTESIAN_POINT ( 'NONE',  ( 74.29505027212704249, 40.25585937608393294, -9.295050272127046043 ) ) ;
#20767=FACE_BOUND ( 'NONE', #13550, .T. ) ;
#20768=CARTESIAN_POINT ( 'NONE',  ( 5.444914386472302859, 38.42031250108393436, 13.14518615778179189 ) ) ;
#20772=ADVANCED_FACE ( 'NONE', ( #21137 ), #1623, .T. ) ;
#20774=CARTESIAN_POINT ( 'NONE',  ( 204.2950502721270425, 32.11992187608393579, 9.295050272127046043 ) ) ;
#20776=CARTESIAN_POINT ( 'NONE',  ( 142.8921516136354342, 35.99999999999997158, -4.169510824908009283 ) ) ;
#20778=DIRECTION ( 'NONE',  ( 0.000000000000000000, 0.000000000000000000, 1.000000000000000000 ) ) ;
#20779=CARTESIAN_POINT ( 'NONE',  ( 118.8544531269044029, 36.00000000000001421, -7.260818043106923803 ) ) ;
#20780=CARTESIAN_POINT ( 'NONE',  ( 124.3771271284222308, 40.15664062716787441, -13.57481594606315412 ) ) ;
#20783=ORIENTED_EDGE ( 'NONE', *, *, #24830, .F. ) ;
#20787=CARTESIAN_POINT ( 'NONE',  ( 208.5748159460630688, 32.66562499999999858, -1.662435489736055892E-15 ) ) ;
#20790=CARTESIAN_POINT ( 'NONE',  ( 99.99999999999995737, 83.68750000136560629, 4.458734124999988779 ) ) ;
#20791=CARTESIAN_POINT ( 'NONE',  ( 65.00000000000000000, 32.41757812608393863, -13.14518615778179544 ) ) ;
#20794=ORIENTED_EDGE ( 'NONE', *, *, #16163, .F. ) ;
#20796=CARTESIAN_POINT ( 'NONE',  ( -5.622872871577873077, 34.50117187499999005, -13.57481594606304753 ) ) ;
#20798=CARTESIAN_POINT ( 'NONE',  ( 139.2950502721270425, 33.90585937608393863, 9.295050272127046043 ) ) ;
#20800=CARTESIAN_POINT ( 'NONE',  ( -6.079080020518830452, 54.65154858643462887, -14.99999999999999822 ) ) ;
#20802=CARTESIAN_POINT ( 'NONE',  ( 96.84719886470459471, 83.56250000136560629, 3.152801135295355994 ) ) ;
#20804=CARTESIAN_POINT ( 'NONE',  ( 51.90409344636400846, 36.00000000000000000, 1.137167824541468031 ) ) ;
#20806=CARTESIAN_POINT ( 'NONE',  ( 13.57481594606304753, 38.37070312716786447, -5.622872871577873077 ) ) ;
#20811=CARTESIAN_POINT ( 'NONE',  ( 189.5550856135277229, 40.40468750108393436, -13.14518615778179900 ) ) ;
#20816=CARTESIAN_POINT ( 'NONE',  ( 200.6228728715779255, 38.17226562716787441, 13.57481594606301023 ) ) ;
#20817=CARTESIAN_POINT ( 'NONE',  ( 13.14518615778179544, 32.41757812608393863, -1.609821015232357215E-15 ) ) ;
#20818=EDGE_CURVE ( 'NONE', #5192, #5473, #19947, .T. ) ;
#20820=CARTESIAN_POINT ( 'NONE',  ( 51.42518405393695957, 32.26874999999999716, 0.000000000000000000 ) ) ;
#20822=CARTESIAN_POINT ( 'NONE',  ( 181.8548138422181921, 32.76484375108393010, -5.444914386472297529 ) ) ;
#20826=SPHERICAL_SURFACE ( 'NONE', #13495, 5.000000000000000000 ) ;
#20832=CARTESIAN_POINT ( 'NONE',  ( 2.414731522848535132E-15, 32.21914062608393436, 13.14518615778179544 ) ) ;
#20833=ADVANCED_FACE ( 'NONE', ( #9111 ), #19279, .T. ) ;
#20834=ORIENTED_EDGE ( 'NONE', *, *, #26766, .T. ) ;
#20835=CARTESIAN_POINT ( 'NONE',  ( 103.1528011352953342, 82.31250000136559208, -3.152801135295383084 ) ) ;
#20836=CIRCLE ( 'NONE', #27667, 13.57481594606304398 ) ;
#20837=AXIS2_PLACEMENT_3D ( 'NONE', #7293, #20423, #907 ) ;
#20838=CARTESIAN_POINT ( 'NONE',  ( -8.312177448680279460E-16, 37.62656249999999858, -13.57481594606304576 ) ) ;
#20839=CARTESIAN_POINT ( 'NONE',  ( 181.8548138422181921, 34.15390625108393863, -5.444914386472297529 ) ) ;
#20841=CARTESIAN_POINT ( 'NONE',  ( 194.0169348148962740, 49.99999999949044849, -13.54930971656736638 ) ) ;
#20847=CARTESIAN_POINT ( 'NONE',  ( 185.4011555911795313, 38.61875000216787157, -9.598844408820458085 ) ) ;
#20849=CARTESIAN_POINT ( 'NONE',  ( 13.14518615778179722, 38.02343750108395426, -5.444914386472297529 ) ) ;
#20850=CARTESIAN_POINT ( 'NONE',  ( -5.444914386472297529, 40.60312500108393863, -13.14518615778179900 ) ) ;
#20852=CARTESIAN_POINT ( 'NONE',  ( 195.0000000000000000, -7.395377635281828788, -2.255140518769849538E-14 ) ) ;
#20857=CARTESIAN_POINT ( 'NONE',  ( 104.4587341249999781, 84.12500000136560629, 1.846868145590721655 ) ) ;
#20859=DIRECTION ( 'NONE',  ( 0.000000000000000000, 1.000000000000000000, 0.000000000000000000 ) ) ;
#20860=CARTESIAN_POINT ( 'NONE',  ( 65.32472431119603584, 53.49346745874647269, 14.99999999999997691 ) ) ;
#20864=DIRECTION ( 'NONE',  ( -0.000000000000000000, 1.000000000000000000, -0.000000000000000000 ) ) ;
#20865=CARTESIAN_POINT ( 'NONE',  ( 185.7049497278729575, 36.08867187608393579, 9.295050272127047819 ) ) ;
#20869=CARTESIAN_POINT ( 'NONE',  ( 74.29505027212704249, 39.46210937608393721, 9.295050272127046043 ) ) ;
#20870=EDGE_LOOP ( 'NONE', ( #25128, #17478, #17136, #28046 ) ) ;
#20879=CARTESIAN_POINT ( 'NONE',  ( 130.0000000000000000, 38.12265625216787157, 13.57481594606304576 ) ) ;
#20883=CARTESIAN_POINT ( 'NONE',  ( 204.2950502721270425, 37.08085937608393579, 9.295050272127046043 ) ) ;
#20888=DIRECTION ( 'NONE',  ( -0.000000000000000000, -1.000000000000000000, -0.000000000000000000 ) ) ;
#20891=FACE_OUTER_BOUND ( 'NONE', #12769, .T. ) ;
#20895=AXIS2_PLACEMENT_3D ( 'NONE', #654, #9327, #13591 ) ;
#20897=DIRECTION ( 'NONE',  ( 0.000000000000000000, 0.000000000000000000, -1.000000000000000000 ) ) ;
#20898=CARTESIAN_POINT ( 'NONE',  ( 135.6228728715778686, 35.19570312499999432, -13.57481594606304753 ) ) ;
#20906=CARTESIAN_POINT ( 'NONE',  ( 124.5550856135277087, 39.01562500108394005, -13.14518615778179900 ) ) ;
#20907=CARTESIAN_POINT ( 'NONE',  ( 78.14518615778179367, 36.93203125108394147, 5.444914386472293977 ) ) ;
#20909=CARTESIAN_POINT ( 'NONE',  ( -13.14518615778179900, 38.12265625108393152, -5.444914386472297529 ) ) ;
#20911=CARTESIAN_POINT ( 'NONE',  ( 51.42518405393695957, 37.82499999999999574, 0.000000000000000000 ) ) ;
#20914=CARTESIAN_POINT ( 'NONE',  ( 181.8548138422181921, 31.77265625108393365, -5.444914386472297529 ) ) ;
#20915=CARTESIAN_POINT ( 'NONE',  ( 142.5314254911195349, 35.99999999999996447, -5.200562670744178995 ) ) ;
#20917=( GEOMETRIC_REPRESENTATION_CONTEXT ( 3 ) GLOBAL_UNCERTAINTY_ASSIGNED_CONTEXT ( ( #17245 ) ) GLOBAL_UNIT_ASSIGNED_CONTEXT ( ( #16604, #1237, #18748 ) ) REPRESENTATION_CONTEXT ( 'NONE', 'WORKASPACE' ) );
#20919=CARTESIAN_POINT ( 'NONE',  ( 116.8258427830772348, 35.99999999999998579, 0.03826467346029212291 ) ) ;
#20920=CARTESIAN_POINT ( 'NONE',  ( 181.4251840539369596, 39.51171875216787299, 0.000000000000000000 ) ) ;
#20928=CARTESIAN_POINT ( 'NONE',  ( 96.84719886470459471, 81.31250000136559208, -3.152801135295383084 ) ) ;
#20929=CARTESIAN_POINT ( 'NONE',  ( 65.00000000000000000, 37.77539062608393294, 13.14518615778179544 ) ) ;
#20933=CARTESIAN_POINT ( 'NONE',  ( 51.42518405393695957, 38.76757812716787299, 5.622872871577880183 ) ) ;
#20935=CARTESIAN_POINT ( 'NONE',  ( 116.8548138422182205, 33.60820312608393579, 0.000000000000000000 ) ) ;
#20937=CARTESIAN_POINT ( 'NONE',  ( 139.5988444088204687, 37.42812500216787441, 9.598844408820456309 ) ) ;
#20943=CARTESIAN_POINT ( 'NONE',  ( 78.57481594606304043, 39.95820312716787726, -5.622872871577873077 ) ) ;
#20945=CARTESIAN_POINT ( 'NONE',  ( 5.622872871577871301, 38.46992187716787015, -13.57481594606304753 ) ) ;
#20947=VECTOR ( 'NONE', #6258, 1000.000000000000000 ) ;
#20951=CARTESIAN_POINT ( 'NONE',  ( 200.4449143864723055, 40.00781250108393294, 13.14518615778179189 ) ) ;
#20954=CARTESIAN_POINT ( 'NONE',  ( 116.8548138422182205, 37.42812500108393436, 5.444914386472304635 ) ) ;
#20955=CARTESIAN_POINT ( 'NONE',  ( 94.99999999999995737, 80.12500000273119838, -1.387778780781445676E-14 ) ) ;
#20956=DIRECTION ( 'NONE',  ( 1.000000000000000000, -0.000000000000000000, -7.228014483236696740E-18 ) ) ;
#20959=CARTESIAN_POINT ( 'NONE',  ( 200.6228728715778686, 39.16445312499999432, -13.57481594606304753 ) ) ;
#20964=AXIS2_PLACEMENT_3D ( 'NONE', #23482, #19617, #5959 ) ;
#20970=CARTESIAN_POINT ( 'NONE',  ( -5.622872871577873077, 40.35507812499998437, 13.57481594606304753 ) ) ;
#20972=CARTESIAN_POINT ( 'NONE',  ( 101.8468681455906903, 83.37500000136563472, -4.458734125000016313 ) ) ;
#20977=EDGE_CURVE ( 'NONE', #15512, #21487, #8005, .T. ) ;
#20979=CARTESIAN_POINT ( 'NONE',  ( 201.1610621748488370, 51.27996893917539012, -15.00000000000137845 ) ) ;
#20987=CARTESIAN_POINT ( 'NONE',  ( 135.4449143864723339, 40.20625000108394431, 13.14518615778179189 ) ) ;
#20988=CARTESIAN_POINT ( 'NONE',  ( 6.944426393311538881, 31.55306875057403104, -11.16113171639042356 ) ) ;
#20990=CARTESIAN_POINT ( 'NONE',  ( 78.57481594606304043, 37.37851562499999858, 5.622872871577869525 ) ) ;
#20996=CARTESIAN_POINT ( 'NONE',  ( 104.4587341249999781, 83.25000000136559208, -1.846868145590750521 ) ) ;
#20999=AXIS2_PLACEMENT_3D ( 'NONE', #20502, #9794, #16061 ) ;
#21001=ORIENTED_EDGE ( 'NONE', *, *, #1090, .F. ) ;
#21002=DIRECTION ( 'NONE',  ( 1.000000000000000000, 1.734723475976808080E-15, -7.228014483236698281E-18 ) ) ;
#21004=EDGE_CURVE ( 'NONE', #19618, #21949, #18559, .T. ) ;
#21006=FACE_OUTER_BOUND ( 'NONE', #20177, .T. ) ;
#21007=CARTESIAN_POINT ( 'NONE',  ( -20.00000000000000000, 50.00000000000000000, 10.00000000000000178 ) ) ;
#21010=CARTESIAN_POINT ( 'NONE',  ( 51.85481384221821344, 38.42031250108393436, 5.444914386472304635 ) ) ;
#21011=ADVANCED_FACE ( 'NONE', ( #12077 ), #27365, .T. ) ;
#21012=CARTESIAN_POINT ( 'NONE',  ( 0.000000000000000000, 52.00000000000000711, 0.000000000000000000 ) ) ;
#21013=CARTESIAN_POINT ( 'NONE',  ( 195.0000000000000000, 32.21914062608393436, 13.14518615778179544 ) ) ;
#21017=CARTESIAN_POINT ( 'NONE',  ( -3.636496246811128596, 51.46815297079189122, -15.00000000000000178 ) ) ;
#21020=CARTESIAN_POINT ( 'NONE',  ( 139.5988444088204687, 35.84062500216786873, 9.598844408820456309 ) ) ;
#21021=CYLINDRICAL_SURFACE ( 'NONE', #27896, 13.57481594606304398 ) ;
#21024=CARTESIAN_POINT ( 'NONE',  ( 195.0000000000000000, 36.58476562608393579, -13.14518615778179544 ) ) ;
#21028=CARTESIAN_POINT ( 'NONE',  ( 104.4587341249999781, 83.00000000136562051, -1.846868145590750521 ) ) ;
#21030=FACE_OUTER_BOUND ( 'NONE', #11588, .T. ) ;
#21033=CARTESIAN_POINT ( 'NONE',  ( 195.0000000000000000, -7.395377635281828788, -2.255140518769849538E-14 ) ) ;
#21041=CARTESIAN_POINT ( 'NONE',  ( 143.1451861577818079, 38.76757812608393294, -1.609821015232357215E-15 ) ) ;
#21042=CARTESIAN_POINT ( 'NONE',  ( 78.14518615778179367, 35.44375000108393436, -5.444914386472297529 ) ) ;
#21044=DIRECTION ( 'NONE',  ( 0.000000000000000000, -1.000000000000000000, 0.000000000000000000 ) ) ;
#21045=CARTESIAN_POINT ( 'NONE',  ( -9.295050272127044266, 35.09648437608392868, 9.295050272127047819 ) ) ;
#21046=( BOUNDED_CURVE ( )  B_SPLINE_CURVE ( 2, ( #9082, #8795, #6515, #15631, #26335, #19491, #15053, #25909, #24195 ),
 .UNSPECIFIED., .F., .T. ) 
 B_SPLINE_CURVE_WITH_KNOTS ( ( 3, 2, 2, 2, 3 ),
 ( 0.2500000000000002220, 0.2750000000000002442, 0.3000000000000002665, 0.3250000000000002887, 0.3500000000000003109 ),
 .UNSPECIFIED. ) 
 CURVE ( )  GEOMETRIC_REPRESENTATION_ITEM ( )  RATIONAL_B_SPLINE_CURVE ( ( 0.9999999999999993339, 0.9238795325112874046, 1.000000000000000000, 0.9238795325112867385, 1.000000000000000000, 0.9238795325112867385, 1.000000000000000000, 0.9238795325112857393, 1.000000000000001110 ) ) 
 REPRESENTATION_ITEM ( '' )  );
#21047=CARTESIAN_POINT ( 'NONE',  ( 196.4643377203195200, 35.99999999999997868, -13.46163418879037188 ) ) ;
#21049=CARTESIAN_POINT ( 'NONE',  ( 195.0000000000000000, 39.21406249999999716, -13.57481594606304576 ) ) ;
#21051=CARTESIAN_POINT ( 'NONE',  ( 195.0000000000000000, 40.80156249999999574, -13.57481594606304576 ) ) ;
#21052=CARTESIAN_POINT ( 'NONE',  ( -8.049105076161786076E-16, 37.18007812608393436, -13.14518615778179544 ) ) ;
#21053=CARTESIAN_POINT ( 'NONE',  ( 131.1371678245417627, 36.00000000000000000, 13.09590655363595602 ) ) ;
#21056=DIRECTION ( 'NONE',  ( -0.000000000000000000, -1.000000000000000000, -0.000000000000000000 ) ) ;
#21059=CARTESIAN_POINT ( 'NONE',  ( 116.4251840539369596, 40.95039062499999005, -5.622872871577872189 ) ) ;
#21065=CARTESIAN_POINT ( 'NONE',  ( 103.1528011352953342, 80.81250000136559208, 3.152801135295355106 ) ) ;
#21066=CARTESIAN_POINT ( 'NONE',  ( 51.85481384221820633, 37.57695312608393579, 0.000000000000000000 ) ) ;
#21072=CARTESIAN_POINT ( 'NONE',  ( 130.0000000000000000, 32.61601562608393579, -13.14518615778179544 ) ) ;
#21074=CARTESIAN_POINT ( 'NONE',  ( 0.8421075954646569661, 53.50112910130383881, -15.00000000000000178 ) ) ;
#21076=CARTESIAN_POINT ( 'NONE',  ( 103.1528011352953342, 79.81250000136559208, 3.152801135295355106 ) ) ;
#21077=CARTESIAN_POINT ( 'NONE',  ( 124.5550856135277087, 39.61093750108393152, -13.14518615778179900 ) ) ;
#21078=CARTESIAN_POINT ( 'NONE',  ( 78.57481594606305464, 35.93984375216787441, -1.662435489736055892E-15 ) ) ;
#21080=CARTESIAN_POINT ( 'NONE',  ( -5.622872871577873077, 34.60039062716786873, -13.57481594606304753 ) ) ;
#21086=CARTESIAN_POINT ( 'NONE',  ( 181.8548138422181921, 36.63437500108393152, 5.444914386472304635 ) ) ;
#21087=CARTESIAN_POINT ( 'NONE',  ( 13.57481594606304753, 36.78320312716788010, -5.622872871577873966 ) ) ;
#21088=CARTESIAN_POINT ( 'NONE',  ( 130.0000000000000000, 37.57695312608392868, 13.14518615778179544 ) ) ;
#21089=CARTESIAN_POINT ( 'NONE',  ( 5.444914386472302859, 32.26875000108393721, 13.14518615778179189 ) ) ;
#21092=CARTESIAN_POINT ( 'NONE',  ( 59.37712712842218821, 37.18007812499999432, 13.57481594606311504 ) ) ;
#21094=CARTESIAN_POINT ( 'NONE',  ( 195.0000000000000000, 38.42031249999999432, -13.57481594606304576 ) ) ;
#21095=PRODUCT_CONTEXT ( 'NONE', #18624, 'mechanical' ) ;
#21096=LINE ( 'NONE', #16675, #20947 ) ;
#21098=CARTESIAN_POINT ( 'NONE',  ( 74.29505027212704249, 40.05742187608392868, 9.295050272127046043 ) ) ;
#21104=CARTESIAN_POINT ( 'NONE',  ( 5.622872871577871301, 38.37070312499999147, -13.57481594606304753 ) ) ;
#21106=CARTESIAN_POINT ( 'NONE',  ( 99.99999999999995737, 84.43750000136560629, -4.458734125000016313 ) ) ;
#21107=AXIS2_PLACEMENT_3D ( 'NONE', #26919, #2687, #5105 ) ;
#21117=CARTESIAN_POINT ( 'NONE',  ( 185.4011555911795597, 39.61093750216787868, 9.598844408820459861 ) ) ;
#21120=CARTESIAN_POINT ( 'NONE',  ( 116.8548138422182205, 40.70234375108392300, -5.444914386472297529 ) ) ;
#21121=CARTESIAN_POINT ( 'NONE',  ( -13.14518615778179189, 33.45937500108392726, 5.444914386472304635 ) ) ;
#21124=CARTESIAN_POINT ( 'NONE',  ( 70.62287287157788285, 36.48554687499999716, 13.57481594606304576 ) ) ;
#21126=CARTESIAN_POINT ( 'NONE',  ( 202.0656349887611327, 36.00000000000000000, 11.21307450592185795 ) ) ;
#21131=CARTESIAN_POINT ( 'NONE',  ( 96.84719886470459471, 83.56250000136560629, -3.152801135295383084 ) ) ;
#21133=CARTESIAN_POINT ( 'NONE',  ( -9.295050272127046043, 39.06523437608392868, -9.295050272127046043 ) ) ;
#21134=LINE ( 'NONE', #3752, #23801 ) ;
#21136=CARTESIAN_POINT ( 'NONE',  ( 65.00000000000000000, 38.91640625216786731, 13.57481594606304576 ) ) ;
#21137=FACE_OUTER_BOUND ( 'NONE', #19297, .T. ) ;
#21140=CARTESIAN_POINT ( 'NONE',  ( 120.4011555911795455, 39.61093750216787868, 9.598844408820459861 ) ) ;
#21141=VERTEX_POINT ( 'NONE', #18521 ) ;
#21142=CARTESIAN_POINT ( 'NONE',  ( 70.44491438647229131, 38.61875000108392442, 13.14518615778179189 ) ) ;
#21144=CARTESIAN_POINT ( 'NONE',  ( 74.18017581364799184, 55.00000000000000000, -14.99999999999999822 ) ) ;
#21146=EDGE_LOOP ( 'NONE', ( #186, #9420, #14095, #518 ) ) ;
#21149=CARTESIAN_POINT ( 'NONE',  ( -0.7238719380229414746, 53.51529642094998707, -14.99999999999999645 ) ) ;
#21150=CARTESIAN_POINT ( 'NONE',  ( 194.1578924045353745, 53.50112910130381749, 14.99999999999995204 ) ) ;
#21151=CARTESIAN_POINT ( 'NONE',  ( 143.5748159460630404, 34.30273437716787299, 5.622872871577869525 ) ) ;
#21152=CARTESIAN_POINT ( 'NONE',  ( 103.5355339059327093, 81.50000000273119838, 3.535533905932726206 ) ) ;
#21153=EDGE_CURVE ( 'NONE', #5951, #10805, #7645, .T. ) ;
#21154=CARTESIAN_POINT ( 'NONE',  ( -15.00000000000000178, 80.00000000000000000, 1.734723475976807489E-15 ) ) ;
#21155=CARTESIAN_POINT ( 'NONE',  ( 181.8548138422181921, 38.32109375108394289, -5.444914386472297529 ) ) ;
#21158=ORIENTED_EDGE ( 'NONE', *, *, #648, .F. ) ;
#21160=DIRECTION ( 'NONE',  ( 0.000000000000000000, -1.000000000000000000, 0.000000000000000000 ) ) ;
#21162=ADVANCED_FACE ( 'NONE', ( #1422 ), #3970, .T. ) ;
#21168=CARTESIAN_POINT ( 'NONE',  ( 13.49550141231717859, 35.99999999999999289, -0.9550757908088484127 ) ) ;
#21170=CARTESIAN_POINT ( 'NONE',  ( 65.00000000000000000, -7.395377635281828788, -13.57481594606305109 ) ) ;
#21171=EDGE_CURVE ( 'NONE', #8092, #15512, #15289, .T. ) ;
#21172=ORIENTED_EDGE ( 'NONE', *, *, #23634, .F. ) ;
#21173=( BOUNDED_CURVE ( )  B_SPLINE_CURVE ( 2, ( #25143, #7620, #27574 ),
 .UNSPECIFIED., .F., .T. ) 
 B_SPLINE_CURVE_WITH_KNOTS ( ( 3, 3 ),
 ( 0.5208333333333332593, 0.5249747582430949189 ),
 .UNSPECIFIED. ) 
 CURVE ( )  GEOMETRIC_REPRESENTATION_ITEM ( )  RATIONAL_B_SPLINE_CURVE ( ( 1.000000000000000888, 0.9697362687807569159, 0.9635368518655843539 ) ) 
 REPRESENTATION_ITEM ( '' )  );
#21177=CARTESIAN_POINT ( 'NONE',  ( 116.8548138422182063, 39.11484375108394573, -5.444914386472297529 ) ) ;
#21178=CARTESIAN_POINT ( 'NONE',  ( 70.44491438647230552, 38.42031250108393436, 13.14518615778179189 ) ) ;
#21179=CARTESIAN_POINT ( 'NONE',  ( 204.2950502721270425, 39.66054687608393436, -9.295050272127046043 ) ) ;
#21180=CARTESIAN_POINT ( 'NONE',  ( 57.22149563187823418, 36.00000000000000000, 10.60546543669440034 ) ) ;
#21181=CARTESIAN_POINT ( 'NONE',  ( -13.14518615778179900, 34.15390625108393863, -5.444914386472297529 ) ) ;
#21182=CARTESIAN_POINT ( 'NONE',  ( 55.40115559117954547, 36.13828124999999147, -9.598844408820458085 ) ) ;
#21186=CARTESIAN_POINT ( 'NONE',  ( 9.295050272127046043, 37.08085937608393579, -9.295050272127046043 ) ) ;
#21187=LINE ( 'NONE', #7657, #12881 ) ;
#21189=CARTESIAN_POINT ( 'NONE',  ( 4.157286354961724939, 36.00000000000000000, -12.92256159328856135 ) ) ;
#21192=CARTESIAN_POINT ( 'NONE',  ( 189.3771271284220745, 39.36289062716787157, -13.57481594606297293 ) ) ;
#21195=AXIS2_PLACEMENT_3D ( 'NONE', #2870, #5301, #13965 ) ;
#21202=CARTESIAN_POINT ( 'NONE',  ( 181.4251840539369596, 36.28710937716787299, -5.622872871577872189 ) ) ;
#21203=CARTESIAN_POINT ( 'NONE',  ( 104.4587341249999781, 84.25000000136559208, -1.846868145590750299 ) ) ;
#21204=CARTESIAN_POINT ( 'NONE',  ( 78.14518615778179367, 39.61093750108393863, -5.444914386472297529 ) ) ;
#21206=CARTESIAN_POINT ( 'NONE',  ( -13.14518615778179722, 40.50390625108394005, -5.444914386472297529 ) ) ;
#21210=CARTESIAN_POINT ( 'NONE',  ( 120.4011555911795455, 39.31328124999999574, -9.598844408820458085 ) ) ;
#21211=ORIENTED_EDGE ( 'NONE', *, *, #27672, .T. ) ;
#21212=CARTESIAN_POINT ( 'NONE',  ( -1.887528725876408409, 53.66306546785492060, -15.00000000000000355 ) ) ;
#21213=DIRECTION ( 'NONE',  ( -0.000000000000000000, 1.000000000000000000, -0.000000000000000000 ) ) ;
#21217=CARTESIAN_POINT ( 'NONE',  ( 78.57481594606304043, 38.27148437716787299, 5.622872871577869525 ) ) ;
#21219=CARTESIAN_POINT ( 'NONE',  ( 5.622872871577871301, 35.29492187716788720, -13.57481594606304753 ) ) ;
#21223=VERTEX_POINT ( 'NONE', #14838 ) ;
#21224=CARTESIAN_POINT ( 'NONE',  ( 208.1451861577817795, 36.23750000108393010, -5.444914386472297529 ) ) ;
#21225=DIRECTION ( 'NONE',  ( -0.000000000000000000, 1.000000000000000000, -0.000000000000000000 ) ) ;
#21226=EDGE_CURVE ( 'NONE', #28031, #3171, #3476, .T. ) ;
#21227=CARTESIAN_POINT ( 'NONE',  ( 116.8548138422182205, 36.63437500108393863, 5.444914386472304635 ) ) ;
#21228=CYLINDRICAL_SURFACE ( 'NONE', #23280, 13.57481594606304398 ) ;
#21234=CARTESIAN_POINT ( 'NONE',  ( 195.0000000000000000, 38.81718749999999574, 13.57481594606304576 ) ) ;
#21238=CARTESIAN_POINT ( 'NONE',  ( 59.55508561352770158, 39.11484375108394573, 13.14518615778179722 ) ) ;
#21244=CARTESIAN_POINT ( 'NONE',  ( -13.57481594606304576, 38.66835937499999432, 5.622872871577880183 ) ) ;
#21245=CARTESIAN_POINT ( 'NONE',  ( 116.8548138422182063, 40.00781250108393294, 5.444914386472304635 ) ) ;
#21247=CARTESIAN_POINT ( 'NONE',  ( 95.54126587499995082, 82.62500000136560629, -1.846868145590750077 ) ) ;
#21251=CARTESIAN_POINT ( 'NONE',  ( 51.85481384221820633, 35.24531250108393721, 5.444914386472304635 ) ) ;
#21256=ORIENTED_EDGE ( 'NONE', *, *, #27057, .F. ) ;
#21257=LINE ( 'NONE', #25945, #6585 ) ;
#21259=CARTESIAN_POINT ( 'NONE',  ( 208.5748159460630688, 38.32109375216786873, -1.662435489736055892E-15 ) ) ;
#21262=CARTESIAN_POINT ( 'NONE',  ( 198.6364962467981456, 51.46815297079464813, 14.99999999999995381 ) ) ;
#21263=CARTESIAN_POINT ( 'NONE',  ( 124.5550856135277087, 40.60312500108393863, -13.14518615778179722 ) ) ;
#21264=CARTESIAN_POINT ( 'NONE',  ( 9.295050272127046043, 39.66054687608393436, -9.295050272127046043 ) ) ;
#21265=CARTESIAN_POINT ( 'NONE',  ( 74.59884440882045453, 39.11484374999999858, -9.598844408820458085 ) ) ;
#21266=DIRECTION ( 'NONE',  ( -0.000000000000000000, 1.000000000000000000, -0.000000000000000000 ) ) ;
#21272=CARTESIAN_POINT ( 'NONE',  ( 98.15313185440923860, 84.50000000136560629, -4.458734125000016313 ) ) ;
#21274=CARTESIAN_POINT ( 'NONE',  ( 5.444914386472302859, 40.20625000108394431, 13.14518615778179189 ) ) ;
#21275=CYLINDRICAL_SURFACE ( 'NONE', #20166, 13.57481594606304398 ) ;
#21279=DIRECTION ( 'NONE',  ( -1.000000000000000000, -0.000000000000000000, 2.385244779468110248E-16 ) ) ;
#21283=CARTESIAN_POINT ( 'NONE',  ( 99.99999999999995737, 80.75000000000000000, -5.000000000000018652 ) ) ;
#21284=ORIENTED_EDGE ( 'NONE', *, *, #18072, .F. ) ;
#21285=CARTESIAN_POINT ( 'NONE',  ( 59.55508561352770158, 38.22187500108393721, -13.14518615778179722 ) ) ;
#21287=CARTESIAN_POINT ( 'NONE',  ( 208.1451861577817795, 32.46718750108393436, -5.444914386472297529 ) ) ;
#21288=VERTEX_POINT ( 'NONE', #25420 ) ;
#21294=CARTESIAN_POINT ( 'NONE',  ( 139.5988444088204403, 35.24531250216787726, -9.598844408820458085 ) ) ;
#21296=CARTESIAN_POINT ( 'NONE',  ( 102.0710678118654329, 81.81250000273118417, -4.999999999999992006 ) ) ;
#21298=CARTESIAN_POINT ( 'NONE',  ( 200.4449143864723055, 37.32890625108393579, -13.14518615778179900 ) ) ;
#21300=EDGE_LOOP ( 'NONE', ( #7567, #7145, #3198, #4717, #7916 ) ) ;
#21303=CARTESIAN_POINT ( 'NONE',  ( 13.57481594606304753, 38.27148437500000711, -5.622872871577873966 ) ) ;
#21304=CARTESIAN_POINT ( 'NONE',  ( 98.15313185440923860, 84.25000000136559208, -4.458734125000016313 ) ) ;
#21305=CARTESIAN_POINT ( 'NONE',  ( 78.57481594606305464, 39.85898437716787157, 5.622872871577868636 ) ) ;
#21307=DIRECTION ( 'NONE',  ( 0.000000000000000000, 0.000000000000000000, -1.000000000000000000 ) ) ;
#21310=VECTOR ( 'NONE', #17909, 1000.000000000000000 ) ;
#21316=CARTESIAN_POINT ( 'NONE',  ( 143.1451861577818079, 39.51171875108392584, 5.444914386472293977 ) ) ;
#21317=EDGE_CURVE ( 'NONE', #3877, #16151, #7817, .T. ) ;
#21318=CARTESIAN_POINT ( 'NONE',  ( 51.85481384221820633, 38.22187500108393010, 5.444914386472304635 ) ) ;
#21319=CARTESIAN_POINT ( 'NONE',  ( 204.2950502721270425, 39.46210937608393721, 9.295050272127046043 ) ) ;
#21322=CARTESIAN_POINT ( 'NONE',  ( -15.00000000000000000, 55.00000000000000000, 9.999999999999998224 ) ) ;
#21323=CARTESIAN_POINT ( 'NONE',  ( -5.444914386472299306, 36.73359375108393010, 13.14518615778179722 ) ) ;
#21324=CARTESIAN_POINT ( 'NONE',  ( 188.5294363033335685, 36.00000000000000711, -11.78199955157030487 ) ) ;
#21326=CARTESIAN_POINT ( 'NONE',  ( 124.3771271284220745, 40.05742187499998863, -13.57481594606297293 ) ) ;
#21327=CARTESIAN_POINT ( 'NONE',  ( -9.295050272127046043, 39.66054687608393436, -9.295050272127046043 ) ) ;
#21328=CARTESIAN_POINT ( 'NONE',  ( 6.079080020518838445, 54.65154858643462177, 14.99999999999999645 ) ) ;
#21331=AXIS2_PLACEMENT_3D ( 'NONE', #16128, #27131, #16417 ) ;
#21341=CARTESIAN_POINT ( 'NONE',  ( 195.0000000000000000, -7.395377635281828788, -13.57481594606306707 ) ) ;
#21344=CARTESIAN_POINT ( 'NONE',  ( 104.4587341249999781, 79.87500000136559208, 1.846868145590721655 ) ) ;
#21345=CARTESIAN_POINT ( 'NONE',  ( 55.70494972787295751, 38.46992187608393721, 9.295050272127047819 ) ) ;
#21346=( BOUNDED_SURFACE ( )  B_SPLINE_SURFACE ( 3, 2, ( 
 ( #24027, #17323, #13020 ),
 ( #13305, #26019, #21473 ),
 ( #19887, #4505, #13162 ),
 ( #373, #2087, #23606 ),
 ( #2234, #2375, #15164 ),
 ( #9057, #17749, #19742 ),
 ( #4085, #10618, #226 ),
 ( #19324, #28026, #8492 ),
 ( #25884, #6353, #15026 ),
 ( #7473, #17890, #18319 ),
 ( #2925, #945, #7332 ),
 ( #20464, #24592, #5074 ),
 ( #9196, #11739, #1088 ),
 ( #5357, #13736, #2791 ),
 ( #9616, #11596, #26597 ),
 ( #27027, #9755, #22460 ),
 ( #16168, #2651, #24446 ),
 ( #15742, #22745, #11456 ),
 ( #11314, #18026, #18465 ),
 ( #7183, #24877, #20316 ) ),
 .UNSPECIFIED., .F., .F., .F. ) 
 B_SPLINE_SURFACE_WITH_KNOTS ( ( 4, 2, 2, 2, 2, 2, 2, 2, 2, 4 ),
 ( 3, 3 ),
 ( 0.009073803551359463371, 0.01139250602759181788, 0.01371120850382417239, 0.01602991098005652690, 0.01834861345628888141, 0.01950796469440505693, 0.02066731593252123592, 0.02298601840875359043, 0.02530472088498594146, 0.02762342336121829597 ),
 ( 0.000000000000000000, 1.000000000000000000 ),
 .UNSPECIFIED. ) 
 GEOMETRIC_REPRESENTATION_ITEM ( )  RATIONAL_B_SPLINE_SURFACE ( (
 ( 1.000000000000000000, 0.7071067811865473507, 1.000000000000000000),
 ( 1.000000000000000000, 0.7344871497828887597, 1.000000000000000000),
 ( 1.000000000000000000, 0.7612510203318868518, 1.000000000000000000),
 ( 1.000000000000000000, 0.8116663633844006798, 1.000000000000000000),
 ( 1.000000000000000000, 0.8353358059751632148, 1.000000000000000000),
 ( 1.000000000000000000, 0.8764699612586239752, 1.000000000000000000),
 ( 1.000000000000000000, 0.8939017358720021678, 1.000000000000000000),
 ( 1.000000000000000000, 0.9185314935646265999, 1.000000000000000000),
 ( 1.000000000000000000, 0.9256439951239476827, 1.000000000000000000),
 ( 1.000000000000000000, 0.9261623622476511386, 1.000000000000000000),
 ( 1.000000000000000000, 0.9246301385978846765, 1.000000000000000000),
 ( 1.000000000000000000, 0.9183304321348021437, 1.000000000000000000),
 ( 1.000000000000000000, 0.9135987334168410579, 1.000000000000000000),
 ( 1.000000000000000000, 0.8954110486039674743, 1.000000000000000000),
 ( 1.000000000000000000, 0.8779877431163538581, 1.000000000000000000),
 ( 1.000000000000000000, 0.8366182664709980177, 1.000000000000000000),
 ( 1.000000000000000000, 0.8126941604015293086, 1.000000000000000000),
 ( 1.000000000000000000, 0.7617527316305964247, 1.000000000000000000),
 ( 1.000000000000000000, 0.7347103785791970765, 1.000000000000000000),
 ( 1.000000000000000000, 0.7071067811865467956, 1.000000000000000000) ) ) 
 REPRESENTATION_ITEM ( '' )  SURFACE ( )  );
#21348=CARTESIAN_POINT ( 'NONE',  ( 13.14518615778179544, 40.15664062608393436, -1.609821015232357215E-15 ) ) ;
#21351=CARTESIAN_POINT ( 'NONE',  ( 51.42518405393695957, 38.71796875216787726, 0.000000000000000000 ) ) ;
#21353=CARTESIAN_POINT ( 'NONE',  ( 143.5748159460630688, 40.60312499999999858, -1.662435489736055892E-15 ) ) ;
#21354=ORIENTED_EDGE ( 'NONE', *, *, #26500, .F. ) ;
#21356=CARTESIAN_POINT ( 'NONE',  ( 99.99999999999995737, 85.00000000000000000, -1.387778780781445676E-14 ) ) ;
#21358=CARTESIAN_POINT ( 'NONE',  ( 124.5550856135277087, 39.90859375108393436, 13.14518615778179722 ) ) ;
#21360=CARTESIAN_POINT ( 'NONE',  ( 78.57481594606304043, 35.89023437716787868, 5.622872871577869525 ) ) ;
#21362=CARTESIAN_POINT ( 'NONE',  ( -13.57481594606304576, 37.13046875216787868, 0.000000000000000000 ) ) ;
#21364=AXIS2_PLACEMENT_3D ( 'NONE', #19548, #19403, #21554 ) ;
#21367=VERTEX_POINT ( 'NONE', #21283 ) ;
#21368=CARTESIAN_POINT ( 'NONE',  ( 195.0000000000000000, 37.97382812608393721, -13.14518615778179544 ) ) ;
#21371=CARTESIAN_POINT ( 'NONE',  ( 143.1451861577818363, 38.51953125108393294, 5.444914386472293977 ) ) ;
#21373=FACE_OUTER_BOUND ( 'NONE', #24170, .T. ) ;
#21377=CARTESIAN_POINT ( 'NONE',  ( 200.6228728715778686, 36.78320312499999289, -13.57481594606304753 ) ) ;
#21381=CARTESIAN_POINT ( 'NONE',  ( 78.14518615778179367, 40.15664062608393436, -1.609821015232357215E-15 ) ) ;
#21386=CIRCLE ( 'NONE', #450, 13.57481594606304398 ) ;
#21387=CARTESIAN_POINT ( 'NONE',  ( 130.0000000000000000, 39.21406249999999716, -13.57481594606304576 ) ) ;
#21388=CARTESIAN_POINT ( 'NONE',  ( 13.57481594606304931, 38.17226562499999432, 5.622872871577869525 ) ) ;
#21391=CARTESIAN_POINT ( 'NONE',  ( 104.4587341249999781, 84.12500000136560629, 1.846868145590721655 ) ) ;
#21393=ORIENTED_EDGE ( 'NONE', *, *, #18203, .F. ) ;
#21396=CARTESIAN_POINT ( 'NONE',  ( 74.29505027212704249, 34.89804687608393863, -9.295050272127046043 ) ) ;
#21399=ADVANCED_FACE ( 'NONE', ( #14430 ), #1085, .T. ) ;
#21401=EDGE_LOOP ( 'NONE', ( #25811, #27845, #25402, #17870 ) ) ;
#21404=CARTESIAN_POINT ( 'NONE',  ( 185.4011555911795313, 38.61875000216787157, -9.598844408820458085 ) ) ;
#21406=CARTESIAN_POINT ( 'NONE',  ( 214.9999999999999716, 75.00000000000000000, 9.999999999999946709 ) ) ;
#21407=CARTESIAN_POINT ( 'NONE',  ( 124.5550856135277087, 39.31328125108392868, 13.14518615778179722 ) ) ;
#21408=CARTESIAN_POINT ( 'NONE',  ( -5.444914386472299306, 39.31328125108394289, 13.14518615778179722 ) ) ;
#21409=AXIS2_PLACEMENT_3D ( 'NONE', #25202, #7527, #24782 ) ;
#21411=CARTESIAN_POINT ( 'NONE',  ( 74.59884440882045453, 36.53515624999999289, 9.598844408820456309 ) ) ;
#21418=CARTESIAN_POINT ( 'NONE',  ( 104.4587341249999781, 80.12500000136560629, 1.846868145590721655 ) ) ;
#21420=CARTESIAN_POINT ( 'NONE',  ( -9.295050272127046043, 40.65273437608393436, -9.295050272127046043 ) ) ;
#21422=ORIENTED_EDGE ( 'NONE', *, *, #19587, .T. ) ;
#21423=CARTESIAN_POINT ( 'NONE',  ( 195.0000000000000000, 50.00000000000000000, -2.255140518769849538E-14 ) ) ;
#21426=CARTESIAN_POINT ( 'NONE',  ( -13.57481594606304753, 40.15664062499999432, -5.622872871577872189 ) ) ;
#21428=CARTESIAN_POINT ( 'NONE',  ( 181.8548138422181921, 38.91640625108393436, -5.444914386472297529 ) ) ;
#21430=CARTESIAN_POINT ( 'NONE',  ( 51.85481384221821344, 39.21406250108392300, 5.444914386472304635 ) ) ;
#21432=CARTESIAN_POINT ( 'NONE',  ( 130.0000000000000000, 36.13828125216787157, -13.57481594606304576 ) ) ;
#21433=VERTEX_POINT ( 'NONE', #14574 ) ;
#21437=CARTESIAN_POINT ( 'NONE',  ( 130.0000000000000000, 34.55078125216787299, -13.57481594606304576 ) ) ;
#21438=CARTESIAN_POINT ( 'NONE',  ( 195.0000000000000000, 40.80156249999999574, -13.57481594606304576 ) ) ;
#21439=CARTESIAN_POINT ( 'NONE',  ( -15.00000000000000355, 75.00000000000000000, -9.999999999999998224 ) ) ;
#21441=CARTESIAN_POINT ( 'NONE',  ( 189.5550856135277229, 33.45937500108394147, -13.14518615778179900 ) ) ;
#21442=VERTEX_POINT ( 'NONE', #21432 ) ;
#21443=ADVANCED_FACE ( 'NONE', ( #7756 ), #10021, .T. ) ;
#21447=CARTESIAN_POINT ( 'NONE',  ( 78.14518615778179367, 39.36289062608393152, -1.609821015232357215E-15 ) ) ;
#21448=CARTESIAN_POINT ( 'NONE',  ( 95.54126587499996504, 79.50000000136560629, 1.846868145590724986 ) ) ;
#21452=CYLINDRICAL_SURFACE ( 'NONE', #28054, 13.57481594606304398 ) ;
#21453=CARTESIAN_POINT ( 'NONE',  ( 181.8548138422182205, 39.90859375108393436, -5.444914386472297529 ) ) ;
#21459=CARTESIAN_POINT ( 'NONE',  ( 120.7049497278729575, 35.89023437608393152, -9.295050272127046043 ) ) ;
#21460=CARTESIAN_POINT ( 'NONE',  ( 59.55508561352770158, 37.52734375108393294, 13.14518615778179722 ) ) ;
#21461=CARTESIAN_POINT ( 'NONE',  ( 195.0000000000000000, 32.02070312608393010, 13.14518615778179544 ) ) ;
#21462=EDGE_LOOP ( 'NONE', ( #3076, #26558, #22036, #14840 ) ) ;
#21463=CARTESIAN_POINT ( 'NONE',  ( 65.27033697766381692, 35.99999999999999289, 13.14949859323921366 ) ) ;
#21464=CARTESIAN_POINT ( 'NONE',  ( -13.14518615778179189, 35.84062500108394289, 5.444914386472304635 ) ) ;
#21465=CARTESIAN_POINT ( 'NONE',  ( 123.8801563722988703, 51.28708186914935396, -14.99999999999929834 ) ) ;
#21466=( BOUNDED_CURVE ( )  B_SPLINE_CURVE ( 2, ( #19286, #4318, #14987, #185, #8587, #8867, #17276, #4743, #6449 ),
 .UNSPECIFIED., .F., .T. ) 
 B_SPLINE_CURVE_WITH_KNOTS ( ( 3, 2, 2, 2, 3 ),
 ( 0.1041666666666664909, 0.1145833333333332732, 0.1250000000000000833, 0.1354166666666668517, 0.1458333333333336757 ),
 .UNSPECIFIED. ) 
 CURVE ( )  GEOMETRIC_REPRESENTATION_ITEM ( )  RATIONAL_B_SPLINE_CURVE ( ( 1.000000000000001332, 0.9238795325112854062, 1.000000000000000000, 0.9238795325112867385, 1.000000000000000000, 0.9238795325112867385, 1.000000000000000000, 0.9238795325112842960, 1.000000000000002442 ) ) 
 REPRESENTATION_ITEM ( '' )  );
#21467=CARTESIAN_POINT ( 'NONE',  ( 130.0000000000000000, 50.00000000000000000, -1.503427012513233026E-14 ) ) ;
#21470=CARTESIAN_POINT ( 'NONE',  ( 2.414731522848535132E-15, 39.95820312608393010, 13.14518615778179544 ) ) ;
#21471=CARTESIAN_POINT ( 'NONE',  ( -0.8421075954646584094, 53.50112910130383170, 14.99999999999999645 ) ) ;
#21473=CARTESIAN_POINT ( 'NONE',  ( 56.59768421877713251, 54.99999999485619639, 14.99999999999998401 ) ) ;
#21479=CARTESIAN_POINT ( 'NONE',  ( 95.54126587499995082, 83.62500000136560629, -1.846868145590750077 ) ) ;
#21480=CARTESIAN_POINT ( 'NONE',  ( 51.85481384221820633, 37.62656250108393863, 5.444914386472304635 ) ) ;
#21482=CARTESIAN_POINT ( 'NONE',  ( 5.444914386472302859, 40.00781250108393294, 13.14518615778179189 ) ) ;
#21486=CARTESIAN_POINT ( 'NONE',  ( 120.4011555911795455, 39.51171874999999289, 9.598844408820459861 ) ) ;
#21487=VERTEX_POINT ( 'NONE', #18730 ) ;
#21490=CARTESIAN_POINT ( 'NONE',  ( 104.4587341249999781, 80.00000000136559208, -1.846868145590750299 ) ) ;
#21491=CARTESIAN_POINT ( 'NONE',  ( 139.2950502721270425, 36.88242187608393152, 9.295050272127046043 ) ) ;
#21492=CARTESIAN_POINT ( 'NONE',  ( 74.59884440882045453, 38.22187500216787015, 9.598844408820456309 ) ) ;
#21494=CARTESIAN_POINT ( 'NONE',  ( -13.57481594606304753, 37.08085937716786873, -5.622872871577873077 ) ) ;
#21497=ADVANCED_FACE ( 'NONE', ( #14843 ), #12561, .F. ) ;
#21498=CARTESIAN_POINT ( 'NONE',  ( 185.7049497278729575, 37.47773437608393010, 9.295050272127047819 ) ) ;
#21501=CARTESIAN_POINT ( 'NONE',  ( 124.5550856135277087, 38.81718750108393579, -13.14518615778179722 ) ) ;
#21510=CARTESIAN_POINT ( 'NONE',  ( 195.0000000000000000, 36.43593749999999432, 13.57481594606304576 ) ) ;
#21513=CARTESIAN_POINT ( 'NONE',  ( 55.70494972787295751, 39.85898437608393152, 9.295050272127047819 ) ) ;
#21516=DIRECTION ( 'NONE',  ( 0.000000000000000000, -1.000000000000000000, 0.000000000000000000 ) ) ;
#21519=CARTESIAN_POINT ( 'NONE',  ( 5.622872871577878406, 39.66054687500000142, 13.57481594606304576 ) ) ;
#21520=CARTESIAN_POINT ( 'NONE',  ( 116.8548138422182205, 40.75195312608393294, 0.000000000000000000 ) ) ;
#21521=ORIENTED_EDGE ( 'NONE', *, *, #26203, .F. ) ;
#21522=CARTESIAN_POINT ( 'NONE',  ( 97.92893218813451028, 84.18750000000000000, 4.999999999999989342 ) ) ;
#21526=EDGE_CURVE ( 'NONE', #467, #16116, #3987, .T. ) ;
#21528=CARTESIAN_POINT ( 'NONE',  ( 51.85481384221819923, 35.93984375108393436, -5.444914386472297529 ) ) ;
#21533=ORIENTED_EDGE ( 'NONE', *, *, #15375, .F. ) ;
#21536=CARTESIAN_POINT ( 'NONE',  ( 185.4011555911795313, 36.23750000216787726, -9.598844408820458085 ) ) ;
#21538=CARTESIAN_POINT ( 'NONE',  ( 130.0000000000000000, -7.395377635281828788, -1.503427012513233026E-14 ) ) ;
#21541=CARTESIAN_POINT ( 'NONE',  ( 116.8548138422182205, 40.00781250108393294, 5.444914386472304635 ) ) ;
#21542=ORIENTED_EDGE ( 'NONE', *, *, #294, .F. ) ;
#21543=CARTESIAN_POINT ( 'NONE',  ( 13.14518615778179544, 39.56132812608393579, -1.609821015232357215E-15 ) ) ;
#21544=CARTESIAN_POINT ( 'NONE',  ( 135.4449143864723055, 34.45156250108393436, 13.14518615778179189 ) ) ;
#21545=CARTESIAN_POINT ( 'NONE',  ( 59.37712712842213136, 37.97382812499999716, 13.57481594606304753 ) ) ;
#21548=EDGE_CURVE ( 'NONE', #19008, #1080, #9994, .T. ) ;
#21552=EDGE_CURVE ( 'NONE', #22369, #19690, #21466, .T. ) ;
#21554=DIRECTION ( 'NONE',  ( 0.000000000000000000, 0.000000000000000000, -1.000000000000000000 ) ) ;
#21555=CARTESIAN_POINT ( 'NONE',  ( 95.54126587499996504, 80.75000000136560629, 1.846868145590724986 ) ) ;
#21557=CARTESIAN_POINT ( 'NONE',  ( -13.14518615778179189, 40.00781250108393294, 5.444914386472304635 ) ) ;
#21565=CARTESIAN_POINT ( 'NONE',  ( 204.2950502721270425, 38.46992187608393010, 9.295050272127046043 ) ) ;
#21567=DIRECTION ( 'NONE',  ( -0.000000000000000000, 1.000000000000000000, -0.000000000000000000 ) ) ;
#21568=CARTESIAN_POINT ( 'NONE',  ( 99.99999999999995737, 83.37500000273119838, 4.999999999999990230 ) ) ;
#21569=CARTESIAN_POINT ( 'NONE',  ( 63.11247127412359958, 53.66306546785491349, -14.99999999999999822 ) ) ;
#21570=AXIS2_PLACEMENT_3D ( 'NONE', #15198, #6521, #26343 ) ;
#21575=CARTESIAN_POINT ( 'NONE',  ( 139.5988444088204403, 33.65781250216787157, -9.598844408820458085 ) ) ;
#21576=CARTESIAN_POINT ( 'NONE',  ( 65.00000000000000000, 39.75976562608394005, -13.14518615778179544 ) ) ;
#21578=CARTESIAN_POINT ( 'NONE',  ( 195.0000000000000000, 34.60039062608393579, 13.14518615778179544 ) ) ;
#21580=ORIENTED_EDGE ( 'NONE', *, *, #9846, .T. ) ;
#21585=CARTESIAN_POINT ( 'NONE',  ( 101.8468681455907046, 82.12500000136560629, -4.458734125000016313 ) ) ;
#21586=CARTESIAN_POINT ( 'NONE',  ( 181.8548138422182205, 37.42812500108393436, 5.444914386472304635 ) ) ;
#21589=FACE_OUTER_BOUND ( 'NONE', #5733, .T. ) ;
#21590=CARTESIAN_POINT ( 'NONE',  ( 195.0000000000000000, 40.55351562608393579, -13.14518615778179544 ) ) ;
#21593=AXIS2_PLACEMENT_3D ( 'NONE', #24396, #2877, #18414 ) ;
#21597=CARTESIAN_POINT ( 'NONE',  ( 120.7049497278729575, 37.47773437608393010, -9.295050272127046043 ) ) ;
#21598=CARTESIAN_POINT ( 'NONE',  ( 78.14518615778179367, 33.80664062608393294, -1.609821015232357215E-15 ) ) ;
#21599=CARTESIAN_POINT ( 'NONE',  ( 204.2950502721270425, 37.27929687608394005, -9.295050272127046043 ) ) ;
#21601=CARTESIAN_POINT ( 'NONE',  ( -13.14518615778179544, 36.58476562608393579, 0.000000000000000000 ) ) ;
#21602=CARTESIAN_POINT ( 'NONE',  ( 138.2685973283865621, 50.00000000054347993, -10.78867689284392561 ) ) ;
#21606=CARTESIAN_POINT ( 'NONE',  ( 5.444914386472302859, 38.42031250108393436, 13.14518615778179189 ) ) ;
#21613=CARTESIAN_POINT ( 'NONE',  ( 71.83113445730414526, 36.00000000000000000, 11.35217666746037679 ) ) ;
#21617=CARTESIAN_POINT ( 'NONE',  ( 123.0976214262113047, 51.13402819306929814, 14.99999999999867661 ) ) ;
#21620=CARTESIAN_POINT ( 'NONE',  ( 103.1528011352953342, 83.06250000136560629, 3.152801135295355106 ) ) ;
#21621=CARTESIAN_POINT ( 'NONE',  ( 51.85481384221820633, 34.40195312608393152, 0.000000000000000000 ) ) ;
#21626=CARTESIAN_POINT ( 'NONE',  ( 219.9999999999999716, 80.00000000000000000, 14.99999999999994316 ) ) ;
#21629=CARTESIAN_POINT ( 'NONE',  ( 143.5748159460630688, 39.80937499999999574, -1.662435489736055892E-15 ) ) ;
#21634=CARTESIAN_POINT ( 'NONE',  ( 130.0000000000000000, 35.19570312608392726, 13.14518615778179544 ) ) ;
#21635=CARTESIAN_POINT ( 'NONE',  ( 78.57481594606304043, 32.71523437716787441, 5.622872871577869525 ) ) ;
#21638=VECTOR ( 'NONE', #24343, 1000.000000000000000 ) ;
#21640=CARTESIAN_POINT ( 'NONE',  ( -5.622872871577873077, 36.98164062716787015, -13.57481594606304753 ) ) ;
#21642=ORIENTED_EDGE ( 'NONE', *, *, #4427, .T. ) ;
#21643=CARTESIAN_POINT ( 'NONE',  ( 208.1451861577817795, 37.72578125108393721, 5.444914386472293977 ) ) ;
#21644=VECTOR ( 'NONE', #7263, 999.9999999999998863 ) ;
#21645=CIRCLE ( 'NONE', #21195, 3.000000000000004441 ) ;
#21646=DIRECTION ( 'NONE',  ( -1.000000000000000000, -0.000000000000000000, 2.385244779468110248E-16 ) ) ;
#21654=CARTESIAN_POINT ( 'NONE',  ( 181.4251840539369596, 33.85624999999999574, 0.000000000000000000 ) ) ;
#21656=LINE ( 'NONE', #2132, #19243 ) ;
#21657=CARTESIAN_POINT ( 'NONE',  ( 65.00000000000000000, 37.18007812608393436, -13.14518615778179544 ) ) ;
#21662=CARTESIAN_POINT ( 'NONE',  ( -8.312177448680279460E-16, 36.03906250000000000, -13.57481594606304576 ) ) ;
#21665=ORIENTED_EDGE ( 'NONE', *, *, #15218, .T. ) ;
#21666=CARTESIAN_POINT ( 'NONE',  ( 95.54126587499995082, 79.75000000136560629, 1.846868145590724986 ) ) ;
#21669=ORIENTED_EDGE ( 'NONE', *, *, #27136, .F. ) ;
#21671=CARTESIAN_POINT ( 'NONE',  ( 78.14518615778179367, 36.38632812608393863, -1.609821015232357215E-15 ) ) ;
#21672=ORIENTED_EDGE ( 'NONE', *, *, #2520, .F. ) ;
#21679=( BOUNDED_SURFACE ( )  B_SPLINE_SURFACE ( 1, 2, ( 
 ( #19659, #15515, #2569, #2289, #19948, #13657, #573, #13219, #16986, #17658, #426, #10428, #12701, #8970, #22233, #26219, #22372, #19136, #26365, #24223, #8827, #10948, #2712, #17946, #21951, #9254, #6825, #11231, #4036, #25686, #26657, #4703, #11373, #141, #7104, #17517, #2429, #23559, #20095, #21813, #15802, #13364, #22092, #4849, #9112, #24506, #27842, #17807, #15661, #6169, #4993, #15365, #26510, #6679, #11090, #24081, #4557, #6966, #24361, #19801, #8298, #14836, #284, #13513, #13936, #3274, #13794, #2845, #24789, #15938, #9390, #22663, #27083, #1282, #11802, #20379, #1007, #5417, #2982, #16373, #5697 ),
 ( #12078, #16517, #26945, #7681, #24654, #18086, #3133, #715, #25074, #26798, #18378, #18662, #5562, #1149, #20802, #14225, #20526, #9948, #7247, #5271, #14364, #11514, #22517, #9676, #5127, #7536, #20232, #11656, #864, #27366, #9537, #18236, #7824, #16233, #7388, #16081, #24931, #9816, #14086, #22806, #22946, #11943, #20665, #18522, #27228, #3407, #25209, #16790, #3695, #10639, #18928, #23491, #3971, #14636, #27773, #27910, #23354, #8372, #12488, #1565, #12631, #1699, #28049, #19065, #27636, #19346, #12358, #14911, #25906, #25350, #12773, #21490, #10356, #1971, #21076, #1423, #6376, #8231, #23631, #8516, #10217 ) ),
 .UNSPECIFIED., .F., .F., .F. ) 
 B_SPLINE_SURFACE_WITH_KNOTS ( ( 2, 2 ),
 ( 3, 2, 2, 2, 2, 2, 2, 2, 2, 2, 2, 2, 2, 2, 2, 2, 2, 2, 2, 2, 2, 2, 2, 2, 2, 2, 2, 2, 2, 2, 2, 2, 2, 2, 2, 2, 2, 2, 2, 2, 3 ),
 ( 0.000000000000000000, 1.000000000000000000 ),
 ( 0.000000000000000000, 0.02500000000000000139, 0.05000000000000000278, 0.07499999999999999722, 0.1000000000000000056, 0.1250000000000000000, 0.1499999999999999944, 0.1749999999999999889, 0.2000000000000000111, 0.2250000000000000056, 0.2500000000000000000, 0.2750000000000000222, 0.2999999999999999889, 0.3250000000000000111, 0.3499999999999999778, 0.3750000000000000000, 0.4000000000000000222, 0.4249999999999999889, 0.4500000000000000111, 0.4749999999999999778, 0.5000000000000000000, 0.5250000000000000222, 0.5500000000000000444, 0.5749999999999999556, 0.5999999999999999778, 0.6250000000000000000, 0.6500000000000000222, 0.6750000000000000444, 0.6999999999999999556, 0.7249999999999999778, 0.7500000000000000000, 0.7750000000000000222, 0.8000000000000000444, 0.8249999999999999556, 0.8499999999999999778, 0.8750000000000000000, 0.9000000000000000222, 0.9250000000000000444, 0.9499999999999999556, 0.9749999999999999778, 1.000000000000000000 ),
 .UNSPECIFIED. ) 
 GEOMETRIC_REPRESENTATION_ITEM ( )  RATIONAL_B_SPLINE_SURFACE ( (
 ( 1.000000000000000000, 0.9238795325112867385, 1.000000000000000000, 0.9238795325112867385, 1.000000000000000000, 0.9238795325112867385, 1.000000000000000000, 0.9238795325112867385, 1.000000000000000000, 0.9238795325112867385, 1.000000000000000000, 0.9238795325112867385, 1.000000000000000000, 0.9238795325112867385, 1.000000000000000000, 0.9238795325112867385, 1.000000000000000000, 0.9238795325112867385, 1.000000000000000000, 0.9238795325112867385, 1.000000000000000000, 0.9238795325112867385, 1.000000000000000000, 0.9238795325112867385, 1.000000000000000000, 0.9238795325112867385, 1.000000000000000000, 0.9238795325112867385, 1.000000000000000000, 0.9238795325112867385, 1.000000000000000000, 0.9238795325112867385, 1.000000000000000000, 0.9238795325112867385, 1.000000000000000000, 0.9238795325112867385, 1.000000000000000000, 0.9238795325112867385, 1.000000000000000000, 0.9238795325112867385, 1.000000000000000000, 0.9238795325112867385, 1.000000000000000000, 0.9238795325112867385, 1.000000000000000000, 0.9238795325112867385, 1.000000000000000000, 0.9238795325112867385, 1.000000000000000000, 0.9238795325112867385, 1.000000000000000000, 0.9238795325112867385, 1.000000000000000000, 0.9238795325112867385, 1.000000000000000000, 0.9238795325112867385, 1.000000000000000000, 0.9238795325112867385, 1.000000000000000000, 0.9238795325112867385, 1.000000000000000000, 0.9238795325112867385, 1.000000000000000000, 0.9238795325112867385, 1.000000000000000000, 0.9238795325112867385, 1.000000000000000000, 0.9238795325112867385, 1.000000000000000000, 0.9238795325112867385, 1.000000000000000000, 0.9238795325112867385, 1.000000000000000000, 0.9238795325112867385, 1.000000000000000000, 0.9238795325112867385, 1.000000000000000000, 0.9238795325112867385, 1.000000000000000000, 0.9238795325112867385, 1.000000000000000000),
 ( 1.000000000000000000, 0.9238795325112867385, 1.000000000000000000, 0.9238795325112867385, 1.000000000000000000, 0.9238795325112867385, 1.000000000000000000, 0.9238795325112867385, 1.000000000000000000, 0.9238795325112867385, 1.000000000000000000, 0.9238795325112867385, 1.000000000000000000, 0.9238795325112867385, 1.000000000000000000, 0.9238795325112867385, 1.000000000000000000, 0.9238795325112867385, 1.000000000000000000, 0.9238795325112867385, 1.000000000000000000, 0.9238795325112867385, 1.000000000000000000, 0.9238795325112867385, 1.000000000000000000, 0.9238795325112867385, 1.000000000000000000, 0.9238795325112867385, 1.000000000000000000, 0.9238795325112867385, 1.000000000000000000, 0.9238795325112867385, 1.000000000000000000, 0.9238795325112867385, 1.000000000000000000, 0.9238795325112867385, 1.000000000000000000, 0.9238795325112867385, 1.000000000000000000, 0.9238795325112867385, 1.000000000000000000, 0.9238795325112867385, 1.000000000000000000, 0.9238795325112867385, 1.000000000000000000, 0.9238795325112867385, 1.000000000000000000, 0.9238795325112867385, 1.000000000000000000, 0.9238795325112867385, 1.000000000000000000, 0.9238795325112867385, 1.000000000000000000, 0.9238795325112867385, 1.000000000000000000, 0.9238795325112867385, 1.000000000000000000, 0.9238795325112867385, 1.000000000000000000, 0.9238795325112867385, 1.000000000000000000, 0.9238795325112867385, 1.000000000000000000, 0.9238795325112867385, 1.000000000000000000, 0.9238795325112867385, 1.000000000000000000, 0.9238795325112867385, 1.000000000000000000, 0.9238795325112867385, 1.000000000000000000, 0.9238795325112867385, 1.000000000000000000, 0.9238795325112867385, 1.000000000000000000, 0.9238795325112867385, 1.000000000000000000, 0.9238795325112867385, 1.000000000000000000, 0.9238795325112867385, 1.000000000000000000) ) ) 
 REPRESENTATION_ITEM ( '' )  SURFACE ( )  );
#21681=CARTESIAN_POINT ( 'NONE',  ( 195.0000000000000000, 38.51953125216787299, -13.57481594606304576 ) ) ;
#21684=CARTESIAN_POINT ( 'NONE',  ( 195.3969994146466149, 51.45716825712325004, 14.99999999999927702 ) ) ;
#21685=CARTESIAN_POINT ( 'NONE',  ( 135.4449143864723339, 36.53515625108394715, -13.14518615778179722 ) ) ;
#21686=CARTESIAN_POINT ( 'NONE',  ( -13.14518615778179900, 36.73359375108393010, -5.444914386472297529 ) ) ;
#21687=CARTESIAN_POINT ( 'NONE',  ( 116.8548138422182205, 33.40976562608393863, 0.000000000000000000 ) ) ;
#21688=CARTESIAN_POINT ( 'NONE',  ( 59.37712712842213136, 33.70742187500000142, -13.57481594606304753 ) ) ;
#21699=CARTESIAN_POINT ( 'NONE',  ( 13.14518615778179900, 37.92421875108392726, 5.444914386472293977 ) ) ;
#21701=ORIENTED_EDGE ( 'NONE', *, *, #26904, .F. ) ;
#21703=AXIS2_PLACEMENT_3D ( 'NONE', #563, #18227, #24781 ) ;
#21704=CARTESIAN_POINT ( 'NONE',  ( 116.4251840539369738, 37.18007812716787441, 5.622872871577880183 ) ) ;
#21705=CARTESIAN_POINT ( 'NONE',  ( 185.4011555911795313, 36.13828124999999147, -9.598844408820458085 ) ) ;
#21707=CARTESIAN_POINT ( 'NONE',  ( 195.0000000000000000, 37.57695312608392868, 13.14518615778179544 ) ) ;
#21708=AXIS2_PLACEMENT_3D ( 'NONE', #11957, #16387, #16931 ) ;
#21711=CARTESIAN_POINT ( 'NONE',  ( 96.46446609406721961, 83.25000000273119838, 3.535533905932727539 ) ) ;
#21712=CIRCLE ( 'NONE', #17134, 4.999999999999999112 ) ;
#21714=ORIENTED_EDGE ( 'NONE', *, *, #19063, .T. ) ;
#21719=CARTESIAN_POINT ( 'NONE',  ( 143.1451861577818079, 40.20625000108393010, -5.444914386472297529 ) ) ;
#21720=DIRECTION ( 'NONE',  ( 1.000000000000000000, 0.000000000000000000, -0.000000000000000000 ) ) ;
#21722=VECTOR ( 'NONE', #1207, 1000.000000000000000 ) ;
#21723=CARTESIAN_POINT ( 'NONE',  ( 65.00000000000000000, 40.15664062608393436, 13.14518615778179544 ) ) ;
#21725=CARTESIAN_POINT ( 'NONE',  ( 208.1451861577817795, 34.05468750108394005, -5.444914386472297529 ) ) ;
#21726=ORIENTED_EDGE ( 'NONE', *, *, #26948, .F. ) ;
#21732=CARTESIAN_POINT ( 'NONE',  ( 95.54126587499996504, 81.43750000136559208, -1.387778780781445676E-14 ) ) ;
#21733=CARTESIAN_POINT ( 'NONE',  ( 208.1451861577818079, 37.82500000108392868, -5.444914386472297529 ) ) ;
#21735=CARTESIAN_POINT ( 'NONE',  ( 188.0976214262265671, 51.13402819307177793, 14.99999999999995559 ) ) ;
#21739=EDGE_LOOP ( 'NONE', ( #610, #357, #19385, #1661 ) ) ;
#21742=CLOSED_SHELL ( 'NONE', ( #2167, #1561, #9467, #13270, #25032, #19180, #7242, #3405, #20700, #13993, #27837, #4190, #11393, #16957, #11549, #1205, #7141, #10856, #23786, #16809, #13596, #13522, #20005, #18729, #16999, #3771, #1983, #6044, #25110, #26160, #25397, #16266, #25725, #22421, #7210, #15973, #7898, #23250, #9470, #6208, #25341, #812, #27471, #6362, #23800, #17662, #4499, #12771, #8439, #12616, #27297, #22152, #14883, #5851, #23279, #10674, #10363, #20772, #20833, #21162, #2107, #22941, #21443, #16231, #22921, #9827, #10549, #793, #21011, #277, #4621, #20501, #19294, #23111, #6861, #7251, #2179, #8633, #3009, #19920, #12764, #20461, #13145, #20475, #8835, #12445, #15504, #22390, #24166, #1357, #10149, #13123, #8625, #26421, #16482, #16391, #15449, #14173, #18044, #22236, #8205, #7737, #14384, #26980, #17828, #15051, #4076, #18740, #19938, #7574, #16305, #2252, #20299, #10401, #12260, #21870, #14857, #2499, #3760, #5515, #22868, #9890, #1666, #10519, #26618, #2144, #8721, #96, #5345, #12245, #26082, #16737, #24141, #2393, #26246, #27331, #9867, #15740, #26585, #11064, #3919, #3044, #27086, #21497, #21399, #17841, #15608, #9480, #24458, #16823, #15336, #8094, #25019, #11025 ) ) ;
#21744=CARTESIAN_POINT ( 'NONE',  ( 124.5550856135277087, 36.63437500108393152, -13.14518615778179900 ) ) ;
#21745=CARTESIAN_POINT ( 'NONE',  ( 78.14518615778179367, 32.16953125108393152, 5.444914386472293977 ) ) ;
#21746=CARTESIAN_POINT ( 'NONE',  ( 189.5550856135277229, 36.63437500108393152, -13.14518615778179900 ) ) ;
#21747=DIRECTION ( 'NONE',  ( 0.000000000000000000, 0.000000000000000000, 1.000000000000000000 ) ) ;
#21748=CARTESIAN_POINT ( 'NONE',  ( -13.14518615778179189, 32.66562500108393863, 5.444914386472304635 ) ) ;
#21749=CARTESIAN_POINT ( 'NONE',  ( 126.0201855542024418, 50.00000000123280586, -13.01613927313105634 ) ) ;
#21750=EDGE_CURVE ( 'NONE', #27310, #5488, #16681, .T. ) ;
#21752=LINE ( 'NONE', #24022, #5884 ) ;
#21754=CARTESIAN_POINT ( 'NONE',  ( 5.444914386472297529, 34.74921875108394431, -13.14518615778179900 ) ) ;
#21758=LINE ( 'NONE', #8771, #1790 ) ;
#21760=ORIENTED_EDGE ( 'NONE', *, *, #28145, .F. ) ;
#21763=CARTESIAN_POINT ( 'NONE',  ( 130.3969994146466433, 51.45716825712460007, 15.00000000000097522 ) ) ;
#21765=CARTESIAN_POINT ( 'NONE',  ( 195.0000000000000000, 36.00000000000000000, -2.255140518769849538E-14 ) ) ;
#21766=CARTESIAN_POINT ( 'NONE',  ( 95.54126587499995082, 82.62500000136560629, -1.846868145590750077 ) ) ;
#21767=CARTESIAN_POINT ( 'NONE',  ( 55.70494972787295751, 34.30273437608393294, -9.295050272127046043 ) ) ;
#21770=CARTESIAN_POINT ( 'NONE',  ( 65.00000000000000000, 36.43593749999999432, 13.57481594606304576 ) ) ;
#21773=CARTESIAN_POINT ( 'NONE',  ( 139.5988444088204403, 35.93984374999999432, -9.598844408820458085 ) ) ;
#21778=CARTESIAN_POINT ( 'NONE',  ( 124.5550856135277087, 37.22968750108393721, -13.14518615778179900 ) ) ;
#21779=CARTESIAN_POINT ( 'NONE',  ( 55.40115559117954547, 33.85625000216787583, -9.598844408820458085 ) ) ;
#21782=CARTESIAN_POINT ( 'NONE',  ( 3.878385410779738418, 31.34156310770110565, -13.57481594606304931 ) ) ;
#21787=CARTESIAN_POINT ( 'NONE',  ( 195.0000000000000000, 34.00507812608393721, -13.14518615778179544 ) ) ;
#21788=CARTESIAN_POINT ( 'NONE',  ( 65.00000000000000000, 38.81718749999999574, 13.57481594606304576 ) ) ;
#21797=CARTESIAN_POINT ( 'NONE',  ( 204.5988444088204687, 34.15390624999999858, 9.598844408820456309 ) ) ;
#21800=CARTESIAN_POINT ( 'NONE',  ( 65.00000000000000000, 35.59257812608393579, -13.14518615778179544 ) ) ;
#21801=EDGE_CURVE ( 'NONE', #13724, #5134, #14696, .T. ) ;
#21806=CARTESIAN_POINT ( 'NONE',  ( -13.57481594606304576, 35.49335937499999005, 5.622872871577880183 ) ) ;
#21807=CARTESIAN_POINT ( 'NONE',  ( 143.1451861577818079, 37.22968750108393721, -5.444914386472297529 ) ) ;
#21808=VECTOR ( 'NONE', #3631, 1000.000000000000000 ) ;
#21810=VERTEX_POINT ( 'NONE', #21049 ) ;
#21811=CARTESIAN_POINT ( 'NONE',  ( 103.5355339059327093, 83.37500000000000000, 3.535533905932726206 ) ) ;
#21812=AXIS2_PLACEMENT_3D ( 'NONE', #16806, #12092, #27651 ) ;
#21813=CARTESIAN_POINT ( 'NONE',  ( 104.9999999999999574, 81.68750000273119838, -2.071067811865491937 ) ) ;
#21818=CARTESIAN_POINT ( 'NONE',  ( 70.44491438647230552, 35.44375000108393436, 13.14518615778179189 ) ) ;
#21819=ORIENTED_EDGE ( 'NONE', *, *, #26777, .F. ) ;
#21822=ORIENTED_EDGE ( 'NONE', *, *, #25461, .F. ) ;
#21826=CARTESIAN_POINT ( 'NONE',  ( 208.5748159460630120, 38.27148437716787299, 5.622872871577869525 ) ) ;
#21829=CARTESIAN_POINT ( 'NONE',  ( 120.7049497278729575, 36.08867187608393579, 9.295050272127047819 ) ) ;
#21830=CARTESIAN_POINT ( 'NONE',  ( 13.14518615778179544, 37.18007812608393436, -1.609821015232357215E-15 ) ) ;
#21832=CARTESIAN_POINT ( 'NONE',  ( 135.4449143864723055, 35.24531250108393010, 13.14518615778179189 ) ) ;
#21833=CARTESIAN_POINT ( 'NONE',  ( 78.57481594606305464, 35.04687499999999289, -1.662435489736055892E-15 ) ) ;
#21834=CARTESIAN_POINT ( 'NONE',  ( 51.42518405393695957, 39.51171875216787299, 0.000000000000000000 ) ) ;
#21841=CARTESIAN_POINT ( 'NONE',  ( 103.1528011352953342, 81.06250000136559208, 3.152801135295355106 ) ) ;
#21843=CARTESIAN_POINT ( 'NONE',  ( -5.444914386472297529, 37.42812500108394147, -13.14518615778179900 ) ) ;
#21845=EDGE_LOOP ( 'NONE', ( #462, #22766, #22703, #8976 ) ) ;
#21846=EDGE_CURVE ( 'NONE', #10395, #22131, #22635, .T. ) ;
#21849=( BOUNDED_CURVE ( )  B_SPLINE_CURVE ( 2, ( #12612, #21059, #25889, #6358, #18910 ),
 .UNSPECIFIED., .F., .F. ) 
 B_SPLINE_CURVE_WITH_KNOTS ( ( 3, 2, 3 ),
 ( 0.000000000000000000, 0.01041666666666679446, 0.02083333333333358892 ),
 .UNSPECIFIED. ) 
 CURVE ( )  GEOMETRIC_REPRESENTATION_ITEM ( )  RATIONAL_B_SPLINE_CURVE ( ( 1.000000000000000000, 0.9238795325112867385, 1.000000000000000000, 0.9238795325112848511, 1.000000000000001776 ) ) 
 REPRESENTATION_ITEM ( '' )  );
#21850=CARTESIAN_POINT ( 'NONE',  ( 181.8548138422181921, 39.71015625108393010, -5.444914386472297529 ) ) ;
#21852=CARTESIAN_POINT ( 'NONE',  ( 55.70494972787295751, 36.08867187608393579, 9.295050272127047819 ) ) ;
#21854=CARTESIAN_POINT ( 'NONE',  ( 64.67527568880393574, 53.49346745874647269, -14.99999999999999822 ) ) ;
#21859=CARTESIAN_POINT ( 'NONE',  ( 116.8548138422182063, 40.50390625108394005, -5.444914386472297529 ) ) ;
#21860=CARTESIAN_POINT ( 'NONE',  ( -5.444914386472297529, 39.80937500108393579, -13.14518615778179722 ) ) ;
#21863=CARTESIAN_POINT ( 'NONE',  ( 55.70494972787295751, 37.67617187608393436, 9.295050272127047819 ) ) ;
#21864=CARTESIAN_POINT ( 'NONE',  ( -20.00000000000000355, 80.00000000000000000, -10.00000000000000000 ) ) ;
#21865=CARTESIAN_POINT ( 'NONE',  ( 200.4449143864723055, 35.74140625108393721, -13.14518615778179900 ) ) ;
#21867=ORIENTED_EDGE ( 'NONE', *, *, #24397, .T. ) ;
#21870=ADVANCED_FACE ( 'NONE', ( #14194 ), #20634, .T. ) ;
#21872=CARTESIAN_POINT ( 'NONE',  ( 98.15313185440923860, 81.62500000136560629, 4.458734124999987891 ) ) ;
#21873=CARTESIAN_POINT ( 'NONE',  ( 204.2950502721270425, 38.66835937608393436, -9.295050272127046043 ) ) ;
#21877=LINE ( 'NONE', #2353, #15745 ) ;
#21878=CARTESIAN_POINT ( 'NONE',  ( 65.00000000000000000, 40.00781250000000000, -13.57481594606304576 ) ) ;
#21881=ORIENTED_EDGE ( 'NONE', *, *, #21317, .F. ) ;
#21887=CARTESIAN_POINT ( 'NONE',  ( 130.0000000000000000, 35.79101562608394005, -13.14518615778179544 ) ) ;
#21888=CARTESIAN_POINT ( 'NONE',  ( 74.29505027212704249, 33.90585937608393152, -9.295050272127046043 ) ) ;
#21890=CARTESIAN_POINT ( 'NONE',  ( 181.8548138422181921, 38.42031250108393436, 5.444914386472304635 ) ) ;
#21893=( BOUNDED_CURVE ( )  B_SPLINE_CURVE ( 2, ( #18640, #7515, #14340, #23057, #20920, #27616, #12467, #21192, #1677 ),
 .UNSPECIFIED., .F., .F. ) 
 B_SPLINE_CURVE_WITH_KNOTS ( ( 3, 2, 2, 2, 3 ),
 ( 0.06250000000000004163, 0.07291666666666665741, 0.08333333333333325932, 0.09374999999999987510, 0.1041666666666664909 ),
 .UNSPECIFIED. ) 
 CURVE ( )  GEOMETRIC_REPRESENTATION_ITEM ( )  RATIONAL_B_SPLINE_CURVE ( ( 0.9999999999999996669, 0.9238795325112870716, 1.000000000000000000, 0.9238795325112867385, 1.000000000000000000, 0.9238795325112867385, 1.000000000000000000, 0.9238795325112880708, 0.9999999999999986677 ) ) 
 REPRESENTATION_ITEM ( '' )  );
#21894=CARTESIAN_POINT ( 'NONE',  ( -13.14518615778179189, 33.45937500108392726, 5.444914386472304635 ) ) ;
#21897=DIRECTION ( 'NONE',  ( 0.000000000000000000, 0.000000000000000000, -1.000000000000000000 ) ) ;
#21899=CARTESIAN_POINT ( 'NONE',  ( 0.3247243111960362305, 53.49346745874646558, 14.99999999999999822 ) ) ;
#21900=CARTESIAN_POINT ( 'NONE',  ( 99.99999999999995737, 79.37500000273119838, 4.999999999999990230 ) ) ;
#21907=CARTESIAN_POINT ( 'NONE',  ( 129.1610731307196147, 53.50081894914377045, 14.99999999999996447 ) ) ;
#21910=CARTESIAN_POINT ( 'NONE',  ( 96.84719886470459471, 82.81250000136560629, 3.152801135295355994 ) ) ;
#21911=CARTESIAN_POINT ( 'NONE',  ( 55.70494972787295751, 36.68398437608393436, -9.295050272127046043 ) ) ;
#21913=CARTESIAN_POINT ( 'NONE',  ( -5.444914386472299306, 37.52734375108393294, 13.14518615778179722 ) ) ;
#21915=CARTESIAN_POINT ( 'NONE',  ( 124.3771271284221029, 36.08867187500000284, -13.57481594606300135 ) ) ;
#21917=CARTESIAN_POINT ( 'NONE',  ( 124.3771271284221314, 37.18007812500000853, 13.57481594606304753 ) ) ;
#21918=EDGE_CURVE ( 'NONE', #1909, #16468, #5527, .T. ) ;
#21923=CARTESIAN_POINT ( 'NONE',  ( 135.4449143864723055, 35.54296875108393294, -13.14518615778179900 ) ) ;
#21924=CARTESIAN_POINT ( 'NONE',  ( 59.37712712842213136, 33.01289062716787726, -13.57481594606304753 ) ) ;
#21926=CARTESIAN_POINT ( 'NONE',  ( -13.14518615778179900, 40.50390625108394005, -5.444914386472297529 ) ) ;
#21929=CARTESIAN_POINT ( 'NONE',  ( 181.8548138422181921, 33.45937500108392726, 5.444914386472304635 ) ) ;
#21932=DIRECTION ( 'NONE',  ( 0.000000000000000000, 0.000000000000000000, 1.000000000000000000 ) ) ;
#21935=CARTESIAN_POINT ( 'NONE',  ( 139.1801758136479918, 55.00000000000000000, 14.99999999999996270 ) ) ;
#21940=CARTESIAN_POINT ( 'NONE',  ( 208.5748159460630120, 35.89023437499999858, -5.622872871577873077 ) ) ;
#21943=CARTESIAN_POINT ( 'NONE',  ( 59.55508561352770158, 35.64218750108392442, -13.14518615778179900 ) ) ;
#21946=CARTESIAN_POINT ( 'NONE',  ( 130.0000000000000000, -7.395377635281828788, -13.57481594606305997 ) ) ;
#21947=CARTESIAN_POINT ( 'NONE',  ( -9.598844408820458085, 36.93203124999999432, -9.598844408820458085 ) ) ;
#21948=CARTESIAN_POINT ( 'NONE',  ( 130.0000000000000000, 36.98164062608393721, 13.14518615778179544 ) ) ;
#21949=VERTEX_POINT ( 'NONE', #3666 ) ;
#21950=CARTESIAN_POINT ( 'NONE',  ( 104.9999999999999574, 82.56250000000002842, -2.071067811865491937 ) ) ;
#21951=CARTESIAN_POINT ( 'NONE',  ( 104.9999999999999716, 82.62500000273119838, -1.449011120738813565E-14 ) ) ;
#21953=CARTESIAN_POINT ( 'NONE',  ( 52.43349327520137138, 36.00000000000001421, -4.295155080288876270 ) ) ;
#21955=CARTESIAN_POINT ( 'NONE',  ( 70.44491438647230552, 32.26875000108393721, 13.14518615778179189 ) ) ;
#21959=ORIENTED_EDGE ( 'NONE', *, *, #19889, .T. ) ;
#21962=CARTESIAN_POINT ( 'NONE',  ( 204.5988444088204687, 34.25312500216787015, 9.598844408820456309 ) ) ;
#21964=VERTEX_POINT ( 'NONE', #12328 ) ;
#21967=LINE ( 'NONE', #20111, #15249 ) ;
#21968=CARTESIAN_POINT ( 'NONE',  ( 2.414731522848535132E-15, 35.39414062608393863, 13.14518615778179544 ) ) ;
#21969=CARTESIAN_POINT ( 'NONE',  ( 143.1451861577818079, 35.44375000108393436, -5.444914386472297529 ) ) ;
#21970=CARTESIAN_POINT ( 'NONE',  ( 70.62287287157788285, 34.10429687499999574, 13.57481594606304576 ) ) ;
#21979=CARTESIAN_POINT ( 'NONE',  ( -8.049105076161786076E-16, 35.79101562608394005, -13.14518615778179544 ) ) ;
#21981=VERTEX_POINT ( 'NONE', #10184 ) ;
#21983=CARTESIAN_POINT ( 'NONE',  ( 195.0000000000000000, 36.43593749999999432, 13.57481594606304576 ) ) ;
#21984=CARTESIAN_POINT ( 'NONE',  ( 195.0000000000000000, 39.95820312608393010, 13.14518615778179544 ) ) ;
#21987=DIRECTION ( 'NONE',  ( 0.000000000000000000, 1.000000000000000000, 0.000000000000000000 ) ) ;
#21994=VECTOR ( 'NONE', #23442, 1000.000000000000000 ) ;
#21995=CARTESIAN_POINT ( 'NONE',  ( 143.1451861577818079, 40.15664062608393436, -1.609821015232357215E-15 ) ) ;
#21998=CARTESIAN_POINT ( 'NONE',  ( 55.70494972787295751, 36.68398437608393436, -9.295050272127046043 ) ) ;
#22001=CARTESIAN_POINT ( 'NONE',  ( 208.1451861577817795, 36.33671875108394289, 5.444914386472293977 ) ) ;
#22006=CARTESIAN_POINT ( 'NONE',  ( 74.29505027212704249, 40.25585937608393294, -9.295050272127046043 ) ) ;
#22007=CARTESIAN_POINT ( 'NONE',  ( 99.99999999999995737, 79.68750000136559208, 4.458734124999988779 ) ) ;
#22008=CARTESIAN_POINT ( 'NONE',  ( 189.5550856135277229, 38.02343750108394005, -13.14518615778179722 ) ) ;
#22014=ORIENTED_EDGE ( 'NONE', *, *, #15137, .F. ) ;
#22015=EDGE_CURVE ( 'NONE', #28147, #16548, #2888, .T. ) ;
#22018=VERTEX_POINT ( 'NONE', #19032 ) ;
#22019=CARTESIAN_POINT ( 'NONE',  ( 120.7049497278729575, 34.50117187608393721, 9.295050272127047819 ) ) ;
#22020=CARTESIAN_POINT ( 'NONE',  ( 78.14518615778179367, 32.96328125108393436, 5.444914386472293977 ) ) ;
#22021=CARTESIAN_POINT ( 'NONE',  ( 181.8548138422181921, 36.73359375108393010, -5.444914386472297529 ) ) ;
#22022=ORIENTED_EDGE ( 'NONE', *, *, #4430, .F. ) ;
#22023=CARTESIAN_POINT ( 'NONE',  ( 62.70203941399186931, 36.00000000000001421, 12.97104423350682900 ) ) ;
#22024=CARTESIAN_POINT ( 'NONE',  ( -8.049105076161786076E-16, 32.41757812608393863, -13.14518615778179544 ) ) ;
#22025=CARTESIAN_POINT ( 'NONE',  ( 127.4704160048206205, 49.99999999938359707, -13.34625891065716807 ) ) ;
#22026=EDGE_CURVE ( 'NONE', #4003, #3976, #1943, .T. ) ;
#22028=DIRECTION ( 'NONE',  ( -1.000000000000000000, 0.000000000000000000, 7.228014483236696740E-18 ) ) ;
#22030=LINE ( 'NONE', #3072, #3358 ) ;
#22036=ORIENTED_EDGE ( 'NONE', *, *, #22026, .T. ) ;
#22039=CARTESIAN_POINT ( 'NONE',  ( 121.2416656076439949, 50.00000000000000000, 10.38725784494027238 ) ) ;
#22040=EDGE_CURVE ( 'NONE', #6189, #25739, #8025, .T. ) ;
#22043=CYLINDRICAL_SURFACE ( 'NONE', #2852, 11.57481594606304398 ) ;
#22044=CARTESIAN_POINT ( 'NONE',  ( 59.55508561352770158, 33.75703125108393721, 13.14518615778179722 ) ) ;
#22046=CARTESIAN_POINT ( 'NONE',  ( 5.444914386472302859, 36.83281250108392868, 13.14518615778179189 ) ) ;
#22047=VECTOR ( 'NONE', #18825, 1000.000000000000000 ) ;
#22051=CARTESIAN_POINT ( 'NONE',  ( 103.5355339059327093, 82.37500000000000000, 3.535533905932726206 ) ) ;
#22052=CARTESIAN_POINT ( 'NONE',  ( 135.6228728715778971, 38.07304687499998863, 13.57481594606304576 ) ) ;
#22059=CARTESIAN_POINT ( 'NONE',  ( 143.1451861577818079, 36.18789062608393436, -1.609821015232357215E-15 ) ) ;
#22060=CARTESIAN_POINT ( 'NONE',  ( 78.57481594606304043, 35.19570312716788152, -5.622872871577873077 ) ) ;
#22062=VERTEX_POINT ( 'NONE', #1667 ) ;
#22064=CARTESIAN_POINT ( 'NONE',  ( 13.57481594606304753, 32.81445312716787299, -5.622872871577873077 ) ) ;
#22069=CARTESIAN_POINT ( 'NONE',  ( 181.8548138422182205, 35.79101562608393294, 0.000000000000000000 ) ) ;
#22072=CARTESIAN_POINT ( 'NONE',  ( 0.000000000000000000, -7.395377635281828788, 0.000000000000000000 ) ) ;
#22073=CARTESIAN_POINT ( 'NONE',  ( 130.0000000000000000, 36.13828125216787157, -13.57481594606304576 ) ) ;
#22079=CARTESIAN_POINT ( 'NONE',  ( 208.5748159460630120, 33.40976562499999858, 5.622872871577869525 ) ) ;
#22082=CARTESIAN_POINT ( 'NONE',  ( 59.55508561352770158, 34.84843750108393579, -13.14518615778179900 ) ) ;
#22086=CARTESIAN_POINT ( 'NONE',  ( -5.622872871577873077, 34.79882812499998579, 13.57481594606304753 ) ) ;
#22087=CARTESIAN_POINT ( 'NONE',  ( 120.7049497278729575, 39.26367187608393294, 9.295050272127047819 ) ) ;
#22089=CARTESIAN_POINT ( 'NONE',  ( 96.46446609406721961, 84.12500000000000000, 3.535533905932727539 ) ) ;
#22090=VECTOR ( 'NONE', #16439, 1000.000000000000000 ) ;
#22091=CARTESIAN_POINT ( 'NONE',  ( 195.0000000000000000, 36.93203125216787441, -13.57481594606304576 ) ) ;
#22092=CARTESIAN_POINT ( 'NONE',  ( 103.5355339059327093, 81.50000000273119838, 3.535533905932726206 ) ) ;
#22095=( BOUNDED_CURVE ( )  B_SPLINE_CURVE ( 2, ( #7906, #14449, #25153, #21303, #23028, #3918, #27584, #16740, #1785 ),
 .UNSPECIFIED., .F., .F. ) 
 B_SPLINE_CURVE_WITH_KNOTS ( ( 3, 2, 2, 2, 3 ),
 ( 0.2708333333333330928, 0.2812499999999998890, 0.2916666666666666852, 0.3020833333333334259, 0.3125000000000002220 ),
 .UNSPECIFIED. ) 
 CURVE ( )  GEOMETRIC_REPRESENTATION_ITEM ( )  RATIONAL_B_SPLINE_CURVE ( ( 1.000000000000001554, 0.9238795325112850731, 1.000000000000000000, 0.9238795325112867385, 1.000000000000000000, 0.9238795325112867385, 1.000000000000000000, 0.9238795325112850731, 1.000000000000001554 ) ) 
 REPRESENTATION_ITEM ( '' )  );
#22097=CARTESIAN_POINT ( 'NONE',  ( 78.57481594606305464, 40.60312499999999858, -1.662435489736055892E-15 ) ) ;
#22098=ORIENTED_EDGE ( 'NONE', *, *, #1705, .T. ) ;
#22102=ORIENTED_EDGE ( 'NONE', *, *, #25973, .T. ) ;
#22105=CARTESIAN_POINT ( 'NONE',  ( 204.5988444088204687, 33.45937500216787441, 9.598844408820456309 ) ) ;
#22107=CARTESIAN_POINT ( 'NONE',  ( 206.1048480505471048, 36.02027164848243501, -8.092840767093784748 ) ) ;
#22108=CARTESIAN_POINT ( 'NONE',  ( 200.6228728715779539, 38.46992187716787726, -13.57481594606299247 ) ) ;
#22109=CARTESIAN_POINT ( 'NONE',  ( 5.444914386472297529, 34.94765625108394147, -13.14518615778179900 ) ) ;
#22110=CARTESIAN_POINT ( 'NONE',  ( 116.8548138422182205, 35.79101562608393294, 0.000000000000000000 ) ) ;
#22111=CARTESIAN_POINT ( 'NONE',  ( 74.59884440882045453, 35.74140624999999716, 9.598844408820456309 ) ) ;
#22114=CARTESIAN_POINT ( 'NONE',  ( 208.4955014123170827, 35.99999999999996447, -0.9550757908099977156 ) ) ;
#22118=AXIS2_PLACEMENT_3D ( 'NONE', #5861, #14660, #12241 ) ;
#22119=CARTESIAN_POINT ( 'NONE',  ( 99.99999999999995737, 83.37500000273119838, 4.999999999999990230 ) ) ;
#22121=CARTESIAN_POINT ( 'NONE',  ( 13.14518615778179900, 37.13046875108393863, 5.444914386472293977 ) ) ;
#22126=DIRECTION ( 'NONE',  ( -0.000000000000000000, 1.000000000000000000, -0.000000000000000000 ) ) ;
#22127=CARTESIAN_POINT ( 'NONE',  ( 208.1451861577817795, 36.93203125108394147, 5.444914386472293977 ) ) ;
#22129=CARTESIAN_POINT ( 'NONE',  ( 13.57481594606304576, 39.90859375216787441, -1.662435489736055892E-15 ) ) ;
#22131=VERTEX_POINT ( 'NONE', #19597 ) ;
#22133=CARTESIAN_POINT ( 'NONE',  ( 99.99999999999995737, 83.87500000273119838, -5.000000000000018652 ) ) ;
#22134=CIRCLE ( 'NONE', #25765, 5.000000000000000000 ) ;
#22136=CARTESIAN_POINT ( 'NONE',  ( 116.8548138422182205, 40.55351562608393579, 0.000000000000000000 ) ) ;
#22137=CARTESIAN_POINT ( 'NONE',  ( 13.14518615778179722, 39.61093750108393863, -5.444914386472297529 ) ) ;
#22139=CARTESIAN_POINT ( 'NONE',  ( 51.85481384221820633, 36.83281250108393579, 5.444914386472304635 ) ) ;
#22140=CARTESIAN_POINT ( 'NONE',  ( 56.74038847111184936, 50.00000000056339644, -10.79618466885979799 ) ) ;
#22141=CARTESIAN_POINT ( 'NONE',  ( 185.4011555911795597, 40.30546874999999574, 9.598844408820459861 ) ) ;
#22142=CARTESIAN_POINT ( 'NONE',  ( 70.62287287157776916, 38.37070312499999858, -13.57481594606313990 ) ) ;
#22149=CARTESIAN_POINT ( 'NONE',  ( 208.1451861577818079, 37.72578125108393010, 5.444914386472293977 ) ) ;
#22152=ADVANCED_FACE ( 'NONE', ( #27743 ), #13838, .T. ) ;
#22156=CARTESIAN_POINT ( 'NONE',  ( 185.7049497278729575, 39.06523437608392868, -9.295050272127046043 ) ) ;
#22162=CARTESIAN_POINT ( 'NONE',  ( 143.1451861577818079, 33.95546875108393436, 5.444914386472293977 ) ) ;
#22163=CARTESIAN_POINT ( 'NONE',  ( 78.14518615778179367, 33.85625000108393579, -5.444914386472297529 ) ) ;
#22164=CARTESIAN_POINT ( 'NONE',  ( 200.4449143864723055, 37.32890625108393579, -13.14518615778179900 ) ) ;
#22167=CARTESIAN_POINT ( 'NONE',  ( 5.444914386472297529, 33.95546875108393436, -13.14518615778179900 ) ) ;
#22170=CARTESIAN_POINT ( 'NONE',  ( 116.4251840539369596, 39.56132812716787583, 5.622872871577880183 ) ) ;
#22173=CARTESIAN_POINT ( 'NONE',  ( 130.0000000000000000, 38.02343749999999289, 13.57481594606304576 ) ) ;
#22174=CARTESIAN_POINT ( 'NONE',  ( 200.4449143864723055, 39.71015625108393010, -13.14518615778179900 ) ) ;
#22177=ORIENTED_EDGE ( 'NONE', *, *, #13399, .T. ) ;
#22182=CARTESIAN_POINT ( 'NONE',  ( 65.00000000000000000, 39.31328125216787583, -13.57481594606304576 ) ) ;
#22183=CARTESIAN_POINT ( 'NONE',  ( 96.84719886470459471, 81.56250000136559208, -3.152801135295383084 ) ) ;
#22184=CARTESIAN_POINT ( 'NONE',  ( 51.85481384221820633, 35.98945312608393721, 0.000000000000000000 ) ) ;
#22186=CARTESIAN_POINT ( 'NONE',  ( -8.049105076161786076E-16, 38.76757812608393294, -13.14518615778179544 ) ) ;
#22188=CARTESIAN_POINT ( 'NONE',  ( -6.902378573780346471, 51.13402819306926261, 15.00000000000000178 ) ) ;
#22190=CARTESIAN_POINT ( 'NONE',  ( 139.5988444088204403, 36.73359374999999716, -9.598844408820458085 ) ) ;
#22192=ORIENTED_EDGE ( 'NONE', *, *, #21750, .F. ) ;
#22193=PLANE ( 'NONE',  #14480 ) ;
#22198=CARTESIAN_POINT ( 'NONE',  ( 130.0000000000000000, 32.41757812608393863, -13.14518615778179544 ) ) ;
#22199=CARTESIAN_POINT ( 'NONE',  ( 55.40115559117954547, 34.84843750216787583, 9.598844408820459861 ) ) ;
#22202=CARTESIAN_POINT ( 'NONE',  ( -13.57481594606304576, 33.16171875216787868, 0.000000000000000000 ) ) ;
#22204=CARTESIAN_POINT ( 'NONE',  ( -15.00000000000000000, 55.00000000000000000, 15.00000000000000178 ) ) ;
#22206=CARTESIAN_POINT ( 'NONE',  ( 208.1451861577817795, 33.06250000108393294, -5.444914386472297529 ) ) ;
#22207=CARTESIAN_POINT ( 'NONE',  ( -20.00000000000000000, 75.00000000000000000, 10.00000000000000000 ) ) ;
#22208=DIRECTION ( 'NONE',  ( 0.000000000000000000, 0.000000000000000000, -1.000000000000000000 ) ) ;
#22215=( BOUNDED_CURVE ( )  B_SPLINE_CURVE ( 2, ( #26448, #8907, #9054, #366, #11452, #13158, #26592, #17886, #222 ),
 .UNSPECIFIED., .F., .F. ) 
 B_SPLINE_CURVE_WITH_KNOTS ( ( 3, 2, 2, 2, 3 ),
 ( 0.02083333333333358892, 0.03125000000000020123, 0.04166666666666681007, 0.05208333333333342585, 0.06250000000000004163 ),
 .UNSPECIFIED. ) 
 CURVE ( )  GEOMETRIC_REPRESENTATION_ITEM ( )  RATIONAL_B_SPLINE_CURVE ( ( 0.9999999999999981126, 0.9238795325112886259, 1.000000000000000000, 0.9238795325112867385, 1.000000000000000000, 0.9238795325112867385, 1.000000000000000000, 0.9238795325112864054, 1.000000000000000222 ) ) 
 REPRESENTATION_ITEM ( '' )  );
#22218=CARTESIAN_POINT ( 'NONE',  ( 181.4251840539369596, 34.64999999999999147, 0.000000000000000000 ) ) ;
#22221=CARTESIAN_POINT ( 'NONE',  ( 135.6228728715780107, 36.78320312499999289, -13.57481594606290898 ) ) ;
#22222=CARTESIAN_POINT ( 'NONE',  ( 74.29505027212704249, 36.88242187608393152, 9.295050272127046043 ) ) ;
#22226=EDGE_CURVE ( 'NONE', #21433, #21442, #22563, .T. ) ;
#22228=CARTESIAN_POINT ( 'NONE',  ( 5.622872871577878406, 36.48554687499999716, 13.57481594606304576 ) ) ;
#22229=CARTESIAN_POINT ( 'NONE',  ( 143.1451861577818079, 37.97382812608393721, -1.609821015232357215E-15 ) ) ;
#22233=CARTESIAN_POINT ( 'NONE',  ( 96.46446609406721961, 83.25000000273119838, 3.535533905932727539 ) ) ;
#22236=ADVANCED_FACE ( 'NONE', ( #13157 ), #16129, .T. ) ;
#22237=AXIS2_PLACEMENT_3D ( 'NONE', #14908, #23629, #15331 ) ;
#22239=CARTESIAN_POINT ( 'NONE',  ( 70.62287287157786864, 39.95820312499999716, -13.57481594606304753 ) ) ;
#22243=EDGE_CURVE ( 'NONE', #20676, #16151, #9579, .T. ) ;
#22246=CARTESIAN_POINT ( 'NONE',  ( 181.4251840539369596, 34.74921875216787726, 0.000000000000000000 ) ) ;
#22249=DIRECTION ( 'NONE',  ( 0.000000000000000000, 1.000000000000000000, 0.000000000000000000 ) ) ;
#22250=CARTESIAN_POINT ( 'NONE',  ( 139.2950502721270425, 37.08085937608393579, 9.295050272127046043 ) ) ;
#22251=CARTESIAN_POINT ( 'NONE',  ( 13.14518615778179900, 34.74921875108395142, 5.444914386472293977 ) ) ;
#22252=CARTESIAN_POINT ( 'NONE',  ( 143.1451861577818079, 33.06250000108393294, -5.444914386472297529 ) ) ;
#22253=CARTESIAN_POINT ( 'NONE',  ( 74.59884440882045453, 33.36015624999999574, 9.598844408820456309 ) ) ;
#22255=CIRCLE ( 'NONE', #17229, 13.57481594606304398 ) ;
#22256=VECTOR ( 'NONE', #20102, 1000.000000000000000 ) ;
#22261=VECTOR ( 'NONE', #23154, 1000.000000000000227 ) ;
#22263=CARTESIAN_POINT ( 'NONE',  ( 181.4251840539369596, 40.99999999999999289, 0.000000000000000000 ) ) ;
#22265=CARTESIAN_POINT ( 'NONE',  ( -9.295050272127044266, 36.88242187608393152, 9.295050272127047819 ) ) ;
#22268=FACE_OUTER_BOUND ( 'NONE', #4854, .T. ) ;
#22273=CARTESIAN_POINT ( 'NONE',  ( 195.0000000000000000, 35.19570312608392726, 13.14518615778179544 ) ) ;
#22275=CARTESIAN_POINT ( 'NONE',  ( 194.6752756888038505, 53.49346745874645137, -14.99999999999999822 ) ) ;
#22281=CARTESIAN_POINT ( 'NONE',  ( 124.5550856135277087, 39.61093750108393152, -13.14518615778179900 ) ) ;
#22283=CARTESIAN_POINT ( 'NONE',  ( 2.414731522848535132E-15, 35.98945312608393010, 13.14518615778179544 ) ) ;
#22285=CARTESIAN_POINT ( 'NONE',  ( 51.85481384221820633, 37.62656250108393863, 5.444914386472304635 ) ) ;
#22286=CARTESIAN_POINT ( 'NONE',  ( 56.60406125870027694, 54.99999999495823033, -15.00000000000000000 ) ) ;
#22288=CARTESIAN_POINT ( 'NONE',  ( 189.3771271284221314, 39.56132812499999574, 13.57481594606304753 ) ) ;
#22289=CARTESIAN_POINT ( 'NONE',  ( 99.99999999999995737, 85.00000000000000000, -1.387778780781445676E-14 ) ) ;
#22292=CARTESIAN_POINT ( 'NONE',  ( 70.44491438647229131, 36.83281250108392868, 13.14518615778179189 ) ) ;
#22293=CYLINDRICAL_SURFACE ( 'NONE', #1976, 13.57481594606304398 ) ;
#22294=CARTESIAN_POINT ( 'NONE',  ( 185.7049497278729575, 36.68398437608392726, 9.295050272127047819 ) ) ;
#22295=ORIENTED_EDGE ( 'NONE', *, *, #10321, .F. ) ;
#22299=CARTESIAN_POINT ( 'NONE',  ( 195.0000000000000000, 37.37851562608393863, -13.14518615778179544 ) ) ;
#22301=VERTEX_POINT ( 'NONE', #24836 ) ;
#22305=CARTESIAN_POINT ( 'NONE',  ( 143.1451861577818079, 33.21132812608393436, -1.609821015232357215E-15 ) ) ;
#22306=CARTESIAN_POINT ( 'NONE',  ( 74.29505027212704249, 40.25585937608393294, 9.295050272127046043 ) ) ;
#22308=CARTESIAN_POINT ( 'NONE',  ( 181.8548138422182205, 34.40195312608393152, 0.000000000000000000 ) ) ;
#22309=ORIENTED_EDGE ( 'NONE', *, *, #10510, .T. ) ;
#22311=CARTESIAN_POINT ( 'NONE',  ( -5.444914386472299306, 31.97109375108393436, 13.14518615778179722 ) ) ;
#22312=CARTESIAN_POINT ( 'NONE',  ( -13.36000105192242060, 40.87597656304196647, 0.000000000000000000 ) ) ;
#22316=FACE_OUTER_BOUND ( 'NONE', #14051, .T. ) ;
#22318=CARTESIAN_POINT ( 'NONE',  ( 200.4449143864723055, 40.50390625108394005, -13.14518615778179900 ) ) ;
#22320=ORIENTED_EDGE ( 'NONE', *, *, #3063, .F. ) ;
#22325=CARTESIAN_POINT ( 'NONE',  ( 139.1801758136480203, 50.00000000000000000, 14.99999999999996980 ) ) ;
#22327=CARTESIAN_POINT ( 'NONE',  ( 195.0000000000000000, 40.00781250000000000, -13.57481594606304576 ) ) ;
#22328=CARTESIAN_POINT ( 'NONE',  ( 70.62287287157778337, 37.37851562716787157, 13.57481594606313813 ) ) ;
#22332=CARTESIAN_POINT ( 'NONE',  ( 13.14518615778179722, 38.51953125108393294, 5.444914386472293977 ) ) ;
#22333=LINE ( 'NONE', #11893, #5745 ) ;
#22334=CARTESIAN_POINT ( 'NONE',  ( 0.9830651850993362695, 49.99999999949037033, 13.54930971656776073 ) ) ;
#22336=CARTESIAN_POINT ( 'NONE',  ( 116.4251840539369596, 36.28710937499999289, 5.622872871577880183 ) ) ;
#22342=CARTESIAN_POINT ( 'NONE',  ( 116.8548138422182063, 34.15390625108393863, -5.444914386472297529 ) ) ;
#22343=CARTESIAN_POINT ( 'NONE',  ( 51.85481384221820633, 39.80937500108392868, 5.444914386472304635 ) ) ;
#22345=CARTESIAN_POINT ( 'NONE',  ( -9.598844408820458085, 33.06250000216787299, -9.598844408820458085 ) ) ;
#22349=CARTESIAN_POINT ( 'NONE',  ( 208.1451861577817795, 34.55078125108393294, 5.444914386472293977 ) ) ;
#22351=CARTESIAN_POINT ( 'NONE',  ( 208.5748159460630688, 39.06523437499999574, -5.622872871577873966 ) ) ;
#22354=CARTESIAN_POINT ( 'NONE',  ( 130.0000000000000000, 38.42031249999999432, -13.57481594606304576 ) ) ;
#22360=CARTESIAN_POINT ( 'NONE',  ( 13.57481594606304931, 36.58476562499999574, 5.622872871577868636 ) ) ;
#22361=CARTESIAN_POINT ( 'NONE',  ( 101.8468681455906903, 82.12500000136560629, -4.458734125000016313 ) ) ;
#22362=CARTESIAN_POINT ( 'NONE',  ( 65.00000000000000000, 34.40195312608393152, 13.14518615778179544 ) ) ;
#22364=CARTESIAN_POINT ( 'NONE',  ( 195.0000000000000000, -7.395377635281828788, 13.57481594606302266 ) ) ;
#22367=CARTESIAN_POINT ( 'NONE',  ( -5.622872871577873077, 32.41757812499999858, 13.57481594606304753 ) ) ;
#22368=CARTESIAN_POINT ( 'NONE',  ( 124.5550856135277087, 36.93203125108394147, 13.14518615778179722 ) ) ;
#22369=VERTEX_POINT ( 'NONE', #26846 ) ;
#22372=CARTESIAN_POINT ( 'NONE',  ( 94.99999999999995737, 83.12500000273119838, -1.387778780781445676E-14 ) ) ;
#22374=DIRECTION ( 'NONE',  ( -0.000000000000000000, 1.000000000000000000, -0.000000000000000000 ) ) ;
#22375=EDGE_CURVE ( 'NONE', #16116, #25435, #10704, .T. ) ;
#22377=CARTESIAN_POINT ( 'NONE',  ( 74.29505027212704249, 32.51679687608393721, -9.295050272127046043 ) ) ;
#22378=ORIENTED_EDGE ( 'NONE', *, *, #8261, .T. ) ;
#22383=CARTESIAN_POINT ( 'NONE',  ( 185.4011555911795597, 34.84843750216787583, 9.598844408820459861 ) ) ;
#22388=CARTESIAN_POINT ( 'NONE',  ( 208.5748159460630688, 38.27148437716787299, 5.622872871577868636 ) ) ;
#22389=CARTESIAN_POINT ( 'NONE',  ( 13.14518615778179544, 36.38632812608393863, -1.609821015232357215E-15 ) ) ;
#22390=ADVANCED_FACE ( 'NONE', ( #1193 ), #24163, .T. ) ;
#22391=CARTESIAN_POINT ( 'NONE',  ( 136.9444237971526945, 31.55306878032414986, -11.16113333171310451 ) ) ;
#22392=CARTESIAN_POINT ( 'NONE',  ( 55.40115559117954547, 32.36796874999999574, 9.598844408820459861 ) ) ;
#22395=CARTESIAN_POINT ( 'NONE',  ( 78.57481594606305464, 36.78320312716788010, -5.622872871577873966 ) ) ;
#22397=CARTESIAN_POINT ( 'NONE',  ( 195.0000000000000000, 38.81718749999999574, 13.57481594606304576 ) ) ;
#22403=CARTESIAN_POINT ( 'NONE',  ( 13.14518615778179544, 34.79882812608394005, -1.609821015232357215E-15 ) ) ;
#22405=ORIENTED_EDGE ( 'NONE', *, *, #13687, .T. ) ;
#22409=CARTESIAN_POINT ( 'NONE',  ( 195.0000000000000000, 36.38632812608393152, -13.14518615778179544 ) ) ;
#22411=DIRECTION ( 'NONE',  ( -0.000000000000000000, -1.000000000000000000, -0.000000000000000000 ) ) ;
#22413=EDGE_CURVE ( 'NONE', #9474, #16468, #25286, .T. ) ;
#22418=CARTESIAN_POINT ( 'NONE',  ( 130.0000000000000000, 37.57695312608392868, 13.14518615778179544 ) ) ;
#22419=CARTESIAN_POINT ( 'NONE',  ( 13.14518615778179722, 37.22968750108394431, -5.444914386472297529 ) ) ;
#22420=CARTESIAN_POINT ( 'NONE',  ( 9.295050272127046043, 34.69960937608393436, -9.295050272127046043 ) ) ;
#22421=ADVANCED_FACE ( 'NONE', ( #14237 ), #7695, .T. ) ;
#22423=CARTESIAN_POINT ( 'NONE',  ( 70.36549656804798758, 54.48174559707608466, -15.00000000000000000 ) ) ;
#22426=AXIS2_PLACEMENT_3D ( 'NONE', #11636, #18215, #18503 ) ;
#22427=CARTESIAN_POINT ( 'NONE',  ( 208.5748159460630688, 40.60312499999999858, -1.662435489736055892E-15 ) ) ;
#22430=ORIENTED_EDGE ( 'NONE', *, *, #5622, .T. ) ;
#22433=CARTESIAN_POINT ( 'NONE',  ( 51.85481384221820633, 38.12265625108393863, -5.444914386472297529 ) ) ;
#22441=CARTESIAN_POINT ( 'NONE',  ( 208.1451861577818079, 37.22968750108394431, -5.444914386472297529 ) ) ;
#22447=CARTESIAN_POINT ( 'NONE',  ( 130.0000000000000000, 34.60039062608393579, 13.14518615778179544 ) ) ;
#22449=CARTESIAN_POINT ( 'NONE',  ( 204.2950502721270425, 35.69179687608394147, -9.295050272127046043 ) ) ;
#22452=CARTESIAN_POINT ( 'NONE',  ( 6.117759945537829758, 54.65941425414898447, -14.99999999999999822 ) ) ;
#22455=CARTESIAN_POINT ( 'NONE',  ( 124.3771271284221314, 37.27929687716787299, 13.57481594606304753 ) ) ;
#22460=CARTESIAN_POINT ( 'NONE',  ( 70.32379096396013551, 54.47170356488336296, 14.99999999999997868 ) ) ;
#22463=EDGE_LOOP ( 'NONE', ( #12446, #2855, #25080, #14043 ) ) ;
#22466=CARTESIAN_POINT ( 'NONE',  ( 204.5988444088204687, 38.12265624999999858, 9.598844408820456309 ) ) ;
#22469=CARTESIAN_POINT ( 'NONE',  ( 78.14518615778179367, 33.26093750108393721, -5.444914386472297529 ) ) ;
#22473=CARTESIAN_POINT ( 'NONE',  ( 13.14518615778179722, 37.72578125108393010, 5.444914386472293977 ) ) ;
#22477=CARTESIAN_POINT ( 'NONE',  ( 116.4251840539369596, 33.85624999999999574, 0.000000000000000000 ) ) ;
#22479=CARTESIAN_POINT ( 'NONE',  ( 0.000000000000000000, 52.00000000000000711, 0.000000000000000000 ) ) ;
#22483=CARTESIAN_POINT ( 'NONE',  ( 139.2950502721270425, 32.91367187608393152, 9.295050272127046043 ) ) ;
#22484=CARTESIAN_POINT ( 'NONE',  ( 55.70494972787295751, 38.86679687608393863, -9.295050272127046043 ) ) ;
#22485=DIRECTION ( 'NONE',  ( 0.000000000000000000, 0.000000000000000000, -1.000000000000000000 ) ) ;
#22486=CARTESIAN_POINT ( 'NONE',  ( 13.14518615778179900, 40.20625000108393010, -5.444914386472297529 ) ) ;
#22491=CARTESIAN_POINT ( 'NONE',  ( 0.000000000000000000, 50.00000000000000000, 0.000000000000000000 ) ) ;
#22494=CARTESIAN_POINT ( 'NONE',  ( 99.99999999999995737, 85.00000000000000000, -5.000000000000018652 ) ) ;
#22501=CARTESIAN_POINT ( 'NONE',  ( 181.4251840539369596, 32.21914062500000142, -5.622872871577873077 ) ) ;
#22503=CARTESIAN_POINT ( 'NONE',  ( -8.312177448680279460E-16, 36.83281249999999574, -13.57481594606304576 ) ) ;
#22505=CARTESIAN_POINT ( 'NONE',  ( 59.55508561352770158, 40.10703125108393152, 13.14518615778179722 ) ) ;
#22510=CARTESIAN_POINT ( 'NONE',  ( 5.622872871577878406, 34.10429687499999574, 13.57481594606304576 ) ) ;
#22511=CARTESIAN_POINT ( 'NONE',  ( 135.4449143864723055, 33.36015625108393579, -13.14518615778179900 ) ) ;
#22514=CARTESIAN_POINT ( 'NONE',  ( 97.92893218813451028, 80.81250000000001421, -5.000000000000018652 ) ) ;
#22516=DIRECTION ( 'NONE',  ( -0.000000000000000000, 1.000000000000000000, -0.000000000000000000 ) ) ;
#22517=CARTESIAN_POINT ( 'NONE',  ( 103.1528011352953342, 83.06250000136560629, -3.152801135295383084 ) ) ;
#22519=CARTESIAN_POINT ( 'NONE',  ( 78.57481594606304043, 39.06523437716786873, 5.622872871577869525 ) ) ;
#22522=CARTESIAN_POINT ( 'NONE',  ( 74.59884440882045453, 40.70234374999999716, -9.598844408820458085 ) ) ;
#22523=CARTESIAN_POINT ( 'NONE',  ( 5.622872871577878406, 38.17226562716786731, 13.57481594606304576 ) ) ;
#22525=CARTESIAN_POINT ( 'NONE',  ( 59.37712712842208873, 36.38632812499999858, 13.57481594606300135 ) ) ;
#22529=CARTESIAN_POINT ( 'NONE',  ( 195.0000000000000000, 35.34453125216787583, -13.57481594606304576 ) ) ;
#22532=CARTESIAN_POINT ( 'NONE',  ( 208.5748159460630688, 38.37070312716787157, -5.622872871577873966 ) ) ;
#22533=CARTESIAN_POINT ( 'NONE',  ( -13.14518615778179544, 35.98945312608393721, 0.000000000000000000 ) ) ;
#22535=CARTESIAN_POINT ( 'NONE',  ( 70.62287287157788285, 32.51679687499999716, 13.57481594606304576 ) ) ;
#22538=CARTESIAN_POINT ( 'NONE',  ( 116.9040934463640156, 36.00000000000000000, 1.137167824541468031 ) ) ;
#22540=CARTESIAN_POINT ( 'NONE',  ( 214.9999999999999716, 55.00000000000000000, -10.00000000000000000 ) ) ;
#22547=CARTESIAN_POINT ( 'NONE',  ( -13.14518615778179189, 34.45156250108394147, 5.444914386472304635 ) ) ;
#22548=EDGE_LOOP ( 'NONE', ( #15696, #3592, #5615, #25888, #17876, #14183, #10300, #14571, #771, #4319, #23088, #11406, #23497, #20451, #15883 ) ) ;
#22554=CARTESIAN_POINT ( 'NONE',  ( 204.2950502721270425, 36.28710937608393294, -9.295050272127046043 ) ) ;
#22555=VERTEX_POINT ( 'NONE', #7967 ) ;
#22556=( BOUNDED_CURVE ( )  B_SPLINE_CURVE ( 2, ( #10003, #1203, #23135, #21272, #20721, #16287, #9871, #1755, #12411, #20857, #18578, #18983, #1616, #16712, #14277, #19128, #8011, #27834, #21131, #25546, #24989, #1339, #1477, #20996, #3884, #5611, #27693, #10274, #18712, #7875, #5469, #14420, #10133, #27281, #6026, #5891, #11996, #14561, #7738, #22995, #16427, #18845, #23276, #23410, #3611, #10421, #14138, #25260, #25124, #3465, #12131, #27412, #12270, #25409, #5751, #27554, #3749, #23551, #21841, #11115, #6437, #8573, #15251, #21555, #14827, #1896, #26104, #23969, #4448, #15106, #10698, #8288, #2172, #21418, #6161, #10562, #19686, #10834, #4028, #6569, #16980 ),
 .UNSPECIFIED., .F., .F. ) 
 B_SPLINE_CURVE_WITH_KNOTS ( ( 3, 2, 2, 2, 2, 2, 2, 2, 2, 2, 2, 2, 2, 2, 2, 2, 2, 2, 2, 2, 2, 2, 2, 2, 2, 2, 2, 2, 2, 2, 2, 2, 2, 2, 2, 2, 2, 2, 2, 2, 3 ),
 ( 0.000000000000000000, 0.02500000000000000139, 0.05000000000000000278, 0.07499999999999999722, 0.1000000000000000056, 0.1250000000000000000, 0.1499999999999999944, 0.1749999999999999889, 0.2000000000000000111, 0.2250000000000000056, 0.2500000000000000000, 0.2750000000000000222, 0.2999999999999999889, 0.3250000000000000111, 0.3499999999999999778, 0.3750000000000000000, 0.4000000000000000222, 0.4249999999999999889, 0.4500000000000000111, 0.4749999999999999778, 0.5000000000000000000, 0.5250000000000000222, 0.5500000000000000444, 0.5749999999999999556, 0.5999999999999999778, 0.6250000000000000000, 0.6500000000000000222, 0.6750000000000000444, 0.6999999999999999556, 0.7249999999999999778, 0.7500000000000000000, 0.7750000000000000222, 0.8000000000000000444, 0.8249999999999999556, 0.8499999999999999778, 0.8750000000000000000, 0.9000000000000000222, 0.9250000000000000444, 0.9499999999999999556, 0.9749999999999999778, 1.000000000000000000 ),
 .UNSPECIFIED. ) 
 CURVE ( )  GEOMETRIC_REPRESENTATION_ITEM ( )  RATIONAL_B_SPLINE_CURVE ( ( 1.000000000000000000, 0.9238795325112867385, 1.000000000000000000, 0.9238795325112867385, 1.000000000000000000, 0.9238795325112867385, 1.000000000000000000, 0.9238795325112867385, 1.000000000000000000, 0.9238795325112867385, 1.000000000000000000, 0.9238795325112867385, 1.000000000000000000, 0.9238795325112867385, 1.000000000000000000, 0.9238795325112867385, 1.000000000000000000, 0.9238795325112867385, 1.000000000000000000, 0.9238795325112867385, 1.000000000000000000, 0.9238795325112867385, 1.000000000000000000, 0.9238795325112867385, 1.000000000000000000, 0.9238795325112867385, 1.000000000000000000, 0.9238795325112867385, 1.000000000000000000, 0.9238795325112867385, 1.000000000000000000, 0.9238795325112867385, 1.000000000000000000, 0.9238795325112867385, 1.000000000000000000, 0.9238795325112867385, 1.000000000000000000, 0.9238795325112867385, 1.000000000000000000, 0.9238795325112867385, 1.000000000000000000, 0.9238795325112867385, 1.000000000000000000, 0.9238795325112867385, 1.000000000000000000, 0.9238795325112867385, 1.000000000000000000, 0.9238795325112867385, 1.000000000000000000, 0.9238795325112867385, 1.000000000000000000, 0.9238795325112867385, 1.000000000000000000, 0.9238795325112867385, 1.000000000000000000, 0.9238795325112867385, 1.000000000000000000, 0.9238795325112867385, 1.000000000000000000, 0.9238795325112867385, 1.000000000000000000, 0.9238795325112867385, 1.000000000000000000, 0.9238795325112867385, 1.000000000000000000, 0.9238795325112867385, 1.000000000000000000, 0.9238795325112867385, 1.000000000000000000, 0.9238795325112867385, 1.000000000000000000, 0.9238795325112867385, 1.000000000000000000, 0.9238795325112867385, 1.000000000000000000, 0.9238795325112867385, 1.000000000000000000, 0.9238795325112867385, 1.000000000000000000, 0.9238795325112867385, 1.000000000000000000 ) ) 
 REPRESENTATION_ITEM ( '' )  );
#22557=CARTESIAN_POINT ( 'NONE',  ( 188.8801563723155823, 51.28708186915214640, -15.00000000000279243 ) ) ;
#22561=VECTOR ( 'NONE', #18943, 1000.000000000000000 ) ;
#22563=LINE ( 'NONE', #11700, #10287 ) ;
#22565=CARTESIAN_POINT ( 'NONE',  ( 124.5550856135277087, 38.32109375108394289, 13.14518615778179722 ) ) ;
#22566=CARTESIAN_POINT ( 'NONE',  ( -5.444914386472297529, 36.63437500108393863, -13.14518615778179722 ) ) ;
#22567=CARTESIAN_POINT ( 'NONE',  ( 13.14518615778179900, 36.13828125108393863, 5.444914386472293977 ) ) ;
#22571=CARTESIAN_POINT ( 'NONE',  ( 66.01413082606791249, 51.45790058219658647, -14.99999999999999645 ) ) ;
#22573=CARTESIAN_POINT ( 'NONE',  ( 78.01985494039040248, 36.00000000000002132, 3.369129453356682014 ) ) ;
#22576=CARTESIAN_POINT ( 'NONE',  ( 70.44491438647229131, 38.71796875108393721, -13.14518615778179722 ) ) ;
#22585=CARTESIAN_POINT ( 'NONE',  ( 185.7049497278729575, 36.68398437608393436, -9.295050272127046043 ) ) ;
#22590=AXIS2_PLACEMENT_3D ( 'NONE', #19865, #6605, #8470 ) ;
#22591=ORIENTED_EDGE ( 'NONE', *, *, #8674, .F. ) ;
#22592=CARTESIAN_POINT ( 'NONE',  ( 135.4449143864723055, 33.06250000108393294, 13.14518615778179189 ) ) ;
#22593=CARTESIAN_POINT ( 'NONE',  ( 70.44491438647229131, 40.20625000108394431, 13.14518615778179189 ) ) ;
#22595=CARTESIAN_POINT ( 'NONE',  ( 204.2950502721270425, 35.49335937608393721, 9.295050272127046043 ) ) ;
#22596=ORIENTED_EDGE ( 'NONE', *, *, #19255, .T. ) ;
#22599=CARTESIAN_POINT ( 'NONE',  ( 195.0000000000000000, 36.00000000000000000, -11.57481594606306707 ) ) ;
#22600=CARTESIAN_POINT ( 'NONE',  ( 139.5988444088204403, 36.83281250216787583, -9.598844408820458085 ) ) ;
#22603=AXIS2_PLACEMENT_3D ( 'NONE', #22289, #26564, #24562 ) ;
#22604=DIRECTION ( 'NONE',  ( 1.000000000000000000, 0.000000000000000000, -2.385244779468110248E-16 ) ) ;
#22609=ORIENTED_EDGE ( 'NONE', *, *, #8960, .T. ) ;
#22612=CARTESIAN_POINT ( 'NONE',  ( 130.0000000000000000, 38.51953125216787299, -13.57481594606304576 ) ) ;
#22613=CARTESIAN_POINT ( 'NONE',  ( -4.780039198851662618, 35.99999999999998579, 12.25280873422828520 ) ) ;
#22614=CARTESIAN_POINT ( 'NONE',  ( 51.85481384221820633, 33.65781250108393152, 5.444914386472304635 ) ) ;
#22617=CARTESIAN_POINT ( 'NONE',  ( 5.908507747193088022, 36.04503594658365984, 12.68159279706100939 ) ) ;
#22619=CARTESIAN_POINT ( 'NONE',  ( -8.268597328389915901, 50.00000000054339466, 10.78867689284126463 ) ) ;
#22620=CARTESIAN_POINT ( 'NONE',  ( 51.42518405393695957, 40.99999999999999289, 0.000000000000000000 ) ) ;
#22621=CARTESIAN_POINT ( 'NONE',  ( 116.4251840539369454, 33.01289062500000426, -5.622872871577873077 ) ) ;
#22627=VECTOR ( 'NONE', #17009, 1000.000000000000000 ) ;
#22629=CARTESIAN_POINT ( 'NONE',  ( 143.1451861577818079, 32.16953125108393152, 5.444914386472293977 ) ) ;
#22630=CARTESIAN_POINT ( 'NONE',  ( 70.44491438647230552, 39.51171875108392584, -13.14518615778179900 ) ) ;
#22631=EDGE_CURVE ( 'NONE', #4145, #23060, #9962, .T. ) ;
#22632=CARTESIAN_POINT ( 'NONE',  ( 104.9999999999999716, 80.50000000000000000, -1.449011120738813565E-14 ) ) ;
#22633=CARTESIAN_POINT ( 'NONE',  ( 13.14518615778179544, 39.36289062608393152, -1.609821015232357215E-15 ) ) ;
#22635=LINE ( 'NONE', #5385, #14839 ) ;
#22638=CARTESIAN_POINT ( 'NONE',  ( 185.7049497278729575, 31.92148437608393508, 9.295050272127047819 ) ) ;
#22642=CARTESIAN_POINT ( 'NONE',  ( 128.7288612287584044, 36.00000000000000000, -13.43002483374371714 ) ) ;
#22643=CARTESIAN_POINT ( 'NONE',  ( 130.0000000000000000, 36.53515625216787299, 13.57481594606304576 ) ) ;
#22644=CARTESIAN_POINT ( 'NONE',  ( 195.0000000000000000, -7.395377635281828788, 13.57481594606302266 ) ) ;
#22653=CARTESIAN_POINT ( 'NONE',  ( 65.00000000000000000, 33.60820312608392868, 13.14518615778179544 ) ) ;
#22657=CARTESIAN_POINT ( 'NONE',  ( -8.312177448680279460E-16, 37.62656249999999858, -13.57481594606304576 ) ) ;
#22658=CARTESIAN_POINT ( 'NONE',  ( -8.312177448680279460E-16, 32.07031249999999289, -13.57481594606304576 ) ) ;
#22659=CARTESIAN_POINT ( 'NONE',  ( 120.7049497278729575, 34.30273437608393294, -9.295050272127046043 ) ) ;
#22660=ORIENTED_EDGE ( 'NONE', *, *, #15915, .F. ) ;
#22663=CARTESIAN_POINT ( 'NONE',  ( 104.9999999999999574, 79.68750000273119838, -2.071067811865491937 ) ) ;
#22665=CARTESIAN_POINT ( 'NONE',  ( 59.37712712842213136, 38.86679687716788578, 13.57481594606304753 ) ) ;
#22667=CARTESIAN_POINT ( 'NONE',  ( 195.0000000000000000, 40.15664062608393436, 13.14518615778179544 ) ) ;
#22668=CARTESIAN_POINT ( 'NONE',  ( 9.598844408820459861, 37.42812500216787441, 9.598844408820456309 ) ) ;
#22669=ORIENTED_EDGE ( 'NONE', *, *, #16960, .T. ) ;
#22671=CARTESIAN_POINT ( 'NONE',  ( 185.9219080773009125, 36.00000000000000711, -9.794392408848729303 ) ) ;
#22673=EDGE_LOOP ( 'NONE', ( #9318, #21959, #14398 ) ) ;
#22675=CARTESIAN_POINT ( 'NONE',  ( 200.4449143864723055, 39.51171875108392584, -13.14518615778179900 ) ) ;
#22679=CARTESIAN_POINT ( 'NONE',  ( -8.049105076161786076E-16, 32.61601562608393579, -13.14518615778179544 ) ) ;
#22681=CARTESIAN_POINT ( 'NONE',  ( 116.8548138422182063, 32.56640625108394005, -5.444914386472297529 ) ) ;
#22682=CARTESIAN_POINT ( 'NONE',  ( 55.40115559117954547, 32.16953124999999147, -9.598844408820458085 ) ) ;
#22686=CARTESIAN_POINT ( 'NONE',  ( -13.57481594606304576, 37.92421875216787441, 0.000000000000000000 ) ) ;
#22689=FACE_OUTER_BOUND ( 'NONE', #12243, .T. ) ;
#22690=CARTESIAN_POINT ( 'NONE',  ( 214.9999999999999716, 75.00000000000000000, -9.999999999999998224 ) ) ;
#22692=CARTESIAN_POINT ( 'NONE',  ( 9.295050272127047819, 34.69960937608393436, 9.295050272127046043 ) ) ;
#22693=VECTOR ( 'NONE', #9803, 1000.000000000000000 ) ;
#22699=CARTESIAN_POINT ( 'NONE',  ( 185.7049497278729575, 35.09648437608392868, 9.295050272127047819 ) ) ;
#22701=CARTESIAN_POINT ( 'NONE',  ( 191.9553905430759926, 53.89089363584393766, -14.99999999999999645 ) ) ;
#22703=ORIENTED_EDGE ( 'NONE', *, *, #2053, .F. ) ;
#22706=CARTESIAN_POINT ( 'NONE',  ( 12.07727640983618400, 35.99999999999999289, -6.197985357348142266 ) ) ;
#22708=CARTESIAN_POINT ( 'NONE',  ( 116.8548138422182205, 37.37851562608393863, 0.000000000000000000 ) ) ;
#22709=CARTESIAN_POINT ( 'NONE',  ( -13.14518615778179722, 36.73359375108393010, -5.444914386472297529 ) ) ;
#22710=CARTESIAN_POINT ( 'NONE',  ( 5.444914386472302859, 36.83281250108392868, 13.14518615778179189 ) ) ;
#22712=CARTESIAN_POINT ( 'NONE',  ( 63.49450781844505087, 53.60078691996341860, -14.99999999999999822 ) ) ;
#22714=ORIENTED_EDGE ( 'NONE', *, *, #23222, .T. ) ;
#22716=CARTESIAN_POINT ( 'NONE',  ( 74.59884440882045453, 38.12265624999999858, 9.598844408820456309 ) ) ;
#22720=CARTESIAN_POINT ( 'NONE',  ( 55.70494972787295751, 37.47773437608393010, 9.295050272127047819 ) ) ;
#22721=DIRECTION ( 'NONE',  ( -0.000000000000000000, -0.000000000000000000, -1.000000000000000000 ) ) ;
#22723=CARTESIAN_POINT ( 'NONE',  ( 204.2950502721270425, 36.88242187608393152, 9.295050272127046043 ) ) ;
#22727=CARTESIAN_POINT ( 'NONE',  ( 189.5550856135277229, 38.22187500108393721, -13.14518615778179722 ) ) ;
#22733=DIRECTION ( 'NONE',  ( 0.000000000000000000, 0.000000000000000000, -1.000000000000000000 ) ) ;
#22734=CARTESIAN_POINT ( 'NONE',  ( 51.85481384221820633, 39.95820312608393010, 0.000000000000000000 ) ) ;
#22735=CARTESIAN_POINT ( 'NONE',  ( 185.8198241863519797, 55.00000000000000000, 9.999999999999953815 ) ) ;
#22736=CARTESIAN_POINT ( 'NONE',  ( 208.1451861577818079, 34.79882812608394005, -1.609821015232357215E-15 ) ) ;
#22737=EDGE_CURVE ( 'NONE', #18276, #12549, #4396, .T. ) ;
#22739=CARTESIAN_POINT ( 'NONE',  ( 65.00000000000000000, -7.395377635281828788, -11.57481594606305109 ) ) ;
#22740=CARTESIAN_POINT ( 'NONE',  ( 7.115490391850728180, 49.99999999945644902, -11.58166858714323055 ) ) ;
#22742=CARTESIAN_POINT ( 'NONE',  ( 124.3771271284221314, 38.86679687716788578, 13.57481594606304753 ) ) ;
#22743=CARTESIAN_POINT ( 'NONE',  ( 130.0000000000000000, 52.00000000000000711, -1.503427012513233026E-14 ) ) ;
#22745=CARTESIAN_POINT ( 'NONE',  ( 73.20144618763828248, 50.69246985422719121, 14.99999999999789146 ) ) ;
#22746=ORIENTED_EDGE ( 'NONE', *, *, #4769, .F. ) ;
#22751=ORIENTED_EDGE ( 'NONE', *, *, #10708, .T. ) ;
#22756=DIRECTION ( 'NONE',  ( 0.000000000000000000, 0.000000000000000000, 1.000000000000000000 ) ) ;
#22758=CARTESIAN_POINT ( 'NONE',  ( -13.57481594606304753, 40.25585937716787299, -5.622872871577872189 ) ) ;
#22760=CARTESIAN_POINT ( 'NONE',  ( -13.57481594606304576, 39.51171875216787299, 0.000000000000000000 ) ) ;
#22764=CARTESIAN_POINT ( 'NONE',  ( 124.3771271284221314, 32.91367187499999858, -13.57481594606304753 ) ) ;
#22766=ORIENTED_EDGE ( 'NONE', *, *, #9429, .F. ) ;
#22770=CARTESIAN_POINT ( 'NONE',  ( 135.4449143864723055, 32.36796875108393579, -13.14518615778179900 ) ) ;
#22771=CARTESIAN_POINT ( 'NONE',  ( 51.85481384221820633, 39.01562500108393294, 5.444914386472304635 ) ) ;
#22774=CARTESIAN_POINT ( 'NONE',  ( 13.14518615778179900, 38.51953125108393294, 5.444914386472293977 ) ) ;
#22776=CARTESIAN_POINT ( 'NONE',  ( 182.1602487631418228, 35.99999999999998579, 2.850296047819894873 ) ) ;
#22777=CARTESIAN_POINT ( 'NONE',  ( 65.00000000000000000, 50.00000000000000000, -13.57481594606305109 ) ) ;
#22779=CARTESIAN_POINT ( 'NONE',  ( 181.8548138422182205, 31.82226562608393650, 0.000000000000000000 ) ) ;
#22780=FACE_OUTER_BOUND ( 'NONE', #15808, .T. ) ;
#22790=CARTESIAN_POINT ( 'NONE',  ( 200.6228728715778686, 32.81445312499999289, -13.57481594606304753 ) ) ;
#22794=CARTESIAN_POINT ( 'NONE',  ( 98.15313185440925281, 83.62500000136560629, 4.458734124999987891 ) ) ;
#22795=CARTESIAN_POINT ( 'NONE',  ( 51.85481384221820633, 31.82226562608393650, 0.000000000000000000 ) ) ;
#22798=CARTESIAN_POINT ( 'NONE',  ( 116.4251840539369738, 37.97382812716787726, 5.622872871577880183 ) ) ;
#22799=DIRECTION ( 'NONE',  ( 0.000000000000000000, 0.000000000000000000, -1.000000000000000000 ) ) ;
#22801=CARTESIAN_POINT ( 'NONE',  ( 116.8548138422182063, 34.35234375108393579, -5.444914386472297529 ) ) ;
#22802=ORIENTED_EDGE ( 'NONE', *, *, #9429, .T. ) ;
#22803=DIRECTION ( 'NONE',  ( -1.156482317317871478E-16, -0.000000000000000000, -1.000000000000000000 ) ) ;
#22805=CARTESIAN_POINT ( 'NONE',  ( 208.5748159460630688, 36.73359375216787015, -1.662435489736055892E-15 ) ) ;
#22806=CARTESIAN_POINT ( 'NONE',  ( 104.4587341249999781, 82.00000000136560629, -1.846868145590750299 ) ) ;
#22810=CARTESIAN_POINT ( 'NONE',  ( 204.2950502721270425, 32.31835937608393294, -9.295050272127046043 ) ) ;
#22811=CARTESIAN_POINT ( 'NONE',  ( 13.57481594606304753, 37.57695312716787583, -5.622872871577873077 ) ) ;
#22812=ORIENTED_EDGE ( 'NONE', *, *, #19754, .T. ) ;
#22814=ORIENTED_EDGE ( 'NONE', *, *, #13642, .F. ) ;
#22816=CARTESIAN_POINT ( 'NONE',  ( 195.0000000000000000, 31.77265625216787370, 13.57481594606304576 ) ) ;
#22819=AXIS2_PLACEMENT_3D ( 'NONE', #22072, #20073, #17786 ) ;
#22820=CARTESIAN_POINT ( 'NONE',  ( 120.7049497278729575, 39.85898437608393152, 9.295050272127047819 ) ) ;
#22821=CARTESIAN_POINT ( 'NONE',  ( -5.444914386472299306, 32.96328125108393436, 13.14518615778179722 ) ) ;
#22822=B_SPLINE_CURVE_WITH_KNOTS ( 'NONE', 3,
 ( #16371, #8229, #5965, #27364, #6102, #3553, #21074, #1835, #14769, #3825, #21212, #1280, #27499, #1697, #20800, #7954, #5832, #22943 ),
 .UNSPECIFIED., .F., .F.,
 ( 4, 2, 2, 2, 2, 2, 2, 2, 4 ),
 ( 0.000000000000000000, 0.004618502246277159280, 0.006927753369415741089, 0.009237004492554323765, 0.01039163005412361250, 0.01154625561569290471, 0.01385550673883148044, 0.01616475786197005618, 0.01847400898510863018 ),
 .UNSPECIFIED. ) ;
#22823=CARTESIAN_POINT ( 'NONE',  ( 130.0000000000000000, 32.81445312608393294, 13.14518615778179544 ) ) ;
#22824=CARTESIAN_POINT ( 'NONE',  ( 51.42518405393695957, 33.06249999999999289, 0.000000000000000000 ) ) ;
#22826=EDGE_CURVE ( 'NONE', #18276, #4141, #16562, .T. ) ;
#22835=CARTESIAN_POINT ( 'NONE',  ( 195.0000000000000000, 40.00781250000000000, -13.57481594606304576 ) ) ;
#22837=CARTESIAN_POINT ( 'NONE',  ( 9.295050272127047819, 33.11210937608393579, 9.295050272127046043 ) ) ;
#22841=CARTESIAN_POINT ( 'NONE',  ( 195.0000000000000000, 33.21132812608393436, -13.14518615778179544 ) ) ;
#22842=ORIENTED_EDGE ( 'NONE', *, *, #5465, .F. ) ;
#22843=CARTESIAN_POINT ( 'NONE',  ( 201.1177599455311338, 54.65941425414898447, -14.99999999999999645 ) ) ;
#22848=DIRECTION ( 'NONE',  ( 0.000000000000000000, 1.000000000000000000, 0.000000000000000000 ) ) ;
#22850=CARTESIAN_POINT ( 'NONE',  ( 135.4449143864723055, 37.13046875108393152, -13.14518615778179900 ) ) ;
#22851=CARTESIAN_POINT ( 'NONE',  ( 9.295050272127047819, 36.28710937608393294, 9.295050272127046043 ) ) ;
#22852=CARTESIAN_POINT ( 'NONE',  ( -5.444914386472299306, 31.97109375108393436, 13.14518615778179722 ) ) ;
#22859=FACE_OUTER_BOUND ( 'NONE', #21845, .T. ) ;
#22860=CARTESIAN_POINT ( 'NONE',  ( 68.79745186895802078, 54.08938259242986391, 14.99999999999998224 ) ) ;
#22862=ORIENTED_EDGE ( 'NONE', *, *, #26373, .T. ) ;
#22868=ADVANCED_FACE ( 'NONE', ( #8526 ), #6800, .T. ) ;
#22874=CARTESIAN_POINT ( 'NONE',  ( 51.85481384221819923, 31.77265625108393365, -5.444914386472297529 ) ) ;
#22875=DIRECTION ( 'NONE',  ( 0.000000000000000000, 0.000000000000000000, -1.000000000000000000 ) ) ;
#22876=CARTESIAN_POINT ( 'NONE',  ( 208.1451861577817795, 33.16171875108393863, 5.444914386472293977 ) ) ;
#22877=VERTEX_POINT ( 'NONE', #17211 ) ;
#22880=VECTOR ( 'NONE', #21646, 1000.000000000000000 ) ;
#22881=CARTESIAN_POINT ( 'NONE',  ( 135.6228728715778686, 36.88242187716787157, -13.57481594606304753 ) ) ;
#22883=DIRECTION ( 'NONE',  ( -0.000000000000000000, 1.000000000000000000, -0.000000000000000000 ) ) ;
#22885=CARTESIAN_POINT ( 'NONE',  ( 208.1451861577817795, 38.02343750108395426, -5.444914386472297529 ) ) ;
#22889=CARTESIAN_POINT ( 'NONE',  ( -8.669112105337029917, 36.00000000000002842, -10.16963847934323262 ) ) ;
#22890=CARTESIAN_POINT ( 'NONE',  ( 131.8921833570923638, 53.66387243068089674, 14.99999999999996447 ) ) ;
#22891=CARTESIAN_POINT ( 'NONE',  ( -12.73839015785548945, 36.00000000000000000, 3.273369733618486155 ) ) ;
#22892=CARTESIAN_POINT ( 'NONE',  ( 51.85481384221819923, 31.97109375108393436, -5.444914386472297529 ) ) ;
#22896=CARTESIAN_POINT ( 'NONE',  ( 1.137167824540872951, 35.99999999999998579, 13.09590655363602707 ) ) ;
#22897=CARTESIAN_POINT ( 'NONE',  ( 96.46446609406721961, 83.12500000000000000, 3.535533905932727539 ) ) ;
#22898=CARTESIAN_POINT ( 'NONE',  ( 120.4011555911795455, 34.74921874999999716, 9.598844408820459861 ) ) ;
#22902=LINE ( 'NONE', #3365, #16765 ) ;
#22906=CARTESIAN_POINT ( 'NONE',  ( 139.2950502721270425, 39.66054687608393436, -9.295050272127046043 ) ) ;
#22907=EDGE_CURVE ( 'NONE', #8135, #778, #17452, .T. ) ;
#22908=CARTESIAN_POINT ( 'NONE',  ( 59.37712712842213136, 31.72304687716787441, 13.57481594606304753 ) ) ;
#22909=EDGE_CURVE ( 'NONE', #17753, #25242, #26099, .T. ) ;
#22911=CARTESIAN_POINT ( 'NONE',  ( -9.295050272127044266, 39.85898437608393152, 9.295050272127047819 ) ) ;
#22913=CARTESIAN_POINT ( 'NONE',  ( 0.000000000000000000, -7.395377635281828788, 13.57481594606304398 ) ) ;
#22917=CARTESIAN_POINT ( 'NONE',  ( 13.14518615778179544, 40.15664062608393436, -1.609821015232357215E-15 ) ) ;
#22920=VECTOR ( 'NONE', #10575, 1000.000000000000000 ) ;
#22921=ADVANCED_FACE ( 'NONE', ( #13768 ), #9088, .T. ) ;
#22923=CARTESIAN_POINT ( 'NONE',  ( 189.3771271284221598, 39.26367187500000000, -13.57481594606310260 ) ) ;
#22924=CARTESIAN_POINT ( 'NONE',  ( 116.4251840539369596, 40.30546875216787583, 0.000000000000000000 ) ) ;
#22933=CARTESIAN_POINT ( 'NONE',  ( 95.54126587499995082, 83.37500000136563472, -1.846868145590750077 ) ) ;
#22934=CARTESIAN_POINT ( 'NONE',  ( 78.14518615778179367, 40.35507812608393863, -1.609821015232357215E-15 ) ) ;
#22937=CARTESIAN_POINT ( 'NONE',  ( 130.0000000000000000, 39.61093749999999147, 13.57481594606304576 ) ) ;
#22938=CARTESIAN_POINT ( 'NONE',  ( -13.57481594606304576, 32.31835937499999289, 5.622872871577880183 ) ) ;
#22940=CARTESIAN_POINT ( 'NONE',  ( 116.8548138422182205, 35.19570312608393436, 0.000000000000000000 ) ) ;
#22941=ADVANCED_FACE ( 'NONE', ( #26487 ), #4679, .T. ) ;
#22943=CARTESIAN_POINT ( 'NONE',  ( -9.180175813647991845, 55.00000000000000000, -14.99999999999999822 ) ) ;
#22944=( BOUNDED_CURVE ( )  B_SPLINE_CURVE ( 2, ( #20126, #23977, #17269 ),
 .UNSPECIFIED., .F., .T. ) 
 B_SPLINE_CURVE_WITH_KNOTS ( ( 3, 3 ),
 ( 0.8250000005912452306, 0.8500000000000007550 ),
 .UNSPECIFIED. ) 
 CURVE ( )  GEOMETRIC_REPRESENTATION_ITEM ( )  RATIONAL_B_SPLINE_CURVE ( ( 1.000000000000000000, 0.9238795325112844070, 1.000000000000002442 ) ) 
 REPRESENTATION_ITEM ( '' )  );
#22945=CARTESIAN_POINT ( 'NONE',  ( 208.5748159460630688, 36.78320312716788010, -5.622872871577873966 ) ) ;
#22946=CARTESIAN_POINT ( 'NONE',  ( 104.4587341249999639, 81.93750000136559208, -1.442382525525748735E-14 ) ) ;
#22947=CARTESIAN_POINT ( 'NONE',  ( 139.2950502721270425, 38.66835937608393436, -9.295050272127046043 ) ) ;
#22948=CARTESIAN_POINT ( 'NONE',  ( 130.0000000000000000, 38.42031249999999432, -13.57481594606304576 ) ) ;
#22951=CARTESIAN_POINT ( 'NONE',  ( 189.5550856135277229, 32.46718750108393436, -13.14518615778179900 ) ) ;
#22952=CARTESIAN_POINT ( 'NONE',  ( -9.598844408820454532, 39.61093750216787868, 9.598844408820459861 ) ) ;
#22953=ORIENTED_EDGE ( 'NONE', *, *, #22737, .T. ) ;
#22958=CARTESIAN_POINT ( 'NONE',  ( 181.4251840539369596, 32.36796875216787583, 0.000000000000000000 ) ) ;
#22961=CARTESIAN_POINT ( 'NONE',  ( 130.0000000000000000, 40.35507812608393152, -13.14518615778179544 ) ) ;
#22962=CARTESIAN_POINT ( 'NONE',  ( 5.444914386472302859, 33.06250000108393294, 13.14518615778179189 ) ) ;
#22966=CARTESIAN_POINT ( 'NONE',  ( 185.4011555911795597, 39.51171874999999289, 9.598844408820459861 ) ) ;
#22968=CARTESIAN_POINT ( 'NONE',  ( 121.8746960822088141, 36.00000000000000000, 10.34220695173579507 ) ) ;
#22975=CARTESIAN_POINT ( 'NONE',  ( -5.444914386472297529, 31.87187500108393223, -13.14518615778179900 ) ) ;
#22977=CARTESIAN_POINT ( 'NONE',  ( 98.15313185440925281, 84.50000000136562051, -4.458734125000016313 ) ) ;
#22978=( BOUNDED_CURVE ( )  B_SPLINE_CURVE ( 2, ( #27180, #27036, #814, #18329, #24604 ),
 .UNSPECIFIED., .F., .F. ) 
 B_SPLINE_CURVE_WITH_KNOTS ( ( 3, 2, 3 ),
 ( 0.000000000000000000, 0.01041666666666679446, 0.02083333333333358892 ),
 .UNSPECIFIED. ) 
 CURVE ( )  GEOMETRIC_REPRESENTATION_ITEM ( )  RATIONAL_B_SPLINE_CURVE ( ( 1.000000000000000000, 0.9238795325112867385, 1.000000000000000000, 0.9238795325112848511, 1.000000000000001776 ) ) 
 REPRESENTATION_ITEM ( '' )  );
#22980=CARTESIAN_POINT ( 'NONE',  ( 204.2950502721270425, 33.90585937608393152, -9.295050272127046043 ) ) ;
#22982=CARTESIAN_POINT ( 'NONE',  ( 187.3780364657951338, 54.91641323977498246, -15.00000000000000000 ) ) ;
#22988=CARTESIAN_POINT ( 'NONE',  ( -5.444914386472297529, 37.42812500108394147, -13.14518615778179722 ) ) ;
#22989=CARTESIAN_POINT ( 'NONE',  ( -5.444914386472299306, 40.10703125108393152, 13.14518615778179722 ) ) ;
#22991=CARTESIAN_POINT ( 'NONE',  ( 94.99999999999995737, 84.56250000136560629, -1.387778780781445676E-14 ) ) ;
#22995=CARTESIAN_POINT ( 'NONE',  ( 104.4587341249999781, 82.25000000136559208, -1.846868145590750521 ) ) ;
#22997=CARTESIAN_POINT ( 'NONE',  ( 2.493653234604083739E-15, 38.91640625216786731, 13.57481594606304576 ) ) ;
#22998=CARTESIAN_POINT ( 'NONE',  ( 57.37605803807456084, 55.00000000000000000, 14.99999999999998579 ) ) ;
#23005=CIRCLE ( 'NONE', #10687, 13.57481594606304398 ) ;
#23008=ORIENTED_EDGE ( 'NONE', *, *, #5320, .F. ) ;
#23009=CARTESIAN_POINT ( 'NONE',  ( 51.85481384221820633, 38.37070312608393152, 0.000000000000000000 ) ) ;
#23012=( BOUNDED_CURVE ( )  B_SPLINE_CURVE ( 2, ( #26345, #4536, #2824, #22351, #26489, #6946, #24202, #20356, #19779 ),
 .UNSPECIFIED., .F., .T. ) 
 B_SPLINE_CURVE_WITH_KNOTS ( ( 3, 2, 2, 2, 3 ),
 ( 0.1875000000000001388, 0.1979166666666667407, 0.2083333333333333703, 0.2187499999999999722, 0.2291666666666665741 ),
 .UNSPECIFIED. ) 
 CURVE ( )  GEOMETRIC_REPRESENTATION_ITEM ( )  RATIONAL_B_SPLINE_CURVE ( ( 0.9999999999999990008, 0.9238795325112877377, 1.000000000000000000, 0.9238795325112867385, 1.000000000000000000, 0.9238795325112867385, 1.000000000000000000, 0.9238795325112872936, 0.9999999999999994449 ) ) 
 REPRESENTATION_ITEM ( '' )  );
#23015=CARTESIAN_POINT ( 'NONE',  ( -1.892183357088964346, 53.66387243068090385, -15.00000000000000000 ) ) ;
#23016=AXIS2_PLACEMENT_3D ( 'NONE', #7276, #9139, #17832 ) ;
#23017=CARTESIAN_POINT ( 'NONE',  ( 188.8834397602831814, 54.66944451632673463, 14.99999999999994849 ) ) ;
#23018=CARTESIAN_POINT ( 'NONE',  ( 135.6228728715778686, 38.46992187716787015, -13.57481594606304753 ) ) ;
#23019=LINE ( 'NONE', #10027, #9214 ) ;
#23021=CARTESIAN_POINT ( 'NONE',  ( 189.5550856135277229, 39.01562500108394005, -13.14518615778179900 ) ) ;
#23022=EDGE_LOOP ( 'NONE', ( #14585, #13448, #2771, #15530 ) ) ;
#23024=VECTOR ( 'NONE', #8461, 1000.000000000000000 ) ;
#23025=ORIENTED_EDGE ( 'NONE', *, *, #9653, .F. ) ;
#23028=CARTESIAN_POINT ( 'NONE',  ( 13.57481594606304576, 38.22187499999999716, -1.662435489736055892E-15 ) ) ;
#23031=SURFACE_STYLE_FILL_AREA ( #25026 ) ;
#23033=CARTESIAN_POINT ( 'NONE',  ( -8.312177448680279460E-16, 40.80156249999999574, -13.57481594606304576 ) ) ;
#23034=VECTOR ( 'NONE', #8580, 1000.000000000000000 ) ;
#23035=CARTESIAN_POINT ( 'NONE',  ( 12.00957333851107300, 36.00000000000000711, 5.901833544882737925 ) ) ;
#23036=CARTESIAN_POINT ( 'NONE',  ( 8.395938741298724750, 54.99999999495823744, 14.99999999999999289 ) ) ;
#23037=CARTESIAN_POINT ( 'NONE',  ( 124.3771271284221314, 33.21132812499999432, 13.57481594606304753 ) ) ;
#23038=ORIENTED_EDGE ( 'NONE', *, *, #27785, .T. ) ;
#23044=CARTESIAN_POINT ( 'NONE',  ( 116.8548138422182205, 38.37070312608393152, 0.000000000000000000 ) ) ;
#23045=CARTESIAN_POINT ( 'NONE',  ( 59.55508561352770158, 37.22968750108393721, -13.14518615778179900 ) ) ;
#23047=CARTESIAN_POINT ( 'NONE',  ( -13.14518615778179544, 38.17226562608393436, 0.000000000000000000 ) ) ;
#23048=( BOUNDED_SURFACE ( )  B_SPLINE_SURFACE ( 1, 2, ( 
 ( #16923, #7825, #25623, #10357, #14503, #6105, #23492, #1424, #14637, #3972, #5698, #23355, #12632, #21358, #18929, #25352, #3408, #1839, #1283, #21077, #10502, #19209, #3828, #27911, #17057, #16656, #5563, #27637, #3556, #9949, #3696, #14365, #23220, #12079, #12359, #14226, #18663, #23081, #22947, #16518, #10083, #12213, #18795, #1566, #8097, #27502, #7957, #16791, #4671, #8655, #15477, #23906, #26182, #19347, #12775, #110, #26042, #2398, #8792, #11056, #6513, #397, #6243, #26331, #8517, #8935, #4386, #21778, #19765, #6648, #17625, #14912, #4525, #249, #21491, #24192, #6792, #4108, #17483, #13333, #15334, #9079, #24050, #17346, #10640, #1972, #28050, #15189, #22059, #13043, #13185, #17202, #25761, #19489, #25907, #6377, #2257, #10919, #2533, #19629, #15050, #21923, #11197, #23768, #19914, #23632, #4244, #12904, #21634, #2110, #10777, #28187, #2677, #7498, #26764, #20489, #2948, #20344, #9358, #13758, #14049, #18344, #970, #11619, #1112, #15628, #16193, #830, #17913, #22342, #9497, #16045, #11338, #7071, #13473, #11765, #3098, #7207, #15901, #4958, #17774, #538, #9221, #20198, #9640, #5380, #18051, #5096, #20628, #26478, #24618, #2812, #18197, #26624, #22483, #26908, #15766, #7354, #6934, #24755, #11481, #5237, #24329, #13902, #22198, #22770, #4813, #27049, #13620, #22629, #24900, #24473, #3236, #11903, #20059, #683, #1388, #7647, #3792, #25039, #25310, #25586, #12451 ),
 ( #7788, #14188, #7921, #1249, #18760, #16339, #10049, #12592, #5521, #18626, #27737, #9779, #12040, #14601, #3933, #23183, #8197, #16617, #5659, #14735, #25453, #27329, #22906, #3369, #23319, #21316, #5799, #16752, #14465, #27464, #16475, #3659, #10317, #21177, #25170, #20906, #1658, #6069, #12320, #19025, #21041, #16887, #1526, #14323, #18887, #10178, #23455, #27596, #23044, #18487, #3517, #27196, #20764, #9911, #12176, #8058, #5933, #13290, #8478, #13004, #2361, #10464, #6614, #8901, #10606, #28151, #21597, #23871, #19313, #4632, #19172, #6757, #17589, #26295, #23735, #10742, #8618, #23591, #27874, #19729, #17448, #28014, #15440, #21744, #11016, #24155, #1799, #15298, #24014, #12735, #19452, #4492, #4073, #17306, #26006, #6206, #13149, #214, #21459, #26147, #21887, #1937, #8336, #17020, #2074, #25723, #8756, #14876, #17167, #25870, #6339, #15013, #2219, #4208, #10883, #12867, #19592, #6477, #15152, #4350, #75, #2780, #13866, #4921, #22447, #4774, #22019, #15730, #6898, #358, #13584, #18016, #20452, #11444, #11302, #20164, #24579, #22162, #7320, #24863, #646, #9184, #11726, #15585, #17737, #9319, #24293, #934, #26727, #24723, #7172, #5061, #22305, #15869, #18307, #22592, #5201, #13725, #5343, #19873, #9605, #2914, #2640, #26583, #11584, #20305, #13435, #20023, #26439, #16009, #3060, #790, #9460, #17877, #2496, #503, #7032, #24434, #27014, #7461, #18163, #26874, #11158 ) ),
 .UNSPECIFIED., .F., .F., .T. ) 
 B_SPLINE_SURFACE_WITH_KNOTS ( ( 2, 2 ),
 ( 3, 2, 2, 2, 2, 2, 2, 2, 2, 2, 2, 2, 2, 2, 2, 2, 2, 2, 2, 2, 2, 2, 2, 2, 2, 2, 2, 2, 2, 2, 2, 2, 2, 2, 2, 2, 2, 2, 2, 2, 2, 2, 2, 2, 2, 2, 2, 2, 2, 2, 2, 2, 2, 2, 2, 2, 2, 2, 2, 2, 2, 2, 2, 2, 2, 2, 2, 2, 2, 2, 2, 2, 2, 2, 2, 2, 2, 2, 2, 2, 2, 2, 2, 2, 2, 2, 2, 2, 2, 2, 2, 3 ),
 ( 0.000000000000000000, 1.000000000000000000 ),
 ( 0.000000000000000000, 0.01041666666666666609, 0.02083333333333333218, 0.03125000000000000000, 0.04166666666666666435, 0.05208333333333333565, 0.06250000000000000000, 0.07291666666666667129, 0.08333333333333332871, 0.09375000000000000000, 0.1041666666666666713, 0.1145833333333333287, 0.1250000000000000000, 0.1354166666666666574, 0.1458333333333333426, 0.1562500000000000000, 0.1666666666666666574, 0.1770833333333333426, 0.1875000000000000000, 0.1979166666666666574, 0.2083333333333333426, 0.2187500000000000000, 0.2291666666666666574, 0.2395833333333333426, 0.2500000000000000000, 0.2604166666666666852, 0.2708333333333333148, 0.2812500000000000000, 0.2916666666666666852, 0.3020833333333333148, 0.3125000000000000000, 0.3229166666666666852, 0.3333333333333333148, 0.3437500000000000000, 0.3541666666666666852, 0.3645833333333333148, 0.3750000000000000000, 0.3854166666666666852, 0.3958333333333333148, 0.4062500000000000000, 0.4166666666666666852, 0.4270833333333333148, 0.4375000000000000000, 0.4479166666666666852, 0.4583333333333333148, 0.4687500000000000000, 0.4791666666666666852, 0.4895833333333333148, 0.5000000000000000000, 0.5104166666666666297, 0.5208333333333333703, 0.5312500000000000000, 0.5416666666666666297, 0.5520833333333333703, 0.5625000000000000000, 0.5729166666666666297, 0.5833333333333333703, 0.5937500000000000000, 0.6041666666666666297, 0.6145833333333333703, 0.6250000000000000000, 0.6354166666666666297, 0.6458333333333333703, 0.6562500000000000000, 0.6666666666666666297, 0.6770833333333333703, 0.6875000000000000000, 0.6979166666666666297, 0.7083333333333333703, 0.7187500000000000000, 0.7291666666666666297, 0.7395833333333333703, 0.7500000000000000000, 0.7604166666666666297, 0.7708333333333333703, 0.7812500000000000000, 0.7916666666666666297, 0.8020833333333333703, 0.8125000000000000000, 0.8229166666666666297, 0.8333333333333333703, 0.8437500000000000000, 0.8541666666666666297, 0.8645833333333333703, 0.8750000000000000000, 0.8854166666666666297, 0.8958333333333333703, 0.9062500000000000000, 0.9166666666666666297, 0.9270833333333333703, 0.9375000000000000000, 0.9448587001587775980 ),
 .UNSPECIFIED. ) 
 GEOMETRIC_REPRESENTATION_ITEM ( )  RATIONAL_B_SPLINE_SURFACE ( (
 ( 1.000000000000000000, 0.9238795325112867385, 1.000000000000000000, 0.9238795325112867385, 1.000000000000000000, 0.9238795325112867385, 1.000000000000000000, 0.9238795325112867385, 1.000000000000000000, 0.9238795325112867385, 1.000000000000000000, 0.9238795325112867385, 1.000000000000000000, 0.9238795325112867385, 1.000000000000000000, 0.9238795325112867385, 1.000000000000000000, 0.9238795325112867385, 1.000000000000000000, 0.9238795325112867385, 1.000000000000000000, 0.9238795325112867385, 1.000000000000000000, 0.9238795325112867385, 1.000000000000000000, 0.9238795325112867385, 1.000000000000000000, 0.9238795325112867385, 1.000000000000000000, 0.9238795325112867385, 1.000000000000000000, 0.9238795325112867385, 1.000000000000000000, 0.9238795325112867385, 1.000000000000000000, 0.9238795325112867385, 1.000000000000000000, 0.9238795325112867385, 1.000000000000000000, 0.9238795325112867385, 1.000000000000000000, 0.9238795325112867385, 1.000000000000000000, 0.9238795325112867385, 1.000000000000000000, 0.9238795325112867385, 1.000000000000000000, 0.9238795325112867385, 1.000000000000000000, 0.9238795325112867385, 1.000000000000000000, 0.9238795325112867385, 1.000000000000000000, 0.9238795325112867385, 1.000000000000000000, 0.9238795325112867385, 1.000000000000000000, 0.9238795325112867385, 1.000000000000000000, 0.9238795325112867385, 1.000000000000000000, 0.9238795325112867385, 1.000000000000000000, 0.9238795325112867385, 1.000000000000000000, 0.9238795325112867385, 1.000000000000000000, 0.9238795325112867385, 1.000000000000000000, 0.9238795325112867385, 1.000000000000000000, 0.9238795325112867385, 1.000000000000000000, 0.9238795325112867385, 1.000000000000000000, 0.9238795325112867385, 1.000000000000000000, 0.9238795325112867385, 1.000000000000000000, 0.9238795325112867385, 1.000000000000000000, 0.9238795325112867385, 1.000000000000000000, 0.9238795325112867385, 1.000000000000000000, 0.9238795325112867385, 1.000000000000000000, 0.9238795325112867385, 1.000000000000000000, 0.9238795325112867385, 1.000000000000000000, 0.9238795325112867385, 1.000000000000000000, 0.9238795325112867385, 1.000000000000000000, 0.9238795325112867385, 1.000000000000000000, 0.9238795325112867385, 1.000000000000000000, 0.9238795325112867385, 1.000000000000000000, 0.9238795325112867385, 1.000000000000000000, 0.9238795325112867385, 1.000000000000000000, 0.9238795325112867385, 1.000000000000000000, 0.9238795325112867385, 1.000000000000000000, 0.9238795325112867385, 1.000000000000000000, 0.9238795325112867385, 1.000000000000000000, 0.9238795325112867385, 1.000000000000000000, 0.9238795325112867385, 1.000000000000000000, 0.9238795325112867385, 1.000000000000000000, 0.9238795325112867385, 1.000000000000000000, 0.9238795325112867385, 1.000000000000000000, 0.9238795325112867385, 1.000000000000000000, 0.9238795325112867385, 1.000000000000000000, 0.9238795325112867385, 1.000000000000000000, 0.9238795325112867385, 1.000000000000000000, 0.9238795325112867385, 1.000000000000000000, 0.9238795325112867385, 1.000000000000000000, 0.9238795325112867385, 1.000000000000000000, 0.9238795325112867385, 1.000000000000000000, 0.9238795325112867385, 1.000000000000000000, 0.9238795325112867385, 1.000000000000000000, 0.9238795325112867385, 1.000000000000000000, 0.9238795325112867385, 1.000000000000000000, 0.9238795325112867385, 1.000000000000000000, 0.9238795325112867385, 1.000000000000000000, 0.9238795325112867385, 1.000000000000000000, 0.9238795325112867385, 1.000000000000000000, 0.9238795325112867385, 1.000000000000000000, 0.9238795325112867385, 1.000000000000000000, 0.9238795325112867385, 1.000000000000000000, 0.9238795325112867385, 1.000000000000000000, 0.9238795325112867385, 1.000000000000000000, 0.9238795325112867385, 1.000000000000000000, 0.9238795325112867385, 1.000000000000000000, 0.9238795325112867385, 1.000000000000000000, 0.9238795325112867385, 1.000000000000000000, 0.9238795325112867385, 1.000000000000000000, 0.9238795325112867385, 1.000000000000000000, 0.9238795325112867385, 1.000000000000000000, 0.9238795325112867385, 1.000000000000000000, 0.9462258211652395667, 0.9684275895297407288),
 ( 1.000000000000000000, 0.9238795325112867385, 1.000000000000000000, 0.9238795325112867385, 1.000000000000000000, 0.9238795325112867385, 1.000000000000000000, 0.9238795325112867385, 1.000000000000000000, 0.9238795325112867385, 1.000000000000000000, 0.9238795325112867385, 1.000000000000000000, 0.9238795325112867385, 1.000000000000000000, 0.9238795325112867385, 1.000000000000000000, 0.9238795325112867385, 1.000000000000000000, 0.9238795325112867385, 1.000000000000000000, 0.9238795325112867385, 1.000000000000000000, 0.9238795325112867385, 1.000000000000000000, 0.9238795325112867385, 1.000000000000000000, 0.9238795325112867385, 1.000000000000000000, 0.9238795325112867385, 1.000000000000000000, 0.9238795325112867385, 1.000000000000000000, 0.9238795325112867385, 1.000000000000000000, 0.9238795325112867385, 1.000000000000000000, 0.9238795325112867385, 1.000000000000000000, 0.9238795325112867385, 1.000000000000000000, 0.9238795325112867385, 1.000000000000000000, 0.9238795325112867385, 1.000000000000000000, 0.9238795325112867385, 1.000000000000000000, 0.9238795325112867385, 1.000000000000000000, 0.9238795325112867385, 1.000000000000000000, 0.9238795325112867385, 1.000000000000000000, 0.9238795325112867385, 1.000000000000000000, 0.9238795325112867385, 1.000000000000000000, 0.9238795325112867385, 1.000000000000000000, 0.9238795325112867385, 1.000000000000000000, 0.9238795325112867385, 1.000000000000000000, 0.9238795325112867385, 1.000000000000000000, 0.9238795325112867385, 1.000000000000000000, 0.9238795325112867385, 1.000000000000000000, 0.9238795325112867385, 1.000000000000000000, 0.9238795325112867385, 1.000000000000000000, 0.9238795325112867385, 1.000000000000000000, 0.9238795325112867385, 1.000000000000000000, 0.9238795325112867385, 1.000000000000000000, 0.9238795325112867385, 1.000000000000000000, 0.9238795325112867385, 1.000000000000000000, 0.9238795325112867385, 1.000000000000000000, 0.9238795325112867385, 1.000000000000000000, 0.9238795325112867385, 1.000000000000000000, 0.9238795325112867385, 1.000000000000000000, 0.9238795325112867385, 1.000000000000000000, 0.9238795325112867385, 1.000000000000000000, 0.9238795325112867385, 1.000000000000000000, 0.9238795325112867385, 1.000000000000000000, 0.9238795325112867385, 1.000000000000000000, 0.9238795325112867385, 1.000000000000000000, 0.9238795325112867385, 1.000000000000000000, 0.9238795325112867385, 1.000000000000000000, 0.9238795325112867385, 1.000000000000000000, 0.9238795325112867385, 1.000000000000000000, 0.9238795325112867385, 1.000000000000000000, 0.9238795325112867385, 1.000000000000000000, 0.9238795325112867385, 1.000000000000000000, 0.9238795325112867385, 1.000000000000000000, 0.9238795325112867385, 1.000000000000000000, 0.9238795325112867385, 1.000000000000000000, 0.9238795325112867385, 1.000000000000000000, 0.9238795325112867385, 1.000000000000000000, 0.9238795325112867385, 1.000000000000000000, 0.9238795325112867385, 1.000000000000000000, 0.9238795325112867385, 1.000000000000000000, 0.9238795325112867385, 1.000000000000000000, 0.9238795325112867385, 1.000000000000000000, 0.9238795325112867385, 1.000000000000000000, 0.9238795325112867385, 1.000000000000000000, 0.9238795325112867385, 1.000000000000000000, 0.9238795325112867385, 1.000000000000000000, 0.9238795325112867385, 1.000000000000000000, 0.9238795325112867385, 1.000000000000000000, 0.9238795325112867385, 1.000000000000000000, 0.9238795325112867385, 1.000000000000000000, 0.9238795325112867385, 1.000000000000000000, 0.9238795325112867385, 1.000000000000000000, 0.9238795325112867385, 1.000000000000000000, 0.9238795325112867385, 1.000000000000000000, 0.9238795325112867385, 1.000000000000000000, 0.9238795325112867385, 1.000000000000000000, 0.9238795325112867385, 1.000000000000000000, 0.9238795325112867385, 1.000000000000000000, 0.9238795325112867385, 1.000000000000000000, 0.9238795325112867385, 1.000000000000000000, 0.9238795325112867385, 1.000000000000000000, 0.9238795325112867385, 1.000000000000000000, 0.9238795325112867385, 1.000000000000000000, 0.9238795325112867385, 1.000000000000000000, 0.9462258211652395667, 0.9684275895297407288) ) ) 
 REPRESENTATION_ITEM ( '' )  SURFACE ( )  );
#23050=CARTESIAN_POINT ( 'NONE',  ( 185.8843427382057882, 36.00000000000002132, 9.510219181138902300 ) ) ;
#23052=CARTESIAN_POINT ( 'NONE',  ( 5.444914386472297529, 40.30546875108393579, -13.14518615778179900 ) ) ;
#23053=CARTESIAN_POINT ( 'NONE',  ( 136.1066586549483191, 35.99999999999999289, 11.74215035806533258 ) ) ;
#23056=CARTESIAN_POINT ( 'NONE',  ( 127.1079374786957317, 36.00000000000001421, -13.15766692561454754 ) ) ;
#23057=CARTESIAN_POINT ( 'NONE',  ( 181.4251840539369596, 39.56132812716787583, 5.622872871577880183 ) ) ;
#23060=VERTEX_POINT ( 'NONE', #22207 ) ;
#23066=CARTESIAN_POINT ( 'NONE',  ( 104.4587341249999781, 80.87500000136560629, 1.846868145590721655 ) ) ;
#23067=CARTESIAN_POINT ( 'NONE',  ( 51.85481384221819923, 33.36015625108393579, -5.444914386472297529 ) ) ;
#23071=VECTOR ( 'NONE', #12680, 1000.000000000000227 ) ;
#23073=CARTESIAN_POINT ( 'NONE',  ( 59.37712712842198926, 38.86679687716787868, 13.57481594606290720 ) ) ;
#23075=CARTESIAN_POINT ( 'NONE',  ( 116.8548138422182063, 33.65781250108393152, 5.444914386472304635 ) ) ;
#23078=CARTESIAN_POINT ( 'NONE',  ( 143.5748159460630688, 37.52734375216787299, -1.662435489736055892E-15 ) ) ;
#23081=CARTESIAN_POINT ( 'NONE',  ( 135.4449143864723055, 38.71796875108393721, -13.14518615778179900 ) ) ;
#23082=CARTESIAN_POINT ( 'NONE',  ( 208.5748159460630688, 37.42812499999999432, -1.662435489736055892E-15 ) ) ;
#23083=AXIS2_PLACEMENT_3D ( 'NONE', #16569, #8155, #12545 ) ;
#23085=CARTESIAN_POINT ( 'NONE',  ( -13.57481594606304753, 40.25585937716787299, -5.622872871577873077 ) ) ;
#23088=ORIENTED_EDGE ( 'NONE', *, *, #27991, .F. ) ;
#23090=CARTESIAN_POINT ( 'NONE',  ( 185.4011555911795313, 32.26875000216787726, -9.598844408820458085 ) ) ;
#23094=CARTESIAN_POINT ( 'NONE',  ( 135.4449143864723339, 37.62656250108393152, 13.14518615778179189 ) ) ;
#23095=CARTESIAN_POINT ( 'NONE',  ( -13.14518615778179900, 31.97109375108393436, -5.444914386472297529 ) ) ;
#23096=CARTESIAN_POINT ( 'NONE',  ( 143.5748159460630688, 37.37851562499999858, 5.622872871577868636 ) ) ;
#23099=EDGE_CURVE ( 'NONE', #12810, #12494, #4969, .T. ) ;
#23100=CARTESIAN_POINT ( 'NONE',  ( 208.1451861577817795, 32.46718750108393436, -5.444914386472297529 ) ) ;
#23102=CARTESIAN_POINT ( 'NONE',  ( 51.42518405393695957, 39.41249999999999432, 0.000000000000000000 ) ) ;
#23110=CARTESIAN_POINT ( 'NONE',  ( 13.57481594606304753, 39.06523437499998863, -5.622872871577873077 ) ) ;
#23111=ADVANCED_FACE ( 'NONE', ( #27060 ), #17784, .T. ) ;
#23112=ORIENTED_EDGE ( 'NONE', *, *, #11224, .F. ) ;
#23113=CARTESIAN_POINT ( 'NONE',  ( 98.15313185440925281, 83.50000000136560629, -4.458734125000016313 ) ) ;
#23116=ORIENTED_EDGE ( 'NONE', *, *, #10096, .T. ) ;
#23119=CARTESIAN_POINT ( 'NONE',  ( 196.6025331306099986, 53.60343507247939243, -15.00000000000000000 ) ) ;
#23121=VERTEX_POINT ( 'NONE', #13341 ) ;
#23124=CARTESIAN_POINT ( 'NONE',  ( 208.5748159460630688, 39.90859375216787441, -1.662435489736055892E-15 ) ) ;
#23127=CARTESIAN_POINT ( 'NONE',  ( -9.295050272127044266, 36.08867187608393579, 9.295050272127047819 ) ) ;
#23128=CARTESIAN_POINT ( 'NONE',  ( -13.14518615778179189, 31.87187500108393223, 5.444914386472304635 ) ) ;
#23129=CARTESIAN_POINT ( 'NONE',  ( 78.57481594606305464, 38.22187499999999716, -1.662435489736055892E-15 ) ) ;
#23130=CARTESIAN_POINT ( 'NONE',  ( 59.37712712842210294, 39.66054687716787441, 13.57481594606302444 ) ) ;
#23131=DIRECTION ( 'NONE',  ( 0.000000000000000000, -1.000000000000000000, 0.000000000000000000 ) ) ;
#23134=( BOUNDED_CURVE ( )  B_SPLINE_CURVE ( 2, ( #5484, #26728, #16010, #18164, #11727, #15870, #20734, #26584, #24724 ),
 .UNSPECIFIED., .F., .F. ) 
 B_SPLINE_CURVE_WITH_KNOTS ( ( 3, 2, 2, 2, 3 ),
 ( 0.3125000000000002220, 0.3229166666666668517, 0.3333333333333334259, 0.3437500000000000555, 0.3541666666666666852 ),
 .UNSPECIFIED. ) 
 CURVE ( )  GEOMETRIC_REPRESENTATION_ITEM ( )  RATIONAL_B_SPLINE_CURVE ( ( 0.9999999999999983347, 0.9238795325112884038, 1.000000000000000000, 0.9238795325112867385, 1.000000000000000000, 0.9238795325112867385, 1.000000000000000000, 0.9238795325112867385, 1.000000000000000000 ) ) 
 REPRESENTATION_ITEM ( '' )  );
#23135=CARTESIAN_POINT ( 'NONE',  ( 96.84719886470459471, 84.56250000136560629, -3.152801135295383084 ) ) ;
#23139=CARTESIAN_POINT ( 'NONE',  ( 66.88752872587643594, 53.66306546785492060, 14.99999999999998579 ) ) ;
#23140=EDGE_LOOP ( 'NONE', ( #15658, #1782 ) ) ;
#23141=DIRECTION ( 'NONE',  ( 0.000000000000000000, 0.000000000000000000, -1.000000000000000000 ) ) ;
#23149=CARTESIAN_POINT ( 'NONE',  ( 70.44491438647229131, 38.91640625108393436, -13.14518615778179722 ) ) ;
#23150=CARTESIAN_POINT ( 'NONE',  ( 1.417506129906585004E-15, 52.00000000000000711, -11.57481594606304398 ) ) ;
#23152=DIRECTION ( 'NONE',  ( -0.000000000000000000, 1.000000000000000000, -0.000000000000000000 ) ) ;
#23154=DIRECTION ( 'NONE',  ( -0.8660254037844407060, 0.4999999999999963363, 0.000000000000000000 ) ) ;
#23156=CARTESIAN_POINT ( 'NONE',  ( 0.000000000000000000, -7.395377635281828788, 13.57481594606304398 ) ) ;
#23157=CARTESIAN_POINT ( 'NONE',  ( 124.3771271284221314, 35.69179687716786731, 13.57481594606304753 ) ) ;
#23160=CARTESIAN_POINT ( 'NONE',  ( 200.4449143864723055, 38.91640625108393436, -13.14518615778179900 ) ) ;
#23161=EDGE_LOOP ( 'NONE', ( #9492, #318, #15507, #7243 ) ) ;
#23164=CARTESIAN_POINT ( 'NONE',  ( 99.99999999999995737, 84.25000000000000000, 4.999999999999990230 ) ) ;
#23165=CARTESIAN_POINT ( 'NONE',  ( 2.493653234604083739E-15, 39.61093749999999147, 13.57481594606304576 ) ) ;
#23166=AXIS2_PLACEMENT_3D ( 'NONE', #17069, #2121, #6252 ) ;
#23171=CARTESIAN_POINT ( 'NONE',  ( 99.99999999999995737, 80.75000000000000000, -5.000000000000018652 ) ) ;
#23172=VECTOR ( 'NONE', #23295, 1000.000000000000000 ) ;
#23176=ORIENTED_EDGE ( 'NONE', *, *, #25386, .F. ) ;
#23177=CARTESIAN_POINT ( 'NONE',  ( 78.57481594606305464, 36.68398437500000142, -5.622872871577873966 ) ) ;
#23183=CARTESIAN_POINT ( 'NONE',  ( 116.8548138422182063, 40.00781250108393294, 5.444914386472304635 ) ) ;
#23184=CARTESIAN_POINT ( 'NONE',  ( 55.70494972787295751, 37.47773437608393010, 9.295050272127047819 ) ) ;
#23185=EDGE_CURVE ( 'NONE', #14316, #21981, #9649, .T. ) ;
#23187=CARTESIAN_POINT ( 'NONE',  ( -13.14518615778179189, 34.25312500108393010, 5.444914386472304635 ) ) ;
#23191=CARTESIAN_POINT ( 'NONE',  ( 130.0000000000000000, 40.00781250000000000, -13.57481594606304576 ) ) ;
#23192=CARTESIAN_POINT ( 'NONE',  ( 130.0000000000000000, 37.22968749999999716, 13.57481594606304576 ) ) ;
#23194=CARTESIAN_POINT ( 'NONE',  ( -5.444914386472297529, 38.02343750108394005, -13.14518615778179900 ) ) ;
#23199=DIRECTION ( 'NONE',  ( 0.000000000000000000, 0.000000000000000000, -1.000000000000000000 ) ) ;
#23200=FACE_OUTER_BOUND ( 'NONE', #5896, .T. ) ;
#23208=CARTESIAN_POINT ( 'NONE',  ( 101.8468681455906903, 83.37500000136563472, -4.458734125000016313 ) ) ;
#23209=CARTESIAN_POINT ( 'NONE',  ( 70.44491438647230552, 39.41250000108393436, 13.14518615778179189 ) ) ;
#23215=CARTESIAN_POINT ( 'NONE',  ( 124.3771271284221314, 40.05742187499999574, -13.57481594606304753 ) ) ;
#23216=ORIENTED_EDGE ( 'NONE', *, *, #4427, .F. ) ;
#23220=CARTESIAN_POINT ( 'NONE',  ( 116.8548138422182205, 38.96601562608393721, 0.000000000000000000 ) ) ;
#23221=CARTESIAN_POINT ( 'NONE',  ( 78.57481594606304043, 38.37070312716786447, -5.622872871577873077 ) ) ;
#23222=EDGE_CURVE ( 'NONE', #13505, #2344, #14708, .T. ) ;
#23224=CARTESIAN_POINT ( 'NONE',  ( -5.622872871577873077, 34.89804687716787868, 13.57481594606304753 ) ) ;
#23225=ORIENTED_EDGE ( 'NONE', *, *, #8793, .T. ) ;
#23229=CARTESIAN_POINT ( 'NONE',  ( 195.0000000000000000, 32.16953125216787157, -13.57481594606304576 ) ) ;
#23231=CARTESIAN_POINT ( 'NONE',  ( 139.2950502721270425, 39.46210937608393010, -9.295050272127046043 ) ) ;
#23232=CARTESIAN_POINT ( 'NONE',  ( -9.295050272127046043, 32.71523437608393436, -9.295050272127046043 ) ) ;
#23234=DIRECTION ( 'NONE',  ( -2.385244779468110248E-16, 0.000000000000000000, -1.000000000000000000 ) ) ;
#23237=CARTESIAN_POINT ( 'NONE',  ( 181.4251840539369596, 37.08085937499999574, 5.622872871577880183 ) ) ;
#23239=CARTESIAN_POINT ( 'NONE',  ( 65.00000000000000000, 39.21406249999999716, -13.57481594606304576 ) ) ;
#23241=CARTESIAN_POINT ( 'NONE',  ( 51.85481384221820633, 38.17226562608393436, 0.000000000000000000 ) ) ;
#23246=CARTESIAN_POINT ( 'NONE',  ( 120.4011555911795455, 39.31328124999999574, -9.598844408820458085 ) ) ;
#23247=CARTESIAN_POINT ( 'NONE',  ( -5.622872871577873077, 39.56132812499999574, 13.57481594606304753 ) ) ;
#23248=EDGE_LOOP ( 'NONE', ( #1470, #9443, #8830, #423 ) ) ;
#23249=CARTESIAN_POINT ( 'NONE',  ( 95.54126587499996504, 81.68750000136559208, -1.387778780781445676E-14 ) ) ;
#23250=ADVANCED_FACE ( 'NONE', ( #24628 ), #11631, .T. ) ;
#23253=ORIENTED_EDGE ( 'NONE', *, *, #11918, .F. ) ;
#23255=EDGE_CURVE ( 'NONE', #26813, #8417, #25321, .T. ) ;
#23262=CARTESIAN_POINT ( 'NONE',  ( 9.598844408820456309, 36.03906250216787299, -9.598844408820458085 ) ) ;
#23264=EDGE_CURVE ( 'NONE', #18668, #17777, #16349, .T. ) ;
#23266=CARTESIAN_POINT ( 'NONE',  ( 116.8548138422182205, 39.95820312608393010, 0.000000000000000000 ) ) ;
#23267=CARTESIAN_POINT ( 'NONE',  ( 13.14518615778179544, 32.21914062608393436, -1.609821015232357215E-15 ) ) ;
#23269=CARTESIAN_POINT ( 'NONE',  ( 55.40115559117954547, 37.92421874999999432, 9.598844408820459861 ) ) ;
#23271=EDGE_CURVE ( 'NONE', #17231, #21964, #20521, .T. ) ;
#23276=CARTESIAN_POINT ( 'NONE',  ( 103.1528011352953342, 82.06250000136559208, 3.152801135295355106 ) ) ;
#23278=CARTESIAN_POINT ( 'NONE',  ( 13.14518615778179900, 39.51171875108392584, 5.444914386472293977 ) ) ;
#23279=ADVANCED_FACE ( 'NONE', ( #22780 ), #7799, .T. ) ;
#23280=AXIS2_PLACEMENT_3D ( 'NONE', #23503, #10514, #25633 ) ;
#23284=CYLINDRICAL_SURFACE ( 'NONE', #7105, 5.000000000000004441 ) ;
#23286=EDGE_CURVE ( 'NONE', #1089, #17753, #21187, .T. ) ;
#23288=ORIENTED_EDGE ( 'NONE', *, *, #112, .F. ) ;
#23289=CARTESIAN_POINT ( 'NONE',  ( 78.14518615778180788, 39.61093750108393863, -5.444914386472297529 ) ) ;
#23290=DIRECTION ( 'NONE',  ( 1.000000000000000000, 0.000000000000000000, -0.000000000000000000 ) ) ;
#23292=ORIENTED_EDGE ( 'NONE', *, *, #27456, .T. ) ;
#23295=DIRECTION ( 'NONE',  ( -0.000000000000000000, 1.000000000000000000, -0.000000000000000000 ) ) ;
#23296=DIRECTION ( 'NONE',  ( -1.000000000000000000, 0.000000000000000000, 0.000000000000000000 ) ) ;
#23298=CARTESIAN_POINT ( 'NONE',  ( 124.3771271284221314, 33.01289062716787726, -13.57481594606304753 ) ) ;
#23302=CARTESIAN_POINT ( 'NONE',  ( 185.7049497278729575, 36.68398437608393436, -9.295050272127046043 ) ) ;
#23303=ORIENTED_EDGE ( 'NONE', *, *, #22909, .F. ) ;
#23304=VERTEX_POINT ( 'NONE', #10894 ) ;
#23306=CARTESIAN_POINT ( 'NONE',  ( 130.0000000000000000, -7.395377635281828788, 13.57481594606302799 ) ) ;
#23312=CARTESIAN_POINT ( 'NONE',  ( 9.031440422454179995, 36.00000000000002132, 9.765766397119126196 ) ) ;
#23313=DIRECTION ( 'NONE',  ( 0.000000000000000000, 0.000000000000000000, -1.000000000000000000 ) ) ;
#23319=CARTESIAN_POINT ( 'NONE',  ( 143.1451861577818079, 39.56132812608393579, -1.609821015232357215E-15 ) ) ;
#23320=CARTESIAN_POINT ( 'NONE',  ( 70.44491438647230552, 36.33671875108394289, -13.14518615778179900 ) ) ;
#23322=CARTESIAN_POINT ( 'NONE',  ( 52.62412159965071368, 36.00000000000000000, 4.513979326318426466 ) ) ;
#23323=CARTESIAN_POINT ( 'NONE',  ( -13.14518615778179900, 35.74140625108393721, -5.444914386472297529 ) ) ;
#23324=CARTESIAN_POINT ( 'NONE',  ( 190.5405265863611817, 36.00000000000001421, -12.68347323196760890 ) ) ;
#23327=CARTESIAN_POINT ( 'NONE',  ( -5.444914386472297529, 39.61093750108393152, -13.14518615778179900 ) ) ;
#23328=CARTESIAN_POINT ( 'NONE',  ( 142.0772764098356333, 36.00000000000000000, -6.197985357349214297 ) ) ;
#23335=ORIENTED_EDGE ( 'NONE', *, *, #8087, .T. ) ;
#23339=CIRCLE ( 'NONE', #16502, 11.57481594606304398 ) ;
#23341=CARTESIAN_POINT ( 'NONE',  ( 181.4251840539369596, 36.33671875216787583, 0.000000000000000000 ) ) ;
#23342=CARTESIAN_POINT ( 'NONE',  ( 95.54126587499995082, 84.62500000136560629, -1.846868145590750077 ) ) ;
#23343=CARTESIAN_POINT ( 'NONE',  ( 59.55508561352770158, 39.80937500108392868, -13.14518615778179900 ) ) ;
#23344=( BOUNDED_CURVE ( )  B_SPLINE_CURVE ( 2, ( #14035, #3360, #12031, #20754, #22760, #3646, #9485, #817, #18187 ),
 .UNSPECIFIED., .F., .F. ) 
 B_SPLINE_CURVE_WITH_KNOTS ( ( 3, 2, 2, 2, 3 ),
 ( 0.06250000000000004163, 0.07291666666666665741, 0.08333333333333325932, 0.09374999999999987510, 0.1041666666666664909 ),
 .UNSPECIFIED. ) 
 CURVE ( )  GEOMETRIC_REPRESENTATION_ITEM ( )  RATIONAL_B_SPLINE_CURVE ( ( 0.9999999999999996669, 0.9238795325112870716, 1.000000000000000000, 0.9238795325112867385, 1.000000000000000000, 0.9238795325112867385, 1.000000000000000000, 0.9238795325112880708, 0.9999999999999986677 ) ) 
 REPRESENTATION_ITEM ( '' )  );
#23346=CYLINDRICAL_SURFACE ( 'NONE', #20964, 13.57481594606304398 ) ;
#23350=CARTESIAN_POINT ( 'NONE',  ( 116.4251840539369596, 39.41249999999999432, 0.000000000000000000 ) ) ;
#23354=CARTESIAN_POINT ( 'NONE',  ( 104.4587341249999639, 80.93750000136559208, -1.442382525525748735E-14 ) ) ;
#23355=CARTESIAN_POINT ( 'NONE',  ( 135.4449143864723055, 40.00781250108393294, 13.14518615778179189 ) ) ;
#23356=CARTESIAN_POINT ( 'NONE',  ( 51.42518405393695957, 37.08085937716786873, -5.622872871577873077 ) ) ;
#23358=CARTESIAN_POINT ( 'NONE',  ( -5.622872871577873077, 36.48554687716787015, 13.57481594606304753 ) ) ;
#23364=CARTESIAN_POINT ( 'NONE',  ( 195.0000000000000000, 38.76757812608393294, -13.14518615778179544 ) ) ;
#23366=CARTESIAN_POINT ( 'NONE',  ( 116.8548138422182205, 38.17226562608393436, 0.000000000000000000 ) ) ;
#23367=LINE ( 'NONE', #8666, #20081 ) ;
#23368=CARTESIAN_POINT ( 'NONE',  ( 139.5988444088204687, 37.32890624999999574, 9.598844408820456309 ) ) ;
#23370=CYLINDRICAL_SURFACE ( 'NONE', #20272, 13.57481594606304398 ) ;
#23372=CARTESIAN_POINT ( 'NONE',  ( 195.0000000000000000, 37.62656249999999858, -13.57481594606304576 ) ) ;
#23376=CARTESIAN_POINT ( 'NONE',  ( 51.85481384221819923, 39.71015625108393010, -5.444914386472297529 ) ) ;
#23377=EDGE_CURVE ( 'NONE', #27310, #4145, #1098, .T. ) ;
#23382=CARTESIAN_POINT ( 'NONE',  ( 2.493653234604083739E-15, 39.61093749999999147, 13.57481594606304576 ) ) ;
#23385=CARTESIAN_POINT ( 'NONE',  ( 96.84719886470459471, 82.81250000136560629, 3.152801135295355994 ) ) ;
#23390=ORIENTED_EDGE ( 'NONE', *, *, #20317, .T. ) ;
#23393=EDGE_LOOP ( 'NONE', ( #28059, #12684, #17665, #16772 ) ) ;
#23396=CARTESIAN_POINT ( 'NONE',  ( 200.6228728715778686, 39.26367187716787299, -13.57481594606304753 ) ) ;
#23399=CARTESIAN_POINT ( 'NONE',  ( 193.9858691739322012, 51.45790058219657936, 15.00000000000130029 ) ) ;
#23400=CARTESIAN_POINT ( 'NONE',  ( 143.1451861577818363, 37.92421875108393436, 5.444914386472293977 ) ) ;
#23401=CARTESIAN_POINT ( 'NONE',  ( 9.295050272127046043, 33.11210937608393579, -9.295050272127046043 ) ) ;
#23403=CARTESIAN_POINT ( 'NONE',  ( 70.62287287157786864, 36.78320312499999289, -13.57481594606304753 ) ) ;
#23404=FACE_OUTER_BOUND ( 'NONE', #23022, .T. ) ;
#23405=CARTESIAN_POINT ( 'NONE',  ( 207.6678442549460328, 36.00000000000000711, 4.396229039743087874 ) ) ;
#23409=EDGE_CURVE ( 'NONE', #4741, #10253, #23467, .T. ) ;
#23410=CARTESIAN_POINT ( 'NONE',  ( 101.8468681455907046, 82.00000000136560629, 4.458734124999987891 ) ) ;
#23412=CARTESIAN_POINT ( 'NONE',  ( 2.414731522848535132E-15, 38.56914062608393579, 13.14518615778179544 ) ) ;
#23414=VERTEX_POINT ( 'NONE', #19602 ) ;
#23415=EDGE_CURVE ( 'NONE', #22018, #10089, #26017, .T. ) ;
#23416=DIRECTION ( 'NONE',  ( 0.000000000000000000, -1.000000000000000000, 0.000000000000000000 ) ) ;
#23417=CARTESIAN_POINT ( 'NONE',  ( 2.493653234604083739E-15, 39.71015625216787015, 13.57481594606304576 ) ) ;
#23419=CARTESIAN_POINT ( 'NONE',  ( 65.00000000000000000, 38.12265625216787157, 13.57481594606304576 ) ) ;
#23423=CARTESIAN_POINT ( 'NONE',  ( 51.85481384221820633, 37.52734375108393294, -5.444914386472297529 ) ) ;
#23424=FACE_OUTER_BOUND ( 'NONE', #13946, .T. ) ;
#23426=CARTESIAN_POINT ( 'NONE',  ( 195.0000000000000000, -7.395377635281828788, -2.255140518769849538E-14 ) ) ;
#23432=CARTESIAN_POINT ( 'NONE',  ( 116.4251840539369596, 34.74921875216787726, 0.000000000000000000 ) ) ;
#23433=CARTESIAN_POINT ( 'NONE',  ( 51.85481384221820633, 40.75195312608393294, 0.000000000000000000 ) ) ;
#23435=CARTESIAN_POINT ( 'NONE',  ( 185.7049497278729575, 37.47773437608393010, -9.295050272127046043 ) ) ;
#23436=EDGE_LOOP ( 'NONE', ( #9128, #22295, #2643, #27943 ) ) ;
#23437=ORIENTED_EDGE ( 'NONE', *, *, #15861, .T. ) ;
#23442=DIRECTION ( 'NONE',  ( -0.000000000000000000, 1.000000000000000000, -0.000000000000000000 ) ) ;
#23445=DIRECTION ( 'NONE',  ( 0.000000000000000000, -1.000000000000000000, 0.000000000000000000 ) ) ;
#23451=EDGE_LOOP ( 'NONE', ( #15439, #6153, #12363, #5974 ) ) ;
#23455=CARTESIAN_POINT ( 'NONE',  ( 120.7049497278729575, 38.46992187608393721, 9.295050272127047819 ) ) ;
#23456=CARTESIAN_POINT ( 'NONE',  ( 78.14518615778179367, 36.98164062608393010, -1.609821015232357215E-15 ) ) ;
#23457=EDGE_CURVE ( 'NONE', #3371, #19109, #24591, .T. ) ;
#23458=CARTESIAN_POINT ( 'NONE',  ( 181.8548138422181921, 40.70234375108393721, -5.444914386472297529 ) ) ;
#23459=CARTESIAN_POINT ( 'NONE',  ( 95.27063293749995410, 79.84375000068280315, -1.387778780781445676E-14 ) ) ;
#23460=CARTESIAN_POINT ( 'NONE',  ( 2.414731522848535132E-15, 35.98945312608393010, 13.14518615778179544 ) ) ;
#23462=( BOUNDED_CURVE ( )  B_SPLINE_CURVE ( 2, ( #22657, #4986, #11935, #5264, #16366, #11507, #3267, #2975, #26939 ),
 .UNSPECIFIED., .F., .F. ) 
 B_SPLINE_CURVE_WITH_KNOTS ( ( 3, 2, 2, 2, 3 ),
 ( 0.3541666666666666852, 0.3645833333333332593, 0.3749999999999998890, 0.3854166666666665741, 0.3958333333333331483 ),
 .UNSPECIFIED. ) 
 CURVE ( )  GEOMETRIC_REPRESENTATION_ITEM ( )  RATIONAL_B_SPLINE_CURVE ( ( 1.000000000000000000, 0.9238795325112867385, 1.000000000000000000, 0.9238795325112867385, 1.000000000000000000, 0.9238795325112867385, 1.000000000000000000, 0.9238795325112879597, 0.9999999999999987788 ) ) 
 REPRESENTATION_ITEM ( '' )  );
#23464=CARTESIAN_POINT ( 'NONE',  ( 120.4011555911795455, 40.30546874999999574, 9.598844408820459861 ) ) ;
#23466=CARTESIAN_POINT ( 'NONE',  ( 5.444914386472302859, 40.00781250108393294, 13.14518615778179189 ) ) ;
#23467=LINE ( 'NONE', #17320, #4726 ) ;
#23479=CARTESIAN_POINT ( 'NONE',  ( 101.8468681455906903, 79.75000000136560629, 4.458734124999987891 ) ) ;
#23480=CARTESIAN_POINT ( 'NONE',  ( 51.85481384221820633, 39.95820312608393010, 0.000000000000000000 ) ) ;
#23482=CARTESIAN_POINT ( 'NONE',  ( 65.00000000000000000, -7.395377635281828788, -7.517135062566165128E-15 ) ) ;
#23483=CARTESIAN_POINT ( 'NONE',  ( 195.0000000000000000, 52.00000000000000711, -2.255140518769849538E-14 ) ) ;
#23484=CARTESIAN_POINT ( 'NONE',  ( 135.6228728715779255, 38.86679687500001279, 13.57481594606301023 ) ) ;
#23486=CARTESIAN_POINT ( 'NONE',  ( 143.1451861577818079, 32.41757812608393863, -1.609821015232357215E-15 ) ) ;
#23488=EDGE_LOOP ( 'NONE', ( #6595, #1186, #13132, #2321, #392, #19288, #13583, #7047, #4382, #8457, #6460, #22669 ) ) ;
#23491=CARTESIAN_POINT ( 'NONE',  ( 98.15313185440925281, 81.25000000136560629, -4.458734125000016313 ) ) ;
#23492=CARTESIAN_POINT ( 'NONE',  ( 139.2950502721270425, 40.25585937608393294, -9.295050272127046043 ) ) ;
#23493=CARTESIAN_POINT ( 'NONE',  ( 65.00000000000000000, 36.13828125216787157, -13.57481594606304576 ) ) ;
#23495=CARTESIAN_POINT ( 'NONE',  ( -5.622872871577873077, 35.39414062716787157, -13.57481594606304753 ) ) ;
#23497=ORIENTED_EDGE ( 'NONE', *, *, #25184, .F. ) ;
#23500=CARTESIAN_POINT ( 'NONE',  ( 195.0000000000000000, 36.78320312608393294, 13.14518615778179544 ) ) ;
#23501=DIRECTION ( 'NONE',  ( 0.000000000000000000, 0.000000000000000000, -1.000000000000000000 ) ) ;
#23502=CARTESIAN_POINT ( 'NONE',  ( 143.1451861577818079, 37.77539062608393294, -1.609821015232357215E-15 ) ) ;
#23503=CARTESIAN_POINT ( 'NONE',  ( 0.000000000000000000, -7.395377635281828788, 0.000000000000000000 ) ) ;
#23510=CARTESIAN_POINT ( 'NONE',  ( 185.4011555911795597, 36.33671874999999574, 9.598844408820459861 ) ) ;
#23514=CARTESIAN_POINT ( 'NONE',  ( 78.14518615778179367, 39.31328125108392868, 5.444914386472293977 ) ) ;
#23520=CARTESIAN_POINT ( 'NONE',  ( -9.598844408820454532, 38.71796874999999716, 9.598844408820459861 ) ) ;
#23521=CARTESIAN_POINT ( 'NONE',  ( 143.1451861577818079, 39.51171875108392584, 5.444914386472293977 ) ) ;
#23522=ORIENTED_EDGE ( 'NONE', *, *, #10708, .F. ) ;
#23523=CARTESIAN_POINT ( 'NONE',  ( 104.4587341249999639, 83.18750000136560629, -1.442382525525748735E-14 ) ) ;
#23527=CARTESIAN_POINT ( 'NONE',  ( 65.00000000000000000, 36.18789062608393436, 13.14518615778179544 ) ) ;
#23536=CARTESIAN_POINT ( 'NONE',  ( 189.3771271284221314, 36.48554687716787015, 13.57481594606304753 ) ) ;
#23538=LINE ( 'NONE', #19256, #13471 ) ;
#23539=CARTESIAN_POINT ( 'NONE',  ( 204.1801758136480203, 50.00000000000000711, 14.99999999999995559 ) ) ;
#23540=CARTESIAN_POINT ( 'NONE',  ( 120.7049497278729575, 40.65273437608393436, -9.295050272127046043 ) ) ;
#23541=CARTESIAN_POINT ( 'NONE',  ( -13.14518615778179544, 38.37070312608393152, 0.000000000000000000 ) ) ;
#23542=ORIENTED_EDGE ( 'NONE', *, *, #26955, .T. ) ;
#23543=CARTESIAN_POINT ( 'NONE',  ( 78.57481594606305464, 37.42812499999999432, -1.662435489736055892E-15 ) ) ;
#23544=CARTESIAN_POINT ( 'NONE',  ( 2.493653234604083739E-15, 38.12265625216787157, 13.57481594606304576 ) ) ;
#23550=CIRCLE ( 'NONE', #18555, 5.000000000000004441 ) ;
#23551=CARTESIAN_POINT ( 'NONE',  ( 104.4587341249999781, 81.12500000136560629, 1.846868145590721655 ) ) ;
#23553=CARTESIAN_POINT ( 'NONE',  ( 13.14518615778179900, 40.30546875108393579, 5.444914386472293977 ) ) ;
#23556=CARTESIAN_POINT ( 'NONE',  ( 204.1801758136479918, 55.00000000000000000, -10.00000000000000000 ) ) ;
#23559=CARTESIAN_POINT ( 'NONE',  ( 102.0710678118654329, 81.81250000273119838, -5.000000000000018652 ) ) ;
#23560=CARTESIAN_POINT ( 'NONE',  ( 2.493653234604083739E-15, 40.40468749999999432, 13.57481594606304576 ) ) ;
#23561=CARTESIAN_POINT ( 'NONE',  ( 200.4449143864723055, 39.21406250108392300, 13.14518615778179189 ) ) ;
#23563=CARTESIAN_POINT ( 'NONE',  ( 65.00000000000000000, 37.37851562608393863, -13.14518615778179544 ) ) ;
#23565=CARTESIAN_POINT ( 'NONE',  ( -8.312177448680279460E-16, 39.21406249999999716, -13.57481594606304576 ) ) ;
#23570=CARTESIAN_POINT ( 'NONE',  ( 139.5988444088204403, 34.45156250216787441, -9.598844408820458085 ) ) ;
#23571=CARTESIAN_POINT ( 'NONE',  ( 104.9999999999999716, 81.56250000273119838, 2.071067811865462627 ) ) ;
#23573=CARTESIAN_POINT ( 'NONE',  ( 185.7049497278729575, 33.70742187608393436, 9.295050272127047819 ) ) ;
#23579=CARTESIAN_POINT ( 'NONE',  ( 99.99999999999995737, 82.68750000136560629, 4.458734124999988779 ) ) ;
#23580=CARTESIAN_POINT ( 'NONE',  ( 78.57481594606305464, 39.90859375216787441, -1.662435489736055892E-15 ) ) ;
#23581=CARTESIAN_POINT ( 'NONE',  ( -20.00000000000000000, 55.00000000000000000, 10.00000000000000178 ) ) ;
#23583=CARTESIAN_POINT ( 'NONE',  ( 185.7049497278729575, 40.05742187608393579, 9.295050272127047819 ) ) ;
#23591=CARTESIAN_POINT ( 'NONE',  ( 124.5550856135277087, 36.93203125108394147, 13.14518615778179722 ) ) ;
#23592=CARTESIAN_POINT ( 'NONE',  ( 65.00000000000000000, 36.38632812608393152, -13.14518615778179544 ) ) ;
#23593=CARTESIAN_POINT ( 'NONE',  ( 208.1451861577817795, 40.40468750108393436, -5.444914386472297529 ) ) ;
#23595=CARTESIAN_POINT ( 'NONE',  ( 9.295050272127046043, 36.28710937608393294, -9.295050272127046043 ) ) ;
#23596=CARTESIAN_POINT ( 'NONE',  ( 129.5539587432196811, 49.99999999978092546, -13.57776691409254433 ) ) ;
#23599=CARTESIAN_POINT ( 'NONE',  ( 97.92893218813455292, 81.81250000000001421, -5.000000000000053291 ) ) ;
#23600=EDGE_CURVE ( 'NONE', #11913, #291, #11454, .T. ) ;
#23601=CARTESIAN_POINT ( 'NONE',  ( 13.14518615778179900, 40.10703125108393152, 5.444914386472293977 ) ) ;
#23605=VECTOR ( 'NONE', #2992, 1000.000000000000000 ) ;
#23606=CARTESIAN_POINT ( 'NONE',  ( 58.88224005446349452, 54.65941425414899868, 14.99999999999998401 ) ) ;
#23608=DIRECTION ( 'NONE',  ( 1.000000000000000000, 0.000000000000000000, 0.000000000000000000 ) ) ;
#23609=CIRCLE ( 'NONE', #17233, 13.57481594606304398 ) ;
#23612=VERTEX_POINT ( 'NONE', #2506 ) ;
#23618=CARTESIAN_POINT ( 'NONE',  ( 130.0000000000000000, 36.53515625216787299, 13.57481594606304576 ) ) ;
#23619=CARTESIAN_POINT ( 'NONE',  ( 96.84719886470459471, 83.81250000136560629, 3.152801135295355994 ) ) ;
#23620=CARTESIAN_POINT ( 'NONE',  ( 74.29505027212704249, 37.87460937608393863, 9.295050272127046043 ) ) ;
#23625=DIRECTION ( 'NONE',  ( 7.228014483236696740E-18, -0.000000000000000000, 1.000000000000000000 ) ) ;
#23627=CARTESIAN_POINT ( 'NONE',  ( 116.8548138422182063, 32.76484375108393010, -5.444914386472297529 ) ) ;
#23628=ORIENTED_EDGE ( 'NONE', *, *, #8973, .F. ) ;
#23629=DIRECTION ( 'NONE',  ( -0.000000000000000000, 1.000000000000000000, -0.000000000000000000 ) ) ;
#23631=CARTESIAN_POINT ( 'NONE',  ( 96.84719886470459471, 79.56250000136559208, 3.152801135295355994 ) ) ;
#23632=CARTESIAN_POINT ( 'NONE',  ( 143.1451861577818079, 35.34453125108392868, 5.444914386472293977 ) ) ;
#23633=CARTESIAN_POINT ( 'NONE',  ( 70.62287287157788285, 38.17226562716786731, 13.57481594606304576 ) ) ;
#23634=EDGE_CURVE ( 'NONE', #9074, #23612, #2744, .T. ) ;
#23636=CARTESIAN_POINT ( 'NONE',  ( 2.493653234604083739E-15, 35.74140625216787015, 13.57481594606304576 ) ) ;
#23639=ORIENTED_EDGE ( 'NONE', *, *, #20977, .F. ) ;
#23640=EDGE_CURVE ( 'NONE', #4741, #14316, #22030, .T. ) ;
#23641=CARTESIAN_POINT ( 'NONE',  ( 189.5550856135277229, 37.22968750108393721, -13.14518615778179900 ) ) ;
#23644=CARTESIAN_POINT ( 'NONE',  ( 120.7049497278729575, 39.66054687608393436, -9.295050272127046043 ) ) ;
#23647=CARTESIAN_POINT ( 'NONE',  ( 130.0000000000000000, 50.00000000000000000, -1.503427012513233026E-14 ) ) ;
#23651=CARTESIAN_POINT ( 'NONE',  ( 200.6228728715778686, 36.48554687499999716, 13.57481594606304576 ) ) ;
#23654=CARTESIAN_POINT ( 'NONE',  ( 74.29505027212704249, 37.67617187608393436, 9.295050272127046043 ) ) ;
#23658=AXIS2_PLACEMENT_3D ( 'NONE', #9567, #18553, #24963 ) ;
#23660=CARTESIAN_POINT ( 'NONE',  ( -5.622872871577873077, 37.97382812499999716, 13.57481594606304753 ) ) ;
#23663=CARTESIAN_POINT ( 'NONE',  ( 95.54126587499996504, 79.68750000136559208, -1.387778780781445676E-14 ) ) ;
#23668=CARTESIAN_POINT ( 'NONE',  ( 59.55508561352770158, 33.75703125108393721, 13.14518615778179722 ) ) ;
#23676=CARTESIAN_POINT ( 'NONE',  ( 195.0000000000000000, 37.32890625216786873, 13.57481594606304576 ) ) ;
#23678=DIRECTION ( 'NONE',  ( 1.000000000000000000, 0.000000000000000000, -2.385244779468110248E-16 ) ) ;
#23679=CARTESIAN_POINT ( 'NONE',  ( 195.0000000000000000, -7.395377635281828788, -13.57481594606306707 ) ) ;
#23680=CARTESIAN_POINT ( 'NONE',  ( 135.4449143864723339, 39.41250000108393436, 13.14518615778179189 ) ) ;
#23681=CARTESIAN_POINT ( 'NONE',  ( 5.444914386472302859, 37.03125000108393294, 13.14518615778179189 ) ) ;
#23682=AXIS2_PLACEMENT_3D ( 'NONE', #17048, #13032, #16782 ) ;
#23683=CARTESIAN_POINT ( 'NONE',  ( 124.5550856135277087, 33.55859375108393294, 13.14518615778179722 ) ) ;
#23684=CARTESIAN_POINT ( 'NONE',  ( 59.37712712842213136, 36.88242187499999858, -13.57481594606304753 ) ) ;
#23693=CARTESIAN_POINT ( 'NONE',  ( 2.414731522848535132E-15, 39.36289062608393152, 13.14518615778179544 ) ) ;
#23699=CARTESIAN_POINT ( 'NONE',  ( 181.4251840539369596, 36.28710937499999289, 5.622872871577880183 ) ) ;
#23700=CARTESIAN_POINT ( 'NONE',  ( 204.2950502721270425, 39.26367187608393294, 9.295050272127046043 ) ) ;
#23703=CARTESIAN_POINT ( 'NONE',  ( 214.9999999999999716, 55.00000000000000000, 9.999999999999946709 ) ) ;
#23704=CARTESIAN_POINT ( 'NONE',  ( 68.11659208046573610, 53.90895096933308395, -14.99999999999999822 ) ) ;
#23709=CARTESIAN_POINT ( 'NONE',  ( 120.4011555911795455, 35.44375000216787441, -9.598844408820458085 ) ) ;
#23714=CARTESIAN_POINT ( 'NONE',  ( 208.1451861577817795, 35.64218750108393152, -5.444914386472297529 ) ) ;
#23717=EDGE_LOOP ( 'NONE', ( #25627, #11522, #8968 ) ) ;
#23721=CARTESIAN_POINT ( 'NONE',  ( 65.00000000000000000, 40.35507812608393152, -13.14518615778179544 ) ) ;
#23722=CARTESIAN_POINT ( 'NONE',  ( 96.84719886470459471, 81.56250000136559208, 3.152801135295355994 ) ) ;
#23723=CARTESIAN_POINT ( 'NONE',  ( 189.5550856135277229, 40.40468750108393436, -13.14518615778179722 ) ) ;
#23724=CARTESIAN_POINT ( 'NONE',  ( 99.99999999999995737, 83.37500000273119838, 4.999999999999990230 ) ) ;
#23735=CARTESIAN_POINT ( 'NONE',  ( 139.2950502721270425, 37.08085937608393579, 9.295050272127046043 ) ) ;
#23736=CARTESIAN_POINT ( 'NONE',  ( 51.85481384221820633, 32.66562500108393863, 5.444914386472304635 ) ) ;
#23737=CARTESIAN_POINT ( 'NONE',  ( 185.7049497278729575, 36.88242187608393152, 9.295050272127047819 ) ) ;
#23739=CARTESIAN_POINT ( 'NONE',  ( 9.295050272127046043, 37.08085937608393579, -9.295050272127046043 ) ) ;
#23740=CARTESIAN_POINT ( 'NONE',  ( 139.1801758136479918, 50.00000000000000000, -10.00000000000000888 ) ) ;
#23741=CARTESIAN_POINT ( 'NONE',  ( 194.4067442974505866, 36.00000000000001421, 13.13889047851778180 ) ) ;
#23742=DIRECTION ( 'NONE',  ( 0.000000000000000000, 0.000000000000000000, -1.000000000000000000 ) ) ;
#23743=CARTESIAN_POINT ( 'NONE',  ( 9.295050272127047819, 38.46992187608393010, 9.295050272127046043 ) ) ;
#23745=DIRECTION ( 'NONE',  ( 0.000000000000000000, 0.000000000000000000, -1.000000000000000000 ) ) ;
#23748=CARTESIAN_POINT ( 'NONE',  ( 73.19315564490973713, 36.00000000000001421, 10.45682415286417921 ) ) ;
#23754=CARTESIAN_POINT ( 'NONE',  ( 0.000000000000000000, -7.395377635281828788, 0.000000000000000000 ) ) ;
#23755=CARTESIAN_POINT ( 'NONE',  ( 51.85481384221819923, 39.90859375108394147, -5.444914386472297529 ) ) ;
#23760=LINE ( 'NONE', #23900, #24975 ) ;
#23762=CARTESIAN_POINT ( 'NONE',  ( 135.6228728715778686, 39.95820312499999716, -13.57481594606304753 ) ) ;
#23763=ORIENTED_EDGE ( 'NONE', *, *, #17318, .T. ) ;
#23764=DIRECTION ( 'NONE',  ( -1.000000000000000000, -0.000000000000000000, 2.385244779468110248E-16 ) ) ;
#23768=CARTESIAN_POINT ( 'NONE',  ( 143.1451861577818079, 35.44375000108393436, -5.444914386472297529 ) ) ;
#23769=CARTESIAN_POINT ( 'NONE',  ( 70.62287287157788285, 35.79101562716787299, 13.57481594606304576 ) ) ;
#23771=CARTESIAN_POINT ( 'NONE',  ( 5.622872871577878406, 36.58476562716787583, 13.57481594606304576 ) ) ;
#23775=CARTESIAN_POINT ( 'NONE',  ( 181.8548138422181921, 38.12265625108393152, -5.444914386472297529 ) ) ;
#23776=CARTESIAN_POINT ( 'NONE',  ( 104.9999999999999716, 81.43750000000002842, 2.071067811865462627 ) ) ;
#23779=CARTESIAN_POINT ( 'NONE',  ( 128.3947281234234197, 53.60388944777321996, 14.99999999999996803 ) ) ;
#23781=( BOUNDED_CURVE ( )  B_SPLINE_CURVE ( 2, ( #24886, #18037, #24457, #14032, #13606, #11888, #20613, #22328, #2799 ),
 .UNSPECIFIED., .F., .F. ) 
 B_SPLINE_CURVE_WITH_KNOTS ( ( 3, 2, 2, 2, 3 ),
 ( 0.2708333333333330928, 0.2812499999999998890, 0.2916666666666666852, 0.3020833333333334259, 0.3125000000000002220 ),
 .UNSPECIFIED. ) 
 CURVE ( )  GEOMETRIC_REPRESENTATION_ITEM ( )  RATIONAL_B_SPLINE_CURVE ( ( 1.000000000000001554, 0.9238795325112850731, 1.000000000000000000, 0.9238795325112867385, 1.000000000000000000, 0.9238795325112867385, 1.000000000000000000, 0.9238795325112850731, 1.000000000000001554 ) ) 
 REPRESENTATION_ITEM ( '' )  );
#23782=CARTESIAN_POINT ( 'NONE',  ( 130.0000000000000000, -7.395377635281828788, 13.57481594606302799 ) ) ;
#23785=CARTESIAN_POINT ( 'NONE',  ( 204.5988444088204403, 34.35234374999999574, -9.598844408820458085 ) ) ;
#23786=ADVANCED_FACE ( 'NONE', ( #657 ), #13876, .T. ) ;
#23789=CARTESIAN_POINT ( 'NONE',  ( 78.14518615778179367, 39.41250000108393436, -5.444914386472297529 ) ) ;
#23791=DIRECTION ( 'NONE',  ( 0.000000000000000000, 0.000000000000000000, 1.000000000000000000 ) ) ;
#23794=CARTESIAN_POINT ( 'NONE',  ( 2.493653234604083739E-15, 34.84843749999999574, 13.57481594606304576 ) ) ;
#23797=CARTESIAN_POINT ( 'NONE',  ( 98.15313185440925281, 80.87500000136560629, 4.458734124999987891 ) ) ;
#23800=ADVANCED_FACE ( 'NONE', ( #22316 ), #21021, .T. ) ;
#23801=VECTOR ( 'NONE', #16289, 1000.000000000000000 ) ;
#23803=CARTESIAN_POINT ( 'NONE',  ( 78.14518615778179367, 35.59257812608393579, -1.609821015232357215E-15 ) ) ;
#23805=CARTESIAN_POINT ( 'NONE',  ( 137.6239419619254534, 54.99999999999999289, -14.99999999999999822 ) ) ;
#23807=ORIENTED_EDGE ( 'NONE', *, *, #2897, .T. ) ;
#23811=CARTESIAN_POINT ( 'NONE',  ( 208.5748159460630120, 39.16445312716788152, -5.622872871577873077 ) ) ;
#23813=CARTESIAN_POINT ( 'NONE',  ( 76.10484805054758795, 36.02027164848242791, -8.092840767093349541 ) ) ;
#23814=CARTESIAN_POINT ( 'NONE',  ( 99.99999999999995737, 85.00000000000000000, 4.999999999999990230 ) ) ;
#23815=CARTESIAN_POINT ( 'NONE',  ( 117.3184072029388290, 36.04503594658365984, 5.908507747192915716 ) ) ;
#23817=CARTESIAN_POINT ( 'NONE',  ( -9.295050272127044266, 36.88242187608393152, 9.295050272127047819 ) ) ;
#23818=CARTESIAN_POINT ( 'NONE',  ( 130.0000000000000000, 33.60820312608392868, 13.14518615778179544 ) ) ;
#23819=CARTESIAN_POINT ( 'NONE',  ( 55.40115559117954547, 33.16171874999999858, 9.598844408820459861 ) ) ;
#23827=DIRECTION ( 'NONE',  ( 1.000000000000000000, 0.000000000000000000, -0.000000000000000000 ) ) ;
#23829=CARTESIAN_POINT ( 'NONE',  ( 13.14518615778179900, 38.71796875108393721, 5.444914386472293977 ) ) ;
#23835=CARTESIAN_POINT ( 'NONE',  ( 130.0000000000000000, -7.395377635281828788, 13.57481594606302799 ) ) ;
#23836=( BOUNDED_CURVE ( )  B_SPLINE_CURVE ( 2, ( #8861, #15113, #4314, #21704, #4592, #19555, #8719, #15547, #17412 ),
 .UNSPECIFIED., .F., .T. ) 
 B_SPLINE_CURVE_WITH_KNOTS ( ( 3, 2, 2, 2, 3 ),
 ( 0.3125000000000002220, 0.3229166666666668517, 0.3333333333333334259, 0.3437500000000000555, 0.3541666666666666852 ),
 .UNSPECIFIED. ) 
 CURVE ( )  GEOMETRIC_REPRESENTATION_ITEM ( )  RATIONAL_B_SPLINE_CURVE ( ( 0.9999999999999983347, 0.9238795325112884038, 1.000000000000000000, 0.9238795325112867385, 1.000000000000000000, 0.9238795325112867385, 1.000000000000000000, 0.9238795325112867385, 1.000000000000000000 ) ) 
 REPRESENTATION_ITEM ( '' )  );
#23837=CARTESIAN_POINT ( 'NONE',  ( 189.5550856135277229, 39.90859375108393436, 13.14518615778179722 ) ) ;
#23838=EDGE_LOOP ( 'NONE', ( #13294, #27094, #5454, #3929 ) ) ;
#23840=DIRECTION ( 'NONE',  ( 1.000000000000000000, 0.000000000000000000, 0.000000000000000000 ) ) ;
#23841=CARTESIAN_POINT ( 'NONE',  ( 61.20254813104200764, 54.08938259242988522, -15.00000000000000355 ) ) ;
#23843=ORIENTED_EDGE ( 'NONE', *, *, #23286, .T. ) ;
#23847=CARTESIAN_POINT ( 'NONE',  ( 139.2950502721270425, 39.46210937608393010, -9.295050272127046043 ) ) ;
#23851=CARTESIAN_POINT ( 'NONE',  ( 185.7049497278729575, 35.89023437608393152, -9.295050272127046043 ) ) ;
#23852=ORIENTED_EDGE ( 'NONE', *, *, #10719, .F. ) ;
#23857=CARTESIAN_POINT ( 'NONE',  ( 94.99999999999995737, 80.00000000000000000, -1.387778780781445676E-14 ) ) ;
#23858=CARTESIAN_POINT ( 'NONE',  ( 95.54126587499996504, 81.37500000136563472, -1.846868145590750077 ) ) ;
#23859=CARTESIAN_POINT ( 'NONE',  ( 208.1451861577818079, 39.41250000108393436, -5.444914386472297529 ) ) ;
#23861=CARTESIAN_POINT ( 'NONE',  ( 130.0000000000000000, 50.00000000000000000, -1.503427012513233026E-14 ) ) ;
#23863=CARTESIAN_POINT ( 'NONE',  ( 189.5550856135277229, 40.60312500108393863, -13.14518615778179722 ) ) ;
#23869=( BOUNDED_CURVE ( )  B_SPLINE_CURVE ( 2, ( #1235, #9899, #14588, #21304, #27316, #1786, #10453, #19159, #12306, #27863, #16460, #25154, #18611, #17008, #8323, #16602, #25712, #3501, #18746, #27446, #25294, #5783, #3642, #21028, #1511, #2206, #347, #28001, #23579, #8745, #10869, #24003, #17436, #25855, #26283, #8887, #4480, #21585, #26428, #15285, #6888, #15140, #6326, #4197, #15428, #21872, #23722, #26135, #21732, #23858, #17153, #6601, #11005, #13136, #15000, #2349, #12856, #19302, #17293, #4060, #12722, #8465, #2061, #10731, #6743, #19579, #11144, #1926, #63, #202, #19717, #12992, #24142, #17577, #4619, #13277, #22007, #19440, #2484, #21448, #6466 ),
 .UNSPECIFIED., .F., .F. ) 
 B_SPLINE_CURVE_WITH_KNOTS ( ( 3, 2, 2, 2, 2, 2, 2, 2, 2, 2, 2, 2, 2, 2, 2, 2, 2, 2, 2, 2, 2, 2, 2, 2, 2, 2, 2, 2, 2, 2, 2, 2, 2, 2, 2, 2, 2, 2, 2, 2, 3 ),
 ( 0.000000000000000000, 0.02500000000000000139, 0.05000000000000000278, 0.07499999999999999722, 0.1000000000000000056, 0.1250000000000000000, 0.1499999999999999944, 0.1749999999999999889, 0.2000000000000000111, 0.2250000000000000056, 0.2500000000000000000, 0.2750000000000000222, 0.2999999999999999889, 0.3250000000000000111, 0.3499999999999999778, 0.3750000000000000000, 0.4000000000000000222, 0.4249999999999999889, 0.4500000000000000111, 0.4749999999999999778, 0.5000000000000000000, 0.5250000000000000222, 0.5500000000000000444, 0.5749999999999999556, 0.5999999999999999778, 0.6250000000000000000, 0.6500000000000000222, 0.6750000000000000444, 0.6999999999999999556, 0.7249999999999999778, 0.7500000000000000000, 0.7750000000000000222, 0.8000000000000000444, 0.8249999999999999556, 0.8499999999999999778, 0.8750000000000000000, 0.9000000000000000222, 0.9250000000000000444, 0.9499999999999999556, 0.9749999999999999778, 1.000000000000000000 ),
 .UNSPECIFIED. ) 
 CURVE ( )  GEOMETRIC_REPRESENTATION_ITEM ( )  RATIONAL_B_SPLINE_CURVE ( ( 1.000000000000000000, 0.9238795325112867385, 1.000000000000000000, 0.9238795325112867385, 1.000000000000000000, 0.9238795325112867385, 1.000000000000000000, 0.9238795325112867385, 1.000000000000000000, 0.9238795325112867385, 1.000000000000000000, 0.9238795325112867385, 1.000000000000000000, 0.9238795325112867385, 1.000000000000000000, 0.9238795325112867385, 1.000000000000000000, 0.9238795325112867385, 1.000000000000000000, 0.9238795325112867385, 1.000000000000000000, 0.9238795325112867385, 1.000000000000000000, 0.9238795325112867385, 1.000000000000000000, 0.9238795325112867385, 1.000000000000000000, 0.9238795325112867385, 1.000000000000000000, 0.9238795325112867385, 1.000000000000000000, 0.9238795325112867385, 1.000000000000000000, 0.9238795325112867385, 1.000000000000000000, 0.9238795325112867385, 1.000000000000000000, 0.9238795325112867385, 1.000000000000000000, 0.9238795325112867385, 1.000000000000000000, 0.9238795325112867385, 1.000000000000000000, 0.9238795325112867385, 1.000000000000000000, 0.9238795325112867385, 1.000000000000000000, 0.9238795325112867385, 1.000000000000000000, 0.9238795325112867385, 1.000000000000000000, 0.9238795325112867385, 1.000000000000000000, 0.9238795325112867385, 1.000000000000000000, 0.9238795325112867385, 1.000000000000000000, 0.9238795325112867385, 1.000000000000000000, 0.9238795325112867385, 1.000000000000000000, 0.9238795325112867385, 1.000000000000000000, 0.9238795325112867385, 1.000000000000000000, 0.9238795325112867385, 1.000000000000000000, 0.9238795325112867385, 1.000000000000000000, 0.9238795325112867385, 1.000000000000000000, 0.9238795325112867385, 1.000000000000000000, 0.9238795325112867385, 1.000000000000000000, 0.9238795325112867385, 1.000000000000000000, 0.9238795325112867385, 1.000000000000000000, 0.9238795325112867385, 1.000000000000000000 ) ) 
 REPRESENTATION_ITEM ( '' )  );
#23871=CARTESIAN_POINT ( 'NONE',  ( 124.5550856135277087, 37.42812500108394147, -13.14518615778179900 ) ) ;
#23872=CARTESIAN_POINT ( 'NONE',  ( 78.14518615778179367, 32.26875000108393721, -5.444914386472297529 ) ) ;
#23873=CARTESIAN_POINT ( 'NONE',  ( 208.1451861577818079, 38.76757812608393294, -1.609821015232357215E-15 ) ) ;
#23875=CARTESIAN_POINT ( 'NONE',  ( -9.295050272127046043, 32.51679687608393721, -9.295050272127046043 ) ) ;
#23876=CARTESIAN_POINT ( 'NONE',  ( 138.7583343923579093, 50.00000000000000000, -10.38725784494287296 ) ) ;
#23878=SPHERICAL_SURFACE ( 'NONE', #10852, 5.000000000000000000 ) ;
#23880=EDGE_CURVE ( 'NONE', #24292, #15436, #17116, .T. ) ;
#23881=CARTESIAN_POINT ( 'NONE',  ( 9.295050272127047819, 36.08867187608392868, 9.295050272127046043 ) ) ;
#23882=CARTESIAN_POINT ( 'NONE',  ( -15.00000000000000355, 80.00000000000000000, -14.99999999999999822 ) ) ;
#23883=CARTESIAN_POINT ( 'NONE',  ( 104.9999999999999716, 79.56250000273118417, 2.071067811865462627 ) ) ;
#23891=CARTESIAN_POINT ( 'NONE',  ( 125.9374164594230763, 50.00000000116060761, 12.98908657125170940 ) ) ;
#23893=FACE_OUTER_BOUND ( 'NONE', #23161, .T. ) ;
#23894=CARTESIAN_POINT ( 'NONE',  ( 99.99999999999995737, 81.43750000136559208, -4.458734125000016313 ) ) ;
#23895=CARTESIAN_POINT ( 'NONE',  ( 78.14518615778179367, 34.79882812608394005, -1.609821015232357215E-15 ) ) ;
#23899=FACE_OUTER_BOUND ( 'NONE', #24126, .T. ) ;
#23900=CARTESIAN_POINT ( 'NONE',  ( 99.99999999999995737, 85.00000000000000000, -3.000000000000018208 ) ) ;
#23901=CARTESIAN_POINT ( 'NONE',  ( 135.6228728715778971, 38.86679687499999858, 13.57481594606304576 ) ) ;
#23906=CARTESIAN_POINT ( 'NONE',  ( 124.5550856135277087, 38.02343750108394005, -13.14518615778179900 ) ) ;
#23907=CARTESIAN_POINT ( 'NONE',  ( 65.00000000000000000, 34.15390625216787157, 13.57481594606304576 ) ) ;
#23910=CARTESIAN_POINT ( 'NONE',  ( -8.312177448680279460E-16, 32.16953125216787157, -13.57481594606304576 ) ) ;
#23914=CARTESIAN_POINT ( 'NONE',  ( 181.8548138422181921, 34.25312500108393010, 5.444914386472304635 ) ) ;
#23915=AXIS2_PLACEMENT_3D ( 'NONE', #13116, #27847, #12460 ) ;
#23916=AXIS2_PLACEMENT_3D ( 'NONE', #23934, #278, #19794 ) ;
#23917=CARTESIAN_POINT ( 'NONE',  ( -20.00000000000000000, 50.00000000000000000, 10.00000000000000178 ) ) ;
#23918=CARTESIAN_POINT ( 'NONE',  ( 102.0710678118654755, 81.68750000000001421, -4.999999999999983125 ) ) ;
#23922=CARTESIAN_POINT ( 'NONE',  ( 208.5748159460630688, 36.63437499999999858, -1.662435489736055892E-15 ) ) ;
#23924=CARTESIAN_POINT ( 'NONE',  ( 65.00000000000000000, -7.395377635281828788, -13.57481594606305109 ) ) ;
#23927=CARTESIAN_POINT ( 'NONE',  ( 200.6228728715778686, 34.10429687499999574, 13.57481594606304576 ) ) ;
#23930=CARTESIAN_POINT ( 'NONE',  ( 51.85481384221820633, 36.58476562608393579, 0.000000000000000000 ) ) ;
#23931=DIRECTION ( 'NONE',  ( 0.000000000000000000, 1.000000000000000000, 0.000000000000000000 ) ) ;
#23932=FACE_BOUND ( 'NONE', #8599, .T. ) ;
#23934=CARTESIAN_POINT ( 'NONE',  ( 65.00000000000000000, 50.00000000000000000, -7.517135062566165128E-15 ) ) ;
#23935=CARTESIAN_POINT ( 'NONE',  ( 13.57481594606304753, 37.47773437500001137, -5.622872871577873077 ) ) ;
#23936=ORIENTED_EDGE ( 'NONE', *, *, #19570, .T. ) ;
#23938=CARTESIAN_POINT ( 'NONE',  ( 104.9999999999999574, 83.43750000000001421, 2.071067811865462627 ) ) ;
#23942=ORIENTED_EDGE ( 'NONE', *, *, #21918, .T. ) ;
#23945=CARTESIAN_POINT ( 'NONE',  ( 70.44491438647230552, 34.65000000108393863, 13.14518615778179189 ) ) ;
#23947=CARTESIAN_POINT ( 'NONE',  ( 143.5748159460630688, 39.11484375216787157, -1.662435489736055892E-15 ) ) ;
#23952=CARTESIAN_POINT ( 'NONE',  ( 204.5988444088204687, 39.01562500216787299, 9.598844408820456309 ) ) ;
#23954=EDGE_CURVE ( 'NONE', #17777, #15111, #23019, .T. ) ;
#23957=CARTESIAN_POINT ( 'NONE',  ( 135.4449143864723339, 37.03125000108393294, 13.14518615778179189 ) ) ;
#23959=CARTESIAN_POINT ( 'NONE',  ( -13.14518615778179900, 38.32109375108394289, -5.444914386472297529 ) ) ;
#23960=CARTESIAN_POINT ( 'NONE',  ( 135.4449143864723055, 34.74921875108394431, -13.14518615778179900 ) ) ;
#23961=CARTESIAN_POINT ( 'NONE',  ( 55.40115559117954547, 33.75703124999999005, -9.598844408820458085 ) ) ;
#23969=CARTESIAN_POINT ( 'NONE',  ( 98.15313185440923860, 80.50000000136560629, -4.458734125000016313 ) ) ;
#23971=CARTESIAN_POINT ( 'NONE',  ( 9.295050272127047819, 37.87460937608393863, 9.295050272127046043 ) ) ;
#23974=ORIENTED_EDGE ( 'NONE', *, *, #7379, .F. ) ;
#23976=AXIS2_PLACEMENT_3D ( 'NONE', #15212, #23931, #2280 ) ;
#23977=CARTESIAN_POINT ( 'NONE',  ( 97.92893218813456713, 79.93750000273118417, -5.000000000000067502 ) ) ;
#23979=CARTESIAN_POINT ( 'NONE',  ( 195.0000000000000000, 40.35507812608393152, -13.14518615778179544 ) ) ;
#23981=CARTESIAN_POINT ( 'NONE',  ( 78.14518615778180788, 36.43593750108394147, -5.444914386472297529 ) ) ;
#23984=ORIENTED_EDGE ( 'NONE', *, *, #5147, .F. ) ;
#23988=CARTESIAN_POINT ( 'NONE',  ( 116.8548138422182063, 39.80937500108392868, 5.444914386472304635 ) ) ;
#23989=CARTESIAN_POINT ( 'NONE',  ( 5.444914386472302859, 40.20625000108394431, 13.14518615778179189 ) ) ;
#23992=CARTESIAN_POINT ( 'NONE',  ( 65.00000000000000000, 37.77539062608393294, 13.14518615778179544 ) ) ;
#23996=CARTESIAN_POINT ( 'NONE',  ( 195.0000000000000000, 36.18789062608393436, 13.14518615778179544 ) ) ;
#23999=VERTEX_POINT ( 'NONE', #14020 ) ;
#24002=CARTESIAN_POINT ( 'NONE',  ( 74.29505027212704249, 40.05742187608392868, 9.295050272127046043 ) ) ;
#24003=CARTESIAN_POINT ( 'NONE',  ( 95.54126587499996504, 82.50000000136560629, 1.846868145590724986 ) ) ;
#24004=CARTESIAN_POINT ( 'NONE',  ( 195.0000000000000000, 40.35507812608393152, -13.14518615778179544 ) ) ;
#24006=CARTESIAN_POINT ( 'NONE',  ( 188.8389378251398796, 51.27996893916986210, 14.99999999999857891 ) ) ;
#24007=DIRECTION ( 'NONE',  ( 0.000000000000000000, 0.000000000000000000, 1.000000000000000000 ) ) ;
#24008=CARTESIAN_POINT ( 'NONE',  ( 208.1451861577818079, 40.35507812608393863, -1.609821015232357215E-15 ) ) ;
#24010=ORIENTED_EDGE ( 'NONE', *, *, #9714, .T. ) ;
#24014=CARTESIAN_POINT ( 'NONE',  ( 143.1451861577818079, 36.38632812608393863, -1.609821015232357215E-15 ) ) ;
#24015=CARTESIAN_POINT ( 'NONE',  ( 70.44491438647230552, 35.24531250108393010, 13.14518615778179189 ) ) ;
#24016=CARTESIAN_POINT ( 'NONE',  ( 185.7049497278729575, 35.89023437608393152, -9.295050272127046043 ) ) ;
#24020=CARTESIAN_POINT ( 'NONE',  ( 136.4508793426651607, 50.00000000106927445, -11.97362904075493084 ) ) ;
#24021=CARTESIAN_POINT ( 'NONE',  ( -18.00000000000000355, 80.00000000000000000, 15.00000000000000178 ) ) ;
#24022=CARTESIAN_POINT ( 'NONE',  ( -20.00000000000000355, 55.00000000000000000, -14.99999999999999822 ) ) ;
#24024=CARTESIAN_POINT ( 'NONE',  ( -13.14518615778179189, 36.63437500108393152, 5.444914386472304635 ) ) ;
#24025=CARTESIAN_POINT ( 'NONE',  ( -9.180175813647995398, 55.00000000000000000, 15.00000000000000000 ) ) ;
#24026=CARTESIAN_POINT ( 'NONE',  ( 102.0710678118653760, 79.43750000273119838, 5.000000000000054179 ) ) ;
#24027=CARTESIAN_POINT ( 'NONE',  ( 55.81982418635200816, 50.00000000000000000, 9.999999999999984013 ) ) ;
#24028=DIRECTION ( 'NONE',  ( 0.000000000000000000, 0.000000000000000000, 1.000000000000000000 ) ) ;
#24032=CARTESIAN_POINT ( 'NONE',  ( 130.8765262653674881, 51.45968077934806217, 14.99999999999996625 ) ) ;
#24034=CARTESIAN_POINT ( 'NONE',  ( 124.3771271284221740, 38.56914062716787583, -13.57481594606310260 ) ) ;
#24035=DIRECTION ( 'NONE',  ( 0.000000000000000000, 0.000000000000000000, 1.000000000000000000 ) ) ;
#24036=CARTESIAN_POINT ( 'NONE',  ( 78.14518615778179367, 35.59257812608393579, -1.609821015232357215E-15 ) ) ;
#24038=CARTESIAN_POINT ( 'NONE',  ( 5.444914386472297529, 37.92421875108393436, -13.14518615778179722 ) ) ;
#24042=CARTESIAN_POINT ( 'NONE',  ( 116.4251840539369738, 36.28710937499999289, 5.622872871577880183 ) ) ;
#24043=CARTESIAN_POINT ( 'NONE',  ( 99.99999999999995737, 82.75000000000000000, -5.000000000000018652 ) ) ;
#24044=CARTESIAN_POINT ( 'NONE',  ( 139.5988444088204687, 36.53515624999999289, 9.598844408820456309 ) ) ;
#24046=DIRECTION ( 'NONE',  ( 0.000000000000000000, -1.000000000000000000, 0.000000000000000000 ) ) ;
#24047=EDGE_CURVE ( 'NONE', #26226, #15733, #3770, .T. ) ;
#24050=CARTESIAN_POINT ( 'NONE',  ( 120.7049497278729575, 36.48554687608393721, -9.295050272127046043 ) ) ;
#24051=CARTESIAN_POINT ( 'NONE',  ( 74.59884440882045453, 32.66562500216787157, 9.598844408820456309 ) ) ;
#24053=CARTESIAN_POINT ( 'NONE',  ( -13.57481594606304753, 33.90585937716787868, -5.622872871577873077 ) ) ;
#24057=CARTESIAN_POINT ( 'NONE',  ( 204.2950502721270425, 33.90585937608393152, -9.295050272127046043 ) ) ;
#24059=FACE_OUTER_BOUND ( 'NONE', #9073, .T. ) ;
#24061=CARTESIAN_POINT ( 'NONE',  ( 65.00000000000000000, 37.32890625216786873, 13.57481594606304576 ) ) ;
#24062=CARTESIAN_POINT ( 'NONE',  ( 133.7974518689580350, 54.08938259242986391, 14.99999999999996447 ) ) ;
#24068=CARTESIAN_POINT ( 'NONE',  ( 181.4251840539369596, 35.49335937499999005, 5.622872871577880183 ) ) ;
#24071=CARTESIAN_POINT ( 'NONE',  ( 55.70494972787295751, 34.10429687608393579, -9.295050272127046043 ) ) ;
#24075=CARTESIAN_POINT ( 'NONE',  ( -13.57481594606304576, 37.82499999999999574, 0.000000000000000000 ) ) ;
#24076=CARTESIAN_POINT ( 'NONE',  ( 143.1451861577818079, 36.38632812608393863, -1.609821015232357215E-15 ) ) ;
#24077=VERTEX_POINT ( 'NONE', #9614 ) ;
#24078=CARTESIAN_POINT ( 'NONE',  ( 94.99999999999995737, 84.06250000000000000, 2.071067811865466624 ) ) ;
#24079=EDGE_CURVE ( 'NONE', #19393, #16078, #26539, .T. ) ;
#24080=AXIS2_PLACEMENT_3D ( 'NONE', #19502, #15346, #3984 ) ;
#24081=CARTESIAN_POINT ( 'NONE',  ( 104.9999999999999574, 80.68750000273119838, -2.071067811865491937 ) ) ;
#24083=CARTESIAN_POINT ( 'NONE',  ( 53.30962175448677698, 35.99999999999999289, -6.307928093363390332 ) ) ;
#24084=B_SPLINE_CURVE_WITH_KNOTS ( 'NONE', 3,
 ( #12337, #26922, #27479, #13915, #1401, #18639, #5250, #27343, #22642, #16207, #3110, #23056, #14338, #3382, #12053, #24911, #842, #11779, #985, #1125, #12190, #20779, #5394, #18213, #3533, #1261, #14063, #9923, #20919, #3675, #7802 ),
 .UNSPECIFIED., .F., .F.,
 ( 4, 2, 2, 2, 2, 2, 2, 2, 2, 2, 1, 2, 2, 2, 2, 4 ),
 ( 1.261830988103825351E-15, 0.001656255954915028267, 0.003312511909828794957, 0.004968767864742561213, 0.005796895842199402925, 0.006625023819656245504, 0.008281279774569928059, 0.009937535729483611482, 0.01325004763931101823, 0.01490630359422470512, 0.01656255954913839548, 0.01821881550405208064, 0.01987507145896576580, 0.02318758336879312223, 0.02484383932370680045, 0.02650009527862047173 ),
 .UNSPECIFIED. ) ;
#24085=( BOUNDED_CURVE ( )  B_SPLINE_CURVE ( 2, ( #19567, #17425, #9161, #4604, #17991, #26416, #26701, #10993, #24555, #191, #13263, #23989, #5036, #13125, #26123, #17714, #15559, #6589, #2615, #21860, #2335, #19706, #8873, #22137, #11278, #17853, #478, #26556, #9436, #3457, #20427, #26849, #3318, #15985, #7586, #9581, #7728, #9863, #16419, #14269, #25116, #11849, #9724, #5603, #16279, #20571, #12123, #911, #20276, #1052, #27134, #3179, #5742, #11989, #26991, #20849, #18285, #1329, #7867, #13981, #24699, #763, #7436, #24978, #5461, #9995, #11702, #22988, #18703, #16131, #14130, #22419, #18136, #27406, #7296, #16561, #20713, #5177, #1195, #13841, #24839, #22709, #25252, #22566, #3033, #2890, #11560, #5322, #27273, #18426, #22851, #18570, #12535, #10264, #23127, #27958, #10410 ),
 .UNSPECIFIED., .F., .F. ) 
 B_SPLINE_CURVE_WITH_KNOTS ( ( 3, 2, 2, 2, 2, 2, 2, 2, 2, 2, 2, 2, 2, 2, 2, 2, 2, 2, 2, 2, 2, 2, 2, 2, 2, 2, 2, 2, 2, 2, 2, 2, 2, 2, 2, 2, 2, 2, 2, 2, 2, 2, 2, 2, 2, 2, 2, 2, 3 ),
 ( 0.000000000000000000, 0.01041666666666666609, 0.02083333333333333218, 0.03125000000000000000, 0.04166666666666666435, 0.05208333333333333565, 0.06250000000000000000, 0.07291666666666667129, 0.08333333333333332871, 0.09374999999999998612, 0.1041666666666666713, 0.1145833333333333287, 0.1250000000000000000, 0.1354166666666666574, 0.1458333333333333426, 0.1562500000000000000, 0.1666666666666666574, 0.1770833333333333426, 0.1874999999999999722, 0.1979166666666666574, 0.2083333333333333426, 0.2187500000000000000, 0.2291666666666666574, 0.2395833333333333426, 0.2500000000000000000, 0.2604166666666666852, 0.2708333333333333148, 0.2812500000000000000, 0.2916666666666666852, 0.3020833333333333148, 0.3125000000000000000, 0.3229166666666666852, 0.3333333333333333148, 0.3437500000000000000, 0.3541666666666666852, 0.3645833333333333148, 0.3749999999999999445, 0.3854166666666666852, 0.3958333333333333148, 0.4062500000000000000, 0.4166666666666666852, 0.4270833333333333148, 0.4375000000000000000, 0.4479166666666666852, 0.4583333333333333148, 0.4687500000000000000, 0.4791666666666666852, 0.4895833333333333148, 0.4988304892921909817 ),
 .UNSPECIFIED. ) 
 CURVE ( )  GEOMETRIC_REPRESENTATION_ITEM ( )  RATIONAL_B_SPLINE_CURVE ( ( 1.000000000000000000, 0.9238795325112867385, 1.000000000000000000, 0.9238795325112867385, 1.000000000000000000, 0.9238795325112867385, 1.000000000000000000, 0.9238795325112867385, 1.000000000000000000, 0.9238795325112867385, 1.000000000000000000, 0.9238795325112867385, 1.000000000000000000, 0.9238795325112867385, 1.000000000000000000, 0.9238795325112867385, 1.000000000000000000, 0.9238795325112867385, 1.000000000000000000, 0.9238795325112867385, 1.000000000000000000, 0.9238795325112867385, 1.000000000000000000, 0.9238795325112867385, 1.000000000000000000, 0.9238795325112867385, 1.000000000000000000, 0.9238795325112867385, 1.000000000000000000, 0.9238795325112867385, 1.000000000000000000, 0.9238795325112867385, 1.000000000000000000, 0.9238795325112867385, 1.000000000000000000, 0.9238795325112867385, 1.000000000000000000, 0.9238795325112867385, 1.000000000000000000, 0.9238795325112867385, 1.000000000000000000, 0.9238795325112867385, 1.000000000000000000, 0.9238795325112867385, 1.000000000000000000, 0.9238795325112867385, 1.000000000000000000, 0.9238795325112867385, 1.000000000000000000, 0.9238795325112867385, 1.000000000000000000, 0.9238795325112867385, 1.000000000000000000, 0.9238795325112867385, 1.000000000000000000, 0.9238795325112867385, 1.000000000000000000, 0.9238795325112867385, 1.000000000000000000, 0.9238795325112867385, 1.000000000000000000, 0.9238795325112867385, 1.000000000000000000, 0.9238795325112867385, 1.000000000000000000, 0.9238795325112867385, 1.000000000000000000, 0.9238795325112867385, 1.000000000000000000, 0.9238795325112867385, 1.000000000000000000, 0.9238795325112867385, 1.000000000000000000, 0.9238795325112867385, 1.000000000000000000, 0.9238795325112867385, 1.000000000000000000, 0.9238795325112867385, 1.000000000000000000, 0.9238795325112867385, 1.000000000000000000, 0.9238795325112867385, 1.000000000000000000, 0.9238795325112867385, 1.000000000000000000, 0.9238795325112867385, 1.000000000000000000, 0.9238795325112867385, 1.000000000000000000, 0.9238795325112867385, 1.000000000000000000, 0.9238795325112867385, 1.000000000000000000, 0.9238795325112867385, 1.000000000000000000, 0.9324258078851886955, 0.9848264816800353927 ) ) 
 REPRESENTATION_ITEM ( '' )  );
#24087=CARTESIAN_POINT ( 'NONE',  ( 51.85481384221820633, 34.45156250108394147, 5.444914386472304635 ) ) ;
#24088=ORIENTED_EDGE ( 'NONE', *, *, #19982, .T. ) ;
#24091=ORIENTED_EDGE ( 'NONE', *, *, #24711, .F. ) ;
#24092=DIRECTION ( 'NONE',  ( 0.000000000000000000, -1.000000000000000000, 0.000000000000000000 ) ) ;
#24094=CARTESIAN_POINT ( 'NONE',  ( 189.3771271284221314, 34.10429687716786873, 13.57481594606304753 ) ) ;
#24097=CARTESIAN_POINT ( 'NONE',  ( 130.0000000000000000, 36.18789062608393436, 13.14518615778179544 ) ) ;
#24098=CARTESIAN_POINT ( 'NONE',  ( 5.444914386472297529, 39.71015625108393010, -13.14518615778179900 ) ) ;
#24099=CARTESIAN_POINT ( 'NONE',  ( 124.5550856135277087, 34.05468750108393294, -13.14518615778179900 ) ) ;
#24100=CARTESIAN_POINT ( 'NONE',  ( 70.62287287157788285, 35.69179687499999432, 13.57481594606304576 ) ) ;
#24103=CARTESIAN_POINT ( 'NONE',  ( 181.4251840539369596, 37.08085937499999574, 5.622872871577880183 ) ) ;
#24107=CARTESIAN_POINT ( 'NONE',  ( 5.622872871577742515, 38.96601562716787015, 13.57481594606318076 ) ) ;
#24110=CARTESIAN_POINT ( 'NONE',  ( -9.295050272127046043, 36.68398437608393436, -9.295050272127046043 ) ) ;
#24111=VECTOR ( 'NONE', #26273, 1000.000000000000000 ) ;
#24113=VERTEX_POINT ( 'NONE', #6051 ) ;
#24116=EDGE_CURVE ( 'NONE', #18823, #13418, #25868, .T. ) ;
#24117=CARTESIAN_POINT ( 'NONE',  ( 214.9999999999999716, 55.00000000000000000, 14.99999999999994493 ) ) ;
#24118=EDGE_CURVE ( 'NONE', #19624, #2438, #23339, .T. ) ;
#24119=CARTESIAN_POINT ( 'NONE',  ( 181.8548138422181921, 39.80937500108392868, 5.444914386472304635 ) ) ;
#24120=( BOUNDED_CURVE ( )  B_SPLINE_CURVE ( 2, ( #11672, #587, #17676, #22107, #15816 ),
 .UNSPECIFIED., .F., .F. ) 
 B_SPLINE_CURVE_WITH_KNOTS ( ( 3, 2, 3 ),
 ( 0.4375000000000003331, 0.4479166666666667962, 0.4520580917964571177 ),
 .UNSPECIFIED. ) 
 CURVE ( )  GEOMETRIC_REPRESENTATION_ITEM ( )  RATIONAL_B_SPLINE_CURVE ( ( 0.9999999999999975575, 0.9238795325112891810, 1.000000000000000000, 0.9697362671728813055, 0.9635368512068493985 ) ) 
 REPRESENTATION_ITEM ( '' )  );
#24124=FACE_OUTER_BOUND ( 'NONE', #8432, .T. ) ;
#24126=EDGE_LOOP ( 'NONE', ( #3520, #5075, #2463, #12863 ) ) ;
#24130=EDGE_CURVE ( 'NONE', #8914, #15622, #18959, .T. ) ;
#24131=CARTESIAN_POINT ( 'NONE',  ( 120.7049497278729575, 40.45429687608393721, -9.295050272127046043 ) ) ;
#24133=CARTESIAN_POINT ( 'NONE',  ( 65.00000000000000000, 38.17226562608394147, -13.14518615778179544 ) ) ;
#24134=CARTESIAN_POINT ( 'NONE',  ( 74.18017581364799184, 50.00000000000000000, -10.00000000000000000 ) ) ;
#24135=CARTESIAN_POINT ( 'NONE',  ( 195.0000000000000000, 33.80664062608393294, 13.14518615778179544 ) ) ;
#24136=ORIENTED_EDGE ( 'NONE', *, *, #15560, .T. ) ;
#24141=ADVANCED_FACE ( 'NONE', ( #4052 ), #1498, .T. ) ;
#24142=CARTESIAN_POINT ( 'NONE',  ( 104.4587341249999639, 79.93750000136559208, -1.442382525525748735E-14 ) ) ;
#24143=CARTESIAN_POINT ( 'NONE',  ( 204.2950502721270425, 37.87460937608393152, -9.295050272127046043 ) ) ;
#24155=CARTESIAN_POINT ( 'NONE',  ( 135.4449143864723055, 36.53515625108393294, -13.14518615778179900 ) ) ;
#24156=CARTESIAN_POINT ( 'NONE',  ( 59.55508561352770158, 33.26093750108393721, -13.14518615778179900 ) ) ;
#24158=CARTESIAN_POINT ( 'NONE',  ( 185.7049497278729575, 37.67617187608393436, 9.295050272127047819 ) ) ;
#24159=ORIENTED_EDGE ( 'NONE', *, *, #19766, .F. ) ;
#24161=CARTESIAN_POINT ( 'NONE',  ( 13.14518615778179900, 32.26875000108393721, -5.444914386472297529 ) ) ;
#24162=CARTESIAN_POINT ( 'NONE',  ( 129.0169348148962172, 49.99999999949010743, -13.54930971656700756 ) ) ;
#24163=PLANE ( 'NONE',  #5779 ) ;
#24164=CARTESIAN_POINT ( 'NONE',  ( 116.4251840539369454, 39.46210937716787726, -5.622872871577873077 ) ) ;
#24166=ADVANCED_FACE ( 'NONE', ( #18942 ), #5848, .T. ) ;
#24170=EDGE_LOOP ( 'NONE', ( #3762, #23936, #5792, #12496, #13807, #5387 ) ) ;
#24176=CARTESIAN_POINT ( 'NONE',  ( 132.5295839951739367, 49.99999999938366813, 13.34625891065843994 ) ) ;
#24178=CARTESIAN_POINT ( 'NONE',  ( 96.84719886470459471, 79.81250000136559208, 3.152801135295355994 ) ) ;
#24179=CARTESIAN_POINT ( 'NONE',  ( 70.44491438647230552, 33.85625000108393579, 13.14518615778179189 ) ) ;
#24181=CARTESIAN_POINT ( 'NONE',  ( 13.14518615778179544, 38.56914062608393579, -1.609821015232357215E-15 ) ) ;
#24183=CARTESIAN_POINT ( 'NONE',  ( 130.0000000000000000, 36.43593749999999432, 13.57481594606304576 ) ) ;
#24185=CARTESIAN_POINT ( 'NONE',  ( 139.5988444088204403, 38.32109374999999574, -9.598844408820458085 ) ) ;
#24188=LINE ( 'NONE', #4667, #9921 ) ;
#24192=CARTESIAN_POINT ( 'NONE',  ( 135.4449143864723055, 36.83281250108392868, 13.14518615778179189 ) ) ;
#24193=CARTESIAN_POINT ( 'NONE',  ( 65.00000000000000000, 34.55078125216787299, -13.57481594606304576 ) ) ;
#24195=CARTESIAN_POINT ( 'NONE',  ( 99.99999999999995737, 83.25000000000000000, 4.999999999999990230 ) ) ;
#24196=CARTESIAN_POINT ( 'NONE',  ( -9.598844408820454532, 33.26093750216787726, 9.598844408820459861 ) ) ;
#24198=CARTESIAN_POINT ( 'NONE',  ( 94.99999999999995737, 84.93750000000001421, -2.071067811865491493 ) ) ;
#24199=CARTESIAN_POINT ( 'NONE',  ( 208.1451861577818079, 35.39414062608393152, -1.609821015232357215E-15 ) ) ;
#24200=DIRECTION ( 'NONE',  ( -0.000000000000000000, 1.000000000000000000, -0.000000000000000000 ) ) ;
#24201=CARTESIAN_POINT ( 'NONE',  ( 124.5550856135277087, 36.43593750108394147, -13.14518615778179722 ) ) ;
#24202=CARTESIAN_POINT ( 'NONE',  ( 204.5988444088204687, 38.91640624999999432, 9.598844408820456309 ) ) ;
#24207=CARTESIAN_POINT ( 'NONE',  ( 139.5988444088204687, 38.12265624999999858, 9.598844408820456309 ) ) ;
#24211=CARTESIAN_POINT ( 'NONE',  ( 185.4011555911795313, 34.55078124999999289, -9.598844408820458085 ) ) ;
#24214=CARTESIAN_POINT ( 'NONE',  ( 78.14518615778179367, 36.93203125108394147, 5.444914386472293977 ) ) ;
#24217=ORIENTED_EDGE ( 'NONE', *, *, #10126, .F. ) ;
#24219=CARTESIAN_POINT ( 'NONE',  ( 9.598844408820459861, 34.94765624999999432, 9.598844408820456309 ) ) ;
#24220=CARTESIAN_POINT ( 'NONE',  ( 116.8548138422182063, 36.83281250108393579, 5.444914386472304635 ) ) ;
#24221=ORIENTED_EDGE ( 'NONE', *, *, #294, .T. ) ;
#24222=CARTESIAN_POINT ( 'NONE',  ( 94.99999999999995737, 83.00000000000000000, -1.387778780781445676E-14 ) ) ;
#24223=CARTESIAN_POINT ( 'NONE',  ( 97.92893218813451028, 82.93750000273119838, -5.000000000000018652 ) ) ;
#24227=CARTESIAN_POINT ( 'NONE',  ( 78.57481594606304043, 39.85898437499999858, -5.622872871577873077 ) ) ;
#24234=CARTESIAN_POINT ( 'NONE',  ( 181.4251840539369596, 35.49335937716787015, -5.622872871577873077 ) ) ;
#24236=CARTESIAN_POINT ( 'NONE',  ( 130.0000000000000000, -7.395377635281828788, -11.57481594606305997 ) ) ;
#24237=CARTESIAN_POINT ( 'NONE',  ( 130.0000000000000000, 36.58476562608393579, -13.14518615778179544 ) ) ;
#24238=CARTESIAN_POINT ( 'NONE',  ( -9.295050272127044266, 34.50117187608393721, 9.295050272127047819 ) ) ;
#24239=EDGE_CURVE ( 'NONE', #19624, #19393, #6254, .T. ) ;
#24240=CARTESIAN_POINT ( 'NONE',  ( 130.0000000000000000, 34.00507812608393721, -13.14518615778179544 ) ) ;
#24241=CARTESIAN_POINT ( 'NONE',  ( 78.57481594606305464, 35.84062499999999574, -1.662435489736055892E-15 ) ) ;
#24244=CARTESIAN_POINT ( 'NONE',  ( 207.3201169669888770, 36.00000000000001421, -5.704949255836485378 ) ) ;
#24247=FACE_OUTER_BOUND ( 'NONE', #20870, .T. ) ;
#24250=CARTESIAN_POINT ( 'NONE',  ( 13.14518615778179544, 36.38632812608393863, -1.609821015232357215E-15 ) ) ;
#24258=CARTESIAN_POINT ( 'NONE',  ( 189.5550856135277229, 35.64218750108392442, -13.14518615778179900 ) ) ;
#24259=VERTEX_POINT ( 'NONE', #14927 ) ;
#24263=ORIENTED_EDGE ( 'NONE', *, *, #16134, .F. ) ;
#24267=CARTESIAN_POINT ( 'NONE',  ( 133.8783854107797424, 31.34156310770110565, -13.57481594606304931 ) ) ;
#24271=CARTESIAN_POINT ( 'NONE',  ( 78.14518615778179367, 38.71796875108393721, 5.444914386472293977 ) ) ;
#24272=EDGE_CURVE ( 'NONE', #13933, #6189, #6479, .T. ) ;
#24273=CARTESIAN_POINT ( 'NONE',  ( 57.91058272766510839, 49.99999999943660356, -11.59823041028830026 ) ) ;
#24274=CARTESIAN_POINT ( 'NONE',  ( 208.5748159460630120, 39.75976562499999289, 5.622872871577869525 ) ) ;
#24276=CARTESIAN_POINT ( 'NONE',  ( 78.39333672780520601, 36.00000000000000000, -2.034633736483404398 ) ) ;
#24277=VERTEX_POINT ( 'NONE', #19782 ) ;
#24280=CARTESIAN_POINT ( 'NONE',  ( 65.00000000000000000, 36.78320312608393294, 13.14518615778179544 ) ) ;
#24282=CARTESIAN_POINT ( 'NONE',  ( 200.4449143864723055, 40.30546875108393579, -13.14518615778179722 ) ) ;
#24285=CARTESIAN_POINT ( 'NONE',  ( 208.1451861577818079, 39.61093750108393863, -5.444914386472297529 ) ) ;
#24287=EDGE_CURVE ( 'NONE', #27029, #18432, #25605, .T. ) ;
#24288=ORIENTED_EDGE ( 'NONE', *, *, #16134, .T. ) ;
#24289=VECTOR ( 'NONE', #692, 1000.000000000000000 ) ;
#24292=VERTEX_POINT ( 'NONE', #6948 ) ;
#24293=CARTESIAN_POINT ( 'NONE',  ( 120.7049497278729575, 33.50898437608393010, -9.295050272127046043 ) ) ;
#24294=CARTESIAN_POINT ( 'NONE',  ( 51.85481384221820633, 33.40976562608393863, 0.000000000000000000 ) ) ;
#24295=CARTESIAN_POINT ( 'NONE',  ( 208.1451861577817795, 38.81718750108393579, -5.444914386472297529 ) ) ;
#24299=LINE ( 'NONE', #22312, #1770 ) ;
#24300=CARTESIAN_POINT ( 'NONE',  ( -8.312177448680279460E-16, 36.03906250000000000, -13.57481594606304576 ) ) ;
#24301=LINE ( 'NONE', #9055, #6707 ) ;
#24304=CARTESIAN_POINT ( 'NONE',  ( 181.8548138422182205, 39.95820312608393010, 0.000000000000000000 ) ) ;
#24309=CARTESIAN_POINT ( 'NONE',  ( 121.7886859848334353, 50.68678854790648103, 15.00000000000135003 ) ) ;
#24313=CARTESIAN_POINT ( 'NONE',  ( 104.4587341249999639, 83.18750000136560629, -1.442382525525748735E-14 ) ) ;
#24314=CARTESIAN_POINT ( 'NONE',  ( 70.44491438647230552, 36.23750000108393721, 13.14518615778179189 ) ) ;
#24316=CARTESIAN_POINT ( 'NONE',  ( -5.444914386472299306, 38.32109375108394289, 13.14518615778179722 ) ) ;
#24318=CARTESIAN_POINT ( 'NONE',  ( 104.9999999999999716, 80.62500000273119838, -1.449011120738813565E-14 ) ) ;
#24321=CARTESIAN_POINT ( 'NONE',  ( 116.4251840539369596, 37.08085937499999574, 5.622872871577880183 ) ) ;
#24323=EDGE_CURVE ( 'NONE', #4141, #26410, #18440, .T. ) ;
#24324=ORIENTED_EDGE ( 'NONE', *, *, #19777, .T. ) ;
#24329=CARTESIAN_POINT ( 'NONE',  ( 120.7049497278729575, 32.51679687608393721, -9.295050272127046043 ) ) ;
#24330=CARTESIAN_POINT ( 'NONE',  ( 78.57481594606305464, 35.14609375216787157, -1.662435489736055892E-15 ) ) ;
#24332=CARTESIAN_POINT ( 'NONE',  ( 195.0000000000000000, 37.62656249999999858, -13.57481594606304576 ) ) ;
#24333=CARTESIAN_POINT ( 'NONE',  ( -13.57481594606304753, 32.31835937716786589, -5.622872871577873077 ) ) ;
#24338=CARTESIAN_POINT ( 'NONE',  ( 185.7049497278729575, 33.31054687608393294, -9.295050272127046043 ) ) ;
#24340=CARTESIAN_POINT ( 'NONE',  ( 193.3974668693900298, 53.60343507248207118, 14.99999999999995026 ) ) ;
#24341=DIRECTION ( 'NONE',  ( -0.000000000000000000, 1.000000000000000000, -0.000000000000000000 ) ) ;
#24343=DIRECTION ( 'NONE',  ( -1.000000000000000000, 0.000000000000000000, 7.228014483236696740E-18 ) ) ;
#24346=CARTESIAN_POINT ( 'NONE',  ( 195.0000000000000000, 34.05468749999999289, 13.57481594606304576 ) ) ;
#24347=EDGE_CURVE ( 'NONE', #27535, #21141, #1656, .T. ) ;
#24350=CARTESIAN_POINT ( 'NONE',  ( 70.44491438647230552, 34.74921875108394431, -13.14518615778179900 ) ) ;
#24355=CARTESIAN_POINT ( 'NONE',  ( 5.622872871577871301, 36.78320312499999289, -13.57481594606304753 ) ) ;
#24356=CARTESIAN_POINT ( 'NONE',  ( 116.8548138422182205, 38.37070312608393152, 0.000000000000000000 ) ) ;
#24357=ORIENTED_EDGE ( 'NONE', *, *, #2356, .F. ) ;
#24358=CARTESIAN_POINT ( 'NONE',  ( 96.46446609406721961, 81.87500000000000000, -3.535533905932755072 ) ) ;
#24359=AXIS2_PLACEMENT_3D ( 'NONE', #16936, #25429, #1715 ) ;
#24361=CARTESIAN_POINT ( 'NONE',  ( 103.5355339059327093, 80.50000000273119838, 3.535533905932726206 ) ) ;
#24365=CARTESIAN_POINT ( 'NONE',  ( 74.29505027212704249, 32.31835937608393294, 9.295050272127046043 ) ) ;
#24372=CARTESIAN_POINT ( 'NONE',  ( 181.4251840539369596, 33.21132812716787441, 5.622872871577880183 ) ) ;
#24376=CARTESIAN_POINT ( 'NONE',  ( 200.6228728715779823, 40.05742187716787583, -13.57481594606294095 ) ) ;
#24377=ORIENTED_EDGE ( 'NONE', *, *, #4744, .T. ) ;
#24378=CARTESIAN_POINT ( 'NONE',  ( 9.295050272127046043, 35.69179687608394147, -9.295050272127046043 ) ) ;
#24380=CARTESIAN_POINT ( 'NONE',  ( 133.7556382656599112, 31.58960998161716560, -13.14518615778179900 ) ) ;
#24381=CARTESIAN_POINT ( 'NONE',  ( 55.40115559117954547, 34.55078124999999289, -9.598844408820458085 ) ) ;
#24382=CYLINDRICAL_SURFACE ( 'NONE', #10472, 13.57481594606304398 ) ;
#24384=CARTESIAN_POINT ( 'NONE',  ( 208.3933367278050923, 36.00000000000000000, -2.034633736484581679 ) ) ;
#24387=DIRECTION ( 'NONE',  ( 0.000000000000000000, -1.000000000000000000, 0.000000000000000000 ) ) ;
#24391=CARTESIAN_POINT ( 'NONE',  ( 5.444914386472297529, 34.94765625108394147, -13.14518615778179900 ) ) ;
#24396=CARTESIAN_POINT ( 'NONE',  ( 99.99999999999995737, 85.00000000000000000, -1.387778780781445676E-14 ) ) ;
#24397=EDGE_CURVE ( 'NONE', #18157, #17002, #19127, .T. ) ;
#24398=CARTESIAN_POINT ( 'NONE',  ( 208.1451861577818079, 34.60039062608392868, -1.609821015232357215E-15 ) ) ;
#24400=CARTESIAN_POINT ( 'NONE',  ( 13.57481594606304931, 39.85898437716787157, 5.622872871577868636 ) ) ;
#24402=ORIENTED_EDGE ( 'NONE', *, *, #26943, .F. ) ;
#24407=CARTESIAN_POINT ( 'NONE',  ( 120.4011555911795455, 31.47500000216787441, -9.598844408820458085 ) ) ;
#24410=CARTESIAN_POINT ( 'NONE',  ( 74.29505027212704249, 38.66835937608393436, 9.295050272127046043 ) ) ;
#24411=CARTESIAN_POINT ( 'NONE',  ( 56.79855381236158252, 50.69246985422713436, -14.99999999999860201 ) ) ;
#24413=CARTESIAN_POINT ( 'NONE',  ( 195.0000000000000000, 40.00781250000000000, -13.57481594606304576 ) ) ;
#24415=( BOUNDED_CURVE ( )  B_SPLINE_CURVE ( 2, ( #3648, #1379, #22897, #5651, #12168, #16608, #25580, #1793, #14456 ),
 .UNSPECIFIED., .F., .F. ) 
 B_SPLINE_CURVE_WITH_KNOTS ( ( 3, 2, 2, 2, 3 ),
 ( 0.3500000000000003109, 0.3750000000000003331, 0.4000000000000003553, 0.4250000000000003775, 0.4500000000000003997 ),
 .UNSPECIFIED. ) 
 CURVE ( )  GEOMETRIC_REPRESENTATION_ITEM ( )  RATIONAL_B_SPLINE_CURVE ( ( 0.9999999999999990008, 0.9238795325112877377, 1.000000000000000000, 0.9238795325112867385, 1.000000000000000000, 0.9238795325112867385, 1.000000000000000000, 0.9238795325112855172, 1.000000000000001110 ) ) 
 REPRESENTATION_ITEM ( '' )  );
#24419=CARTESIAN_POINT ( 'NONE',  ( 55.70494972787295751, 38.27148437608393294, 9.295050272127047819 ) ) ;
#24420=CARTESIAN_POINT ( 'NONE',  ( 65.00000000000000000, 36.13828125216787157, -13.57481594606304576 ) ) ;
#24422=ORIENTED_EDGE ( 'NONE', *, *, #6530, .F. ) ;
#24426=CARTESIAN_POINT ( 'NONE',  ( 185.7049497278729575, 37.47773437608393010, -9.295050272127046043 ) ) ;
#24433=EDGE_LOOP ( 'NONE', ( #1704, #6756, #4664, #2624 ) ) ;
#24434=CARTESIAN_POINT ( 'NONE',  ( 116.8548138422182063, 31.97109375108393436, -5.444914386472297529 ) ) ;
#24436=CARTESIAN_POINT ( 'NONE',  ( 204.2950502721270425, 34.89804687608393863, -9.295050272127046043 ) ) ;
#24439=CARTESIAN_POINT ( 'NONE',  ( 9.295050272127046043, 33.11210937608393579, -9.295050272127046043 ) ) ;
#24442=DIRECTION ( 'NONE',  ( -0.000000000000000000, -1.000000000000000000, -0.000000000000000000 ) ) ;
#24443=DIRECTION ( 'NONE',  ( -0.000000000000000000, 1.000000000000000000, -0.000000000000000000 ) ) ;
#24446=CARTESIAN_POINT ( 'NONE',  ( 71.08594421599755719, 54.65299103241510181, 14.99999999999997868 ) ) ;
#24448=SURFACE_SIDE_STYLE ('',( #5216 ) ) ;
#24453=CARTESIAN_POINT ( 'NONE',  ( 195.0000000000000000, 38.42031249999999432, -13.57481594606304576 ) ) ;
#24457=CARTESIAN_POINT ( 'NONE',  ( 74.59884440882045453, 37.62656250216787157, -9.598844408820458085 ) ) ;
#24458=ADVANCED_FACE ( 'NONE', ( #553 ), #15782, .F. ) ;
#24459=CARTESIAN_POINT ( 'NONE',  ( 185.4011555911795313, 37.72578124999999005, -9.598844408820458085 ) ) ;
#24460=CARTESIAN_POINT ( 'NONE',  ( -5.444914386472297529, 38.02343750108394005, -13.14518615778179722 ) ) ;
#24461=VECTOR ( 'NONE', #10613, 1000.000000000000000 ) ;
#24464=CARTESIAN_POINT ( 'NONE',  ( -6.117759945536496602, 54.65941425414899868, 14.99999999999999822 ) ) ;
#24466=CARTESIAN_POINT ( 'NONE',  ( 139.5988444088204687, 37.32890624999999574, 9.598844408820456309 ) ) ;
#24467=ORIENTED_EDGE ( 'NONE', *, *, #7379, .T. ) ;
#24473=CARTESIAN_POINT ( 'NONE',  ( 135.4449143864723055, 32.07031250108393294, 13.14518615778179189 ) ) ;
#24474=EDGE_CURVE ( 'NONE', #15169, #3638, #24487, .T. ) ;
#24475=CARTESIAN_POINT ( 'NONE',  ( 51.42518405393695957, 35.49335937716787015, -5.622872871577873077 ) ) ;
#24476=EDGE_CURVE ( 'NONE', #19007, #8752, #25054, .T. ) ;
#24477=DIRECTION ( 'NONE',  ( 0.000000000000000000, -1.000000000000000000, -0.000000000000000000 ) ) ;
#24478=CARTESIAN_POINT ( 'NONE',  ( 5.622872871577871301, 33.70742187716787441, -13.57481594606304753 ) ) ;
#24479=FACE_OUTER_BOUND ( 'NONE', #14641, .T. ) ;
#24481=CARTESIAN_POINT ( 'NONE',  ( 189.5550856135277229, 32.76484375108393010, 13.14518615778179722 ) ) ;
#24487=LINE ( 'NONE', #16210, #10113 ) ;
#24492=CARTESIAN_POINT ( 'NONE',  ( 195.0000000000000000, 32.86406249999999574, -13.57481594606304576 ) ) ;
#24494=CARTESIAN_POINT ( 'NONE',  ( 65.00000000000000000, 50.00000000000000000, -7.517135062566165128E-15 ) ) ;
#24496=CARTESIAN_POINT ( 'NONE',  ( 78.14518615778179367, 34.55078125108393294, 5.444914386472293977 ) ) ;
#24499=CARTESIAN_POINT ( 'NONE',  ( 124.3771271284221598, 38.07304687716787583, 13.57481594606308128 ) ) ;
#24500=CARTESIAN_POINT ( 'NONE',  ( 9.598844408820456309, 32.76484374999999716, -9.598844408820458085 ) ) ;
#24501=CARTESIAN_POINT ( 'NONE',  ( 135.4449143864723055, 38.12265625108393152, -13.14518615778179900 ) ) ;
#24503=ORIENTED_EDGE ( 'NONE', *, *, #8798, .T. ) ;
#24504=CARTESIAN_POINT ( 'NONE',  ( 97.92893218813451028, 81.18750000000001421, 4.999999999999989342 ) ) ;
#24506=CARTESIAN_POINT ( 'NONE',  ( 97.92893218813451028, 81.31250000273121259, 4.999999999999989342 ) ) ;
#24511=CARTESIAN_POINT ( 'NONE',  ( 51.85481384221820633, 32.81445312608393294, 0.000000000000000000 ) ) ;
#24514=CARTESIAN_POINT ( 'NONE',  ( 130.0000000000000000, 39.31328125216787583, -13.57481594606304576 ) ) ;
#24519=CARTESIAN_POINT ( 'NONE',  ( 204.5988444088204687, 35.04687500216787299, 9.598844408820456309 ) ) ;
#24524=CARTESIAN_POINT ( 'NONE',  ( -5.444914386472299306, 36.13828125108393863, 13.14518615778179722 ) ) ;
#24528=CARTESIAN_POINT ( 'NONE',  ( 120.8843427382055893, 35.99999999999998579, 9.510219181138795719 ) ) ;
#24532=VECTOR ( 'NONE', #15063, 1000.000000000000000 ) ;
#24536=CARTESIAN_POINT ( 'NONE',  ( -5.444914386472299306, 35.34453125108393579, 13.14518615778179722 ) ) ;
#24541=CARTESIAN_POINT ( 'NONE',  ( 2.493653234604083739E-15, 36.43593749999999432, 13.57481594606304576 ) ) ;
#24543=CARTESIAN_POINT ( 'NONE',  ( 181.8548138422181921, 34.25312500108393010, 5.444914386472304635 ) ) ;
#24546=CARTESIAN_POINT ( 'NONE',  ( 204.1801758136480203, 50.00000000000000000, -14.99999999999999822 ) ) ;
#24551=( GEOMETRIC_REPRESENTATION_CONTEXT ( 3 ) GLOBAL_UNCERTAINTY_ASSIGNED_CONTEXT ( ( #12945 ) ) GLOBAL_UNIT_ASSIGNED_CONTEXT ( ( #13881, #19743, #4648 ) ) REPRESENTATION_CONTEXT ( 'NONE', 'WORKASPACE' ) );
#24552=CARTESIAN_POINT ( 'NONE',  ( 94.99999999999995737, 79.18750000273121259, 2.071067811865466624 ) ) ;
#24553=MECHANICAL_DESIGN_GEOMETRIC_PRESENTATION_REPRESENTATION('',(#26847),#20917);
#24554=CARTESIAN_POINT ( 'NONE',  ( 143.1451861577818079, 37.77539062608393294, -1.609821015232357215E-15 ) ) ;
#24555=CARTESIAN_POINT ( 'NONE',  ( 13.14518615778179544, 40.35507812608393863, -1.609821015232357215E-15 ) ) ;
#24556=CARTESIAN_POINT ( 'NONE',  ( -13.14518615778179900, 34.94765625108392726, -5.444914386472297529 ) ) ;
#24558=CARTESIAN_POINT ( 'NONE',  ( 70.44491438647230552, 37.82500000108392868, 13.14518615778179189 ) ) ;
#24559=CARTESIAN_POINT ( 'NONE',  ( 72.63624106799308322, 54.91786508990981730, -15.00000000000000000 ) ) ;
#24561=CARTESIAN_POINT ( 'NONE',  ( 200.4449143864723055, 32.56640625108394005, -13.14518615778179900 ) ) ;
#24562=DIRECTION ( 'NONE',  ( 0.000000000000000000, 0.000000000000000000, -1.000000000000000000 ) ) ;
#24566=CARTESIAN_POINT ( 'NONE',  ( 78.14518615778179367, 37.77539062608393294, -1.609821015232357215E-15 ) ) ;
#24570=ORIENTED_EDGE ( 'NONE', *, *, #23409, .F. ) ;
#24571=CARTESIAN_POINT ( 'NONE',  ( 130.0000000000000000, 39.21406249999999716, -13.57481594606304576 ) ) ;
#24573=CARTESIAN_POINT ( 'NONE',  ( 195.0000000000000000, 38.56914062608393579, 13.14518615778179544 ) ) ;
#24579=CARTESIAN_POINT ( 'NONE',  ( 143.1451861577818079, 34.00507812608393721, -1.609821015232357215E-15 ) ) ;
#24580=AXIS2_PLACEMENT_3D ( 'NONE', #25446, #5927, #23313 ) ;
#24581=CARTESIAN_POINT ( 'NONE',  ( 185.7049497278729575, 32.71523437608393436, -9.295050272127046043 ) ) ;
#24582=VERTEX_POINT ( 'NONE', #20644 ) ;
#24585=CARTESIAN_POINT ( 'NONE',  ( 120.8198241863519655, 55.00000000000000000, -15.00000000000000000 ) ) ;
#24586=CARTESIAN_POINT ( 'NONE',  ( 124.3771271284221314, 38.56914062716788294, -13.57481594606304753 ) ) ;
#24591=B_SPLINE_CURVE_WITH_KNOTS ( 'NONE', 3,
 ( #24025, #3945, #4503, #27748, #8346, #13160, #21471, #21899, #8208, #12604, #10616, #25595, #14745, #12878, #21328, #10474, #19182, #1947 ),
 .UNSPECIFIED., .F., .F.,
 ( 4, 2, 2, 2, 2, 2, 2, 2, 4 ),
 ( 0.000000000000000000, 0.004618502246277159280, 0.006927753369415741089, 0.009237004492554322030, 0.01039163005412361424, 0.01154625561569290644, 0.01385550673883148391, 0.01616475786197006312, 0.01847400898510863712 ),
 .UNSPECIFIED. ) ;
#24592=CARTESIAN_POINT ( 'NONE',  ( 66.81435535458352604, 51.46618445021699273, 14.99999999999929834 ) ) ;
#24593=PRODUCT_DEFINITION ( 'UNKNOWN', '', #26804, #14597 ) ;
#24594=VECTOR ( 'NONE', #9666, 1000.000000000000000 ) ;
#24596=VERTEX_POINT ( 'NONE', #987 ) ;
#24597=SURFACE_STYLE_USAGE ( .BOTH. , #24448 ) ;
#24599=VERTEX_POINT ( 'NONE', #9796 ) ;
#24602=CARTESIAN_POINT ( 'NONE',  ( 130.0000000000000000, 38.12265625216787157, 13.57481594606304576 ) ) ;
#24604=CARTESIAN_POINT ( 'NONE',  ( 195.0000000000000000, 40.10703125216787157, -13.57481594606304576 ) ) ;
#24608=CARTESIAN_POINT ( 'NONE',  ( -13.14518615778179722, 38.12265625108393863, -5.444914386472297529 ) ) ;
#24610=CARTESIAN_POINT ( 'NONE',  ( 1.814355354584273661, 51.46618445021836408, 15.00000000000034106 ) ) ;
#24612=CARTESIAN_POINT ( 'NONE',  ( 139.5988444088204687, 34.15390624999999858, 9.598844408820456309 ) ) ;
#24613=ORIENTED_EDGE ( 'NONE', *, *, #2854, .T. ) ;
#24618=CARTESIAN_POINT ( 'NONE',  ( 139.2950502721270425, 33.11210937608393579, -9.295050272127046043 ) ) ;
#24619=CARTESIAN_POINT ( 'NONE',  ( 51.42518405393695957, 31.52460937716787370, -5.622872871577873077 ) ) ;
#24621=CARTESIAN_POINT ( 'NONE',  ( 2.493653234604083739E-15, 38.12265625216787157, 13.57481594606304576 ) ) ;
#24622=CARTESIAN_POINT ( 'NONE',  ( 13.14518615778179544, 37.77539062608393294, -1.609821015232357215E-15 ) ) ;
#24627=CARTESIAN_POINT ( 'NONE',  ( -9.295050272127046043, 40.45429687608393721, -9.295050272127046043 ) ) ;
#24628=FACE_OUTER_BOUND ( 'NONE', #8214, .T. ) ;
#24629=DIRECTION ( 'NONE',  ( 0.000000000000000000, 1.000000000000000000, -0.000000000000000000 ) ) ;
#24631=CARTESIAN_POINT ( 'NONE',  ( 181.4251840539369596, 40.25585937499999289, 5.622872871577880183 ) ) ;
#24635=CARTESIAN_POINT ( 'NONE',  ( 130.0000000000000000, -7.395377635281828788, -1.503427012513233026E-14 ) ) ;
#24638=EDGE_CURVE ( 'NONE', #2105, #17002, #15917, .T. ) ;
#24640=CIRCLE ( 'NONE', #25988, 5.000000000000004441 ) ;
#24644=CARTESIAN_POINT ( 'NONE',  ( 78.14518615778179367, 40.40468750108393436, -5.444914386472297529 ) ) ;
#24649=CARTESIAN_POINT ( 'NONE',  ( 9.598844408820459861, 34.15390624999999858, 9.598844408820456309 ) ) ;
#24650=CARTESIAN_POINT ( 'NONE',  ( 143.1451861577818079, 38.02343750108395426, -5.444914386472297529 ) ) ;
#24652=CARTESIAN_POINT ( 'NONE',  ( 94.99999999999995737, 81.93750000000001421, -2.071067811865491048 ) ) ;
#24654=CARTESIAN_POINT ( 'NONE',  ( 99.99999999999995737, 84.18750000136560629, -4.458734125000016313 ) ) ;
#24656=CARTESIAN_POINT ( 'NONE',  ( 59.37712712842213136, 39.36289062716787157, -13.57481594606304753 ) ) ;
#24659=CARTESIAN_POINT ( 'NONE',  ( 74.29505027212704249, 33.11210937608393579, 9.295050272127046043 ) ) ;
#24661=ORIENTED_EDGE ( 'NONE', *, *, #15225, .T. ) ;
#24665=CARTESIAN_POINT ( 'NONE',  ( 200.6228728715778686, 33.40976562716787157, 13.57481594606304576 ) ) ;
#24670=CARTESIAN_POINT ( 'NONE',  ( -13.14518615778179544, 34.40195312608393152, 0.000000000000000000 ) ) ;
#24671=CARTESIAN_POINT ( 'NONE',  ( 130.0000000000000000, 33.21132812608393436, -13.14518615778179544 ) ) ;
#24677=CARTESIAN_POINT ( 'NONE',  ( 189.3771271284222735, 36.88242187499999858, -13.57481594606318254 ) ) ;
#24682=CARTESIAN_POINT ( 'NONE',  ( 9.180175813647995398, 55.00000000000000000, 14.99999999999999467 ) ) ;
#24683=CARTESIAN_POINT ( 'NONE',  ( 5.444914386472302859, 32.26875000108393721, 13.14518615778179189 ) ) ;
#24686=CARTESIAN_POINT ( 'NONE',  ( 116.4251840539369596, 36.98164062499999005, -5.622872871577872189 ) ) ;
#24688=DIRECTION ( 'NONE',  ( 3.469446951953613696E-16, 0.000000000000000000, 1.000000000000000000 ) ) ;
#24689=CARTESIAN_POINT ( 'NONE',  ( 185.7049497278729575, 36.48554687608393721, -9.295050272127046043 ) ) ;
#24691=CARTESIAN_POINT ( 'NONE',  ( 186.6077847083615495, 54.99999999999997868, -14.99999999999999645 ) ) ;
#24693=ORIENTED_EDGE ( 'NONE', *, *, #15166, .F. ) ;
#24696=CARTESIAN_POINT ( 'NONE',  ( 217.9999999999999716, 52.00000000000000711, -13.00000000000000000 ) ) ;
#24698=CARTESIAN_POINT ( 'NONE',  ( 120.7049497278729575, 36.48554687608393721, -9.295050272127046043 ) ) ;
#24699=CARTESIAN_POINT ( 'NONE',  ( 2.414731522848535132E-15, 37.77539062608393294, 13.14518615778179544 ) ) ;
#24700=CARTESIAN_POINT ( 'NONE',  ( -5.444914386472297529, 34.05468750108393294, -13.14518615778179900 ) ) ;
#24702=CARTESIAN_POINT ( 'NONE',  ( -13.57481594606304398, 36.38632812716788578, 5.622872871577880183 ) ) ;
#24705=CARTESIAN_POINT ( 'NONE',  ( 68.30411859782175554, 35.99999999999998579, 12.77244747738262731 ) ) ;
#24709=CARTESIAN_POINT ( 'NONE',  ( 59.55508561352770158, 37.22968750108394431, -13.14518615778179722 ) ) ;
#24710=PRODUCT_DEFINITION_SHAPE ( 'NONE', 'NONE',  #24593 ) ;
#24711=EDGE_CURVE ( 'NONE', #12289, #4613, #4546, .T. ) ;
#24713=CARTESIAN_POINT ( 'NONE',  ( 185.7049497278729575, 36.48554687608393721, -9.295050272127046043 ) ) ;
#24717=CARTESIAN_POINT ( 'NONE',  ( 189.5550856135277229, 39.31328125108392868, 13.14518615778179722 ) ) ;
#24719=ORIENTED_EDGE ( 'NONE', *, *, #13648, .F. ) ;
#24723=CARTESIAN_POINT ( 'NONE',  ( 135.4449143864723055, 33.36015625108393579, -13.14518615778179900 ) ) ;
#24724=CARTESIAN_POINT ( 'NONE',  ( 195.0000000000000000, 36.93203125216787441, -13.57481594606304576 ) ) ;
#24725=CARTESIAN_POINT ( 'NONE',  ( 195.0000000000000000, 34.99726562608393721, -13.14518615778179544 ) ) ;
#24726=ORIENTED_EDGE ( 'NONE', *, *, #22826, .T. ) ;
#24730=CARTESIAN_POINT ( 'NONE',  ( 116.4251840539369596, 36.33671875216787583, 0.000000000000000000 ) ) ;
#24732=DIRECTION ( 'NONE',  ( 0.000000000000000000, -1.000000000000000000, 0.000000000000000000 ) ) ;
#24734=CARTESIAN_POINT ( 'NONE',  ( 195.0000000000000000, 40.15664062608393436, 13.14518615778179544 ) ) ;
#24735=FILL_AREA_STYLE_COLOUR ( '', #10413 ) ;
#24738=CARTESIAN_POINT ( 'NONE',  ( 3.089260913797906571, 36.00000000000000000, -13.21136010216355672 ) ) ;
#24740=CARTESIAN_POINT ( 'NONE',  ( 133.0446094569239506, 53.89089363584123760, 14.99999999999996447 ) ) ;
#24741=CARTESIAN_POINT ( 'NONE',  ( -9.115657261794684274, 36.00000000000000000, 9.510219181138523936 ) ) ;
#24742=CARTESIAN_POINT ( 'NONE',  ( 65.00000000000000000, 33.40976562608393863, -13.14518615778179544 ) ) ;
#24746=CARTESIAN_POINT ( 'NONE',  ( -13.57481594606304753, 38.56914062499999574, -5.622872871577872189 ) ) ;
#24748=CARTESIAN_POINT ( 'NONE',  ( 0.3286002765677282222, 53.49358765998907472, 14.99999999999999645 ) ) ;
#24749=CARTESIAN_POINT ( 'NONE',  ( 130.0000000000000000, 35.24531249999999716, -13.57481594606304576 ) ) ;
#24750=ORIENTED_EDGE ( 'NONE', *, *, #22413, .F. ) ;
#24751=DIRECTION ( 'NONE',  ( -0.000000000000000000, 1.000000000000000000, -0.000000000000000000 ) ) ;
#24755=CARTESIAN_POINT ( 'NONE',  ( 116.8548138422182063, 32.66562500108393863, 5.444914386472304635 ) ) ;
#24756=CARTESIAN_POINT ( 'NONE',  ( 65.00000000000000000, 40.35507812608393152, -13.14518615778179544 ) ) ;
#24759=CARTESIAN_POINT ( 'NONE',  ( 130.0000000000000000, -7.395377635281828788, -1.503427012513233026E-14 ) ) ;
#24760=CARTESIAN_POINT ( 'NONE',  ( -5.444914386472297529, 38.81718750108393579, -13.14518615778179900 ) ) ;
#24762=CARTESIAN_POINT ( 'NONE',  ( -15.00000000000000000, 55.00000000000000000, 10.00000000000000000 ) ) ;
#24765=CARTESIAN_POINT ( 'NONE',  ( 189.5550856135277229, 32.46718750108393436, -13.14518615778179900 ) ) ;
#24769=CARTESIAN_POINT ( 'NONE',  ( 195.0000000000000000, 39.61093749999999147, 13.57481594606304576 ) ) ;
#24779=CARTESIAN_POINT ( 'NONE',  ( 104.4587341249999781, 83.00000000136559208, -1.846868145590750299 ) ) ;
#24780=CARTESIAN_POINT ( 'NONE',  ( 65.00000000000000000, 33.21132812608393436, -13.14518615778179544 ) ) ;
#24781=DIRECTION ( 'NONE',  ( 0.000000000000000000, 0.000000000000000000, -1.000000000000000000 ) ) ;
#24782=DIRECTION ( 'NONE',  ( 0.000000000000000000, 0.000000000000000000, 1.000000000000000000 ) ) ;
#24783=CARTESIAN_POINT ( 'NONE',  ( 116.4251840539369596, 37.87460937716787868, -5.622872871577872189 ) ) ;
#24784=CARTESIAN_POINT ( 'NONE',  ( -8.312177448680279460E-16, 34.45156249999999432, -13.57481594606304576 ) ) ;
#24785=CARTESIAN_POINT ( 'NONE',  ( 143.1451861577818079, 34.74921875108395142, 5.444914386472293977 ) ) ;
#24789=CARTESIAN_POINT ( 'NONE',  ( 99.99999999999995737, 79.87500000273119838, -5.000000000000018652 ) ) ;
#24791=CARTESIAN_POINT ( 'NONE',  ( 70.62287287157786864, 40.05742187716786873, -13.57481594606304753 ) ) ;
#24793=CARTESIAN_POINT ( 'NONE',  ( 65.00000000000000000, 40.80156249999999574, -13.57481594606304576 ) ) ;
#24794=CARTESIAN_POINT ( 'NONE',  ( -5.622872871577873077, 38.56914062716788294, -13.57481594606304753 ) ) ;
#24797=CARTESIAN_POINT ( 'NONE',  ( 65.00000000000000000, 36.43593749999999432, 13.57481594606304576 ) ) ;
#24802=CARTESIAN_POINT ( 'NONE',  ( 185.7049497278729575, 39.66054687608393436, -9.295050272127046043 ) ) ;
#24806=CARTESIAN_POINT ( 'NONE',  ( -5.444914386472297529, 32.66562500108393863, -13.14518615778179900 ) ) ;
#24807=CARTESIAN_POINT ( 'NONE',  ( 143.1451861577818079, 32.26875000108393721, -5.444914386472297529 ) ) ;
#24819=CARTESIAN_POINT ( 'NONE',  ( 3.755638155860017591, 31.78804748261757140, -13.14518615778179367 ) ) ;
#24825=CARTESIAN_POINT ( 'NONE',  ( 195.0000000000000000, 35.59257812608393579, -13.14518615778179544 ) ) ;
#24828=CARTESIAN_POINT ( 'NONE',  ( 193.1856446454109459, 51.46618445022109256, -15.00000000000000000 ) ) ;
#24830=EDGE_CURVE ( 'NONE', #10007, #24596, #7468, .T. ) ;
#24833=CIRCLE ( 'NONE', #28005, 4.999999999999997335 ) ;
#24836=CARTESIAN_POINT ( 'NONE',  ( 9.180175813647991845, 50.00000000000000000, -9.999999999999998224 ) ) ;
#24838=CARTESIAN_POINT ( 'NONE',  ( 143.1451861577818079, 38.61875000108393152, -5.444914386472297529 ) ) ;
#24839=CARTESIAN_POINT ( 'NONE',  ( -13.14518615778179544, 36.78320312608393294, 0.000000000000000000 ) ) ;
#24840=CARTESIAN_POINT ( 'NONE',  ( -9.295050272127046043, 34.89804687608393152, -9.295050272127046043 ) ) ;
#24844=CARTESIAN_POINT ( 'NONE',  ( 71.11775994554184877, 54.65941425414899157, -15.00000000000000000 ) ) ;
#24851=CARTESIAN_POINT ( 'NONE',  ( 74.29505027212704249, 38.66835937608393436, -9.295050272127046043 ) ) ;
#24857=CARTESIAN_POINT ( 'NONE',  ( 181.8548138422182205, 39.11484375108393863, -5.444914386472297529 ) ) ;
#24863=CARTESIAN_POINT ( 'NONE',  ( 135.4449143864723055, 33.85625000108393579, 13.14518615778179189 ) ) ;
#24864=CARTESIAN_POINT ( 'NONE',  ( 51.85481384221821344, 40.00781250108393294, 5.444914386472304635 ) ) ;
#24866=CARTESIAN_POINT ( 'NONE',  ( 208.1451861577817795, 33.95546875108393436, 5.444914386472293977 ) ) ;
#24869=DIRECTION ( 'NONE',  ( -0.000000000000000000, 1.000000000000000000, -0.000000000000000000 ) ) ;
#24870=EDGE_CURVE ( 'NONE', #25247, #11161, #21656, .T. ) ;
#24871=CARTESIAN_POINT ( 'NONE',  ( 124.3771271284221314, 37.77539062716788010, -13.57481594606304753 ) ) ;
#24874=AXIS2_PLACEMENT_3D ( 'NONE', #16423, #9729, #11854 ) ;
#24877=CARTESIAN_POINT ( 'NONE',  ( 74.18017581364802027, 49.99999999999999289, 14.99999999999997513 ) ) ;
#24884=CARTESIAN_POINT ( 'NONE',  ( 136.1198436276953032, 51.28708186915216771, 14.99999999999926992 ) ) ;
#24885=CARTESIAN_POINT ( 'NONE',  ( -13.09590655363597733, 36.00000000000000000, 1.137167824541468031 ) ) ;
#24886=CARTESIAN_POINT ( 'NONE',  ( 65.00000000000000000, 37.72578125216787726, -13.57481594606304576 ) ) ;
#24889=CARTESIAN_POINT ( 'NONE',  ( 96.46446609406721961, 81.12500000000000000, 3.535533905932727539 ) ) ;
#24891=CARTESIAN_POINT ( 'NONE',  ( 3.803054373245578823, 54.09082899096177499, 14.99999999999999645 ) ) ;
#24893=CARTESIAN_POINT ( 'NONE',  ( 135.6228728715778686, 34.40195312499999858, -13.57481594606304753 ) ) ;
#24895=DIRECTION ( 'NONE',  ( 1.156482317317871478E-16, 0.000000000000000000, 1.000000000000000000 ) ) ;
#24900=CARTESIAN_POINT ( 'NONE',  ( 139.2950502721270425, 32.11992187608393579, 9.295050272127046043 ) ) ;
#24901=CARTESIAN_POINT ( 'NONE',  ( 65.00000000000000000, 39.16445312608392726, 13.14518615778179544 ) ) ;
#24903=CARTESIAN_POINT ( 'NONE',  ( 5.444914386472302859, 40.00781250108393294, 13.14518615778179189 ) ) ;
#24906=DIRECTION ( 'NONE',  ( 0.000000000000000000, 0.000000000000000000, -1.000000000000000000 ) ) ;
#24908=DIRECTION ( 'NONE',  ( 0.000000000000000000, 0.000000000000000000, 1.000000000000000000 ) ) ;
#24911=CARTESIAN_POINT ( 'NONE',  ( 123.5294363033336822, 36.00000000000001421, -11.78199955157030487 ) ) ;
#24917=CARTESIAN_POINT ( 'NONE',  ( 195.0000000000000000, 32.46718749999999432, 13.57481594606304576 ) ) ;
#24921=CARTESIAN_POINT ( 'NONE',  ( 78.14518615778179367, 33.06250000108393294, -5.444914386472297529 ) ) ;
#24925=FACE_OUTER_BOUND ( 'NONE', #533, .T. ) ;
#24927=CARTESIAN_POINT ( 'NONE',  ( 143.1451861577818079, 34.84843750108393579, -5.444914386472297529 ) ) ;
#24929=CARTESIAN_POINT ( 'NONE',  ( 102.0710678118654329, 80.31250000000000000, 4.999999999999989342 ) ) ;
#24931=CARTESIAN_POINT ( 'NONE',  ( 99.99999999999995737, 82.18750000136559208, -4.458734125000016313 ) ) ;
#24933=CARTESIAN_POINT ( 'NONE',  ( 65.00000000000000000, 36.00000000000000000, 11.57481594606303688 ) ) ;
#24935=CARTESIAN_POINT ( 'NONE',  ( 181.8548138422182205, 40.75195312608393294, 0.000000000000000000 ) ) ;
#24936=CARTESIAN_POINT ( 'NONE',  ( -9.598844408820458085, 38.61875000216787157, -9.598844408820458085 ) ) ;
#24937=EDGE_LOOP ( 'NONE', ( #24217, #9029, #6136, #11695 ) ) ;
#24940=ORIENTED_EDGE ( 'NONE', *, *, #6691, .T. ) ;
#24942=CARTESIAN_POINT ( 'NONE',  ( 181.8548138422181921, 39.71015625108393010, -5.444914386472297529 ) ) ;
#24945=CARTESIAN_POINT ( 'NONE',  ( 130.0000000000000000, 39.95820312608393010, 13.14518615778179544 ) ) ;
#24946=CARTESIAN_POINT ( 'NONE',  ( -9.295050272127044266, 32.91367187608393152, 9.295050272127047819 ) ) ;
#24951=CARTESIAN_POINT ( 'NONE',  ( 195.0000000000000000, 50.00000000000000000, 13.57481594606302266 ) ) ;
#24959=LINE ( 'NONE', #5445, #14800 ) ;
#24960=CARTESIAN_POINT ( 'NONE',  ( -13.14518615778179544, 32.81445312608393294, 0.000000000000000000 ) ) ;
#24961=CIRCLE ( 'NONE', #11749, 13.57481594606304398 ) ;
#24963=DIRECTION ( 'NONE',  ( 0.000000000000000000, 0.000000000000000000, 1.000000000000000000 ) ) ;
#24964=( BOUNDED_CURVE ( )  B_SPLINE_CURVE ( 2, ( #2781, #7613, #791, #935, #15731, #5202, #4922, #13867, #13585, #27015, #22306, #22593, #27161, #7462, #16157, #24864, #22734, #3200, #11871, #1076, #12424, #1490, #3480, #23289, #25559, #1629, #20869, #18996, #1353, #5627, #3625, #21430, #6039, #27567, #25275, #12705, #14433, #23149, #5764, #1767, #16991, #25690, #12286, #21142, #19141, #8302, #7888, #21010, #23009, #10433, #10018, #21285, #16725, #5906, #3897, #10289, #27846, #27296, #18591, #6174, #14841, #27705, #12559, #18857, #8169, #23423, #3763, #8027, #23563, #14705, #10145, #4041, #14572, #9883, #16860, #18727, #25422, #7753, #12145, #16440, #25137, #14293, #27425, #16583, #15262, #17416, #2328, #23981, #8724, #17557, #5133, #8865, #28119, #13799, #21852, #1910, #6721 ),
 .UNSPECIFIED., .F., .F. ) 
 B_SPLINE_CURVE_WITH_KNOTS ( ( 3, 2, 2, 2, 2, 2, 2, 2, 2, 2, 2, 2, 2, 2, 2, 2, 2, 2, 2, 2, 2, 2, 2, 2, 2, 2, 2, 2, 2, 2, 2, 2, 2, 2, 2, 2, 2, 2, 2, 2, 2, 2, 2, 2, 2, 2, 2, 2, 3 ),
 ( 0.000000000000000000, 0.01041666666666666609, 0.02083333333333333218, 0.03125000000000000000, 0.04166666666666666435, 0.05208333333333333565, 0.06250000000000000000, 0.07291666666666667129, 0.08333333333333332871, 0.09374999999999998612, 0.1041666666666666713, 0.1145833333333333287, 0.1250000000000000000, 0.1354166666666666574, 0.1458333333333333426, 0.1562500000000000000, 0.1666666666666666574, 0.1770833333333333426, 0.1874999999999999722, 0.1979166666666666574, 0.2083333333333333426, 0.2187500000000000000, 0.2291666666666666574, 0.2395833333333333426, 0.2500000000000000000, 0.2604166666666666852, 0.2708333333333333148, 0.2812500000000000000, 0.2916666666666666852, 0.3020833333333333148, 0.3125000000000000000, 0.3229166666666666852, 0.3333333333333333148, 0.3437500000000000000, 0.3541666666666666852, 0.3645833333333333148, 0.3749999999999999445, 0.3854166666666666852, 0.3958333333333333148, 0.4062500000000000000, 0.4166666666666666852, 0.4270833333333333148, 0.4375000000000000000, 0.4479166666666666852, 0.4583333333333333148, 0.4687500000000000000, 0.4791666666666666852, 0.4895833333333333148, 0.4988304892921909817 ),
 .UNSPECIFIED. ) 
 CURVE ( )  GEOMETRIC_REPRESENTATION_ITEM ( )  RATIONAL_B_SPLINE_CURVE ( ( 1.000000000000000000, 0.9238795325112867385, 1.000000000000000000, 0.9238795325112867385, 1.000000000000000000, 0.9238795325112867385, 1.000000000000000000, 0.9238795325112867385, 1.000000000000000000, 0.9238795325112867385, 1.000000000000000000, 0.9238795325112867385, 1.000000000000000000, 0.9238795325112867385, 1.000000000000000000, 0.9238795325112867385, 1.000000000000000000, 0.9238795325112867385, 1.000000000000000000, 0.9238795325112867385, 1.000000000000000000, 0.9238795325112867385, 1.000000000000000000, 0.9238795325112867385, 1.000000000000000000, 0.9238795325112867385, 1.000000000000000000, 0.9238795325112867385, 1.000000000000000000, 0.9238795325112867385, 1.000000000000000000, 0.9238795325112867385, 1.000000000000000000, 0.9238795325112867385, 1.000000000000000000, 0.9238795325112867385, 1.000000000000000000, 0.9238795325112867385, 1.000000000000000000, 0.9238795325112867385, 1.000000000000000000, 0.9238795325112867385, 1.000000000000000000, 0.9238795325112867385, 1.000000000000000000, 0.9238795325112867385, 1.000000000000000000, 0.9238795325112867385, 1.000000000000000000, 0.9238795325112867385, 1.000000000000000000, 0.9238795325112867385, 1.000000000000000000, 0.9238795325112867385, 1.000000000000000000, 0.9238795325112867385, 1.000000000000000000, 0.9238795325112867385, 1.000000000000000000, 0.9238795325112867385, 1.000000000000000000, 0.9238795325112867385, 1.000000000000000000, 0.9238795325112867385, 1.000000000000000000, 0.9238795325112867385, 1.000000000000000000, 0.9238795325112867385, 1.000000000000000000, 0.9238795325112867385, 1.000000000000000000, 0.9238795325112867385, 1.000000000000000000, 0.9238795325112867385, 1.000000000000000000, 0.9238795325112867385, 1.000000000000000000, 0.9238795325112867385, 1.000000000000000000, 0.9238795325112867385, 1.000000000000000000, 0.9238795325112867385, 1.000000000000000000, 0.9238795325112867385, 1.000000000000000000, 0.9238795325112867385, 1.000000000000000000, 0.9238795325112867385, 1.000000000000000000, 0.9238795325112867385, 1.000000000000000000, 0.9238795325112867385, 1.000000000000000000, 0.9238795325112867385, 1.000000000000000000, 0.9324258078851886955, 0.9848264816800353927 ) ) 
 REPRESENTATION_ITEM ( '' )  );
#24966=CARTESIAN_POINT ( 'NONE',  ( 204.2950502721270425, 33.11210937608393579, -9.295050272127046043 ) ) ;
#24968=CARTESIAN_POINT ( 'NONE',  ( 187.9105827276678156, 49.99999999943695173, -11.59823041029156165 ) ) ;
#24974=CARTESIAN_POINT ( 'NONE',  ( 5.622872871577912157, 38.86679687500001279, 13.57481594606301023 ) ) ;
#24975=VECTOR ( 'NONE', #17474, 1000.000000000000000 ) ;
#24977=CARTESIAN_POINT ( 'NONE',  ( 130.0000000000000000, 38.76757812608393294, -13.14518615778179544 ) ) ;
#24978=CARTESIAN_POINT ( 'NONE',  ( -13.14518615778179189, 37.62656250108393152, 5.444914386472304635 ) ) ;
#24979=CARTESIAN_POINT ( 'NONE',  ( 2.414731522848535132E-15, 32.81445312608393294, 13.14518615778179544 ) ) ;
#24981=CIRCLE ( 'NONE', #404, 11.57481594606304398 ) ;
#24989=CARTESIAN_POINT ( 'NONE',  ( 99.99999999999995737, 83.43750000136560629, -4.458734125000016313 ) ) ;
#24990=CARTESIAN_POINT ( 'NONE',  ( -9.598844408820458085, 38.61875000216787157, -9.598844408820458085 ) ) ;
#24992=CARTESIAN_POINT ( 'NONE',  ( 208.1451861577818079, 37.03125000108393294, -5.444914386472297529 ) ) ;
#24994=EDGE_CURVE ( 'NONE', #4636, #25739, #1136, .T. ) ;
#24997=DIRECTION ( 'NONE',  ( -0.000000000000000000, -1.000000000000000000, -0.000000000000000000 ) ) ;
#24998=DIRECTION ( 'NONE',  ( -0.000000000000000000, 1.000000000000000000, -0.000000000000000000 ) ) ;
#25002=ORIENTED_EDGE ( 'NONE', *, *, #19217, .F. ) ;
#25004=CARTESIAN_POINT ( 'NONE',  ( 68.75563826565991121, 31.58960998161716560, -13.14518615778179900 ) ) ;
#25009=CARTESIAN_POINT ( 'NONE',  ( 204.2950502721270425, 34.10429687608393579, -9.295050272127046043 ) ) ;
#25011=ORIENTED_EDGE ( 'NONE', *, *, #4466, .F. ) ;
#25014=CARTESIAN_POINT ( 'NONE',  ( 95.27063293749995410, 79.84375000068280315, -1.387778780781445676E-14 ) ) ;
#25015=CARTESIAN_POINT ( 'NONE',  ( 116.4251840539369596, 37.13046875216787868, 0.000000000000000000 ) ) ;
#25018=CARTESIAN_POINT ( 'NONE',  ( 195.0000000000000000, 38.17226562608394147, -13.14518615778179544 ) ) ;
#25019=ADVANCED_FACE ( 'NONE', ( #20368 ), #15273, .T. ) ;
#25022=CARTESIAN_POINT ( 'NONE',  ( 120.8198241863519939, 55.00000000000000000, -15.00000000000000000 ) ) ;
#25024=CARTESIAN_POINT ( 'NONE',  ( -1.021803718759902280, 36.00000000000000711, 13.11239906893438878 ) ) ;
#25025=CARTESIAN_POINT ( 'NONE',  ( 70.44491438647230552, 33.36015625108393579, -13.14518615778179900 ) ) ;
#25026=FILL_AREA_STYLE ('',( #25156 ) ) ;
#25029=CARTESIAN_POINT ( 'NONE',  ( 1.662435489736055498E-15, -7.395377635281828788, -13.57481594606304398 ) ) ;
#25030=CARTESIAN_POINT ( 'NONE',  ( 0.7238719380229381439, 53.51529642094862993, 14.99999999999999645 ) ) ;
#25031=CARTESIAN_POINT ( 'NONE',  ( 124.3771271284221314, 33.70742187500000142, -13.57481594606304753 ) ) ;
#25032=ADVANCED_FACE ( 'NONE', ( #4656 ), #22043, .F. ) ;
#25039=CARTESIAN_POINT ( 'NONE',  ( 124.5550856135277087, 31.67343750108393863, -13.14518615778179900 ) ) ;
#25040=CARTESIAN_POINT ( 'NONE',  ( 55.40115559117954547, 32.26875000216787726, -9.598844408820458085 ) ) ;
#25041=CARTESIAN_POINT ( 'NONE',  ( 59.37712712842213136, 36.98164062716787015, -13.57481594606304753 ) ) ;
#25042=CARTESIAN_POINT ( 'NONE',  ( -13.14518615778179544, 37.37851562608393863, 0.000000000000000000 ) ) ;
#25046=AXIS2_PLACEMENT_3D ( 'NONE', #7662, #6535, #6128 ) ;
#25048=CARTESIAN_POINT ( 'NONE',  ( 181.8548138422181921, 31.87187500108393223, 5.444914386472304635 ) ) ;
#25053=LINE ( 'NONE', #27345, #16330 ) ;
#25054=LINE ( 'NONE', #2827, #4680 ) ;
#25065=CARTESIAN_POINT ( 'NONE',  ( 71.94442639331153089, 31.55306875057403104, -11.16113171639042356 ) ) ;
#25068=CARTESIAN_POINT ( 'NONE',  ( 13.57481594606304576, 33.45937499999999432, -1.662435489736055892E-15 ) ) ;
#25070=CARTESIAN_POINT ( 'NONE',  ( 130.0000000000000000, 35.39414062608393863, 13.14518615778179544 ) ) ;
#25074=CARTESIAN_POINT ( 'NONE',  ( 104.4587341249999639, 83.93750000136560629, -1.442382525525748735E-14 ) ) ;
#25078=CARTESIAN_POINT ( 'NONE',  ( 195.0000000000000000, 32.41757812608393863, -13.14518615778179544 ) ) ;
#25079=CARTESIAN_POINT ( 'NONE',  ( -5.622872871577873077, 39.36289062716787157, -13.57481594606304753 ) ) ;
#25080=ORIENTED_EDGE ( 'NONE', *, *, #5487, .F. ) ;
#25084=CARTESIAN_POINT ( 'NONE',  ( 181.4251840539369596, 32.41757812716787157, 5.622872871577880183 ) ) ;
#25085=CARTESIAN_POINT ( 'NONE',  ( 9.598844408820456309, 36.83281250216787583, -9.598844408820458085 ) ) ;
#25087=CIRCLE ( 'NONE', #4148, 11.57481594606304398 ) ;
#25089=CARTESIAN_POINT ( 'NONE',  ( 94.99999999999995737, 80.18750000273119838, 2.071067811865466624 ) ) ;
#25093=CARTESIAN_POINT ( 'NONE',  ( 204.5988444088204403, 39.90859374999999432, -9.598844408820458085 ) ) ;
#25097=DIRECTION ( 'NONE',  ( -0.000000000000000000, 1.000000000000000000, -0.000000000000000000 ) ) ;
#25098=AXIS2_PLACEMENT_3D ( 'NONE', #7658, #24629, #7081 ) ;
#25103=CARTESIAN_POINT ( 'NONE',  ( -13.14518615778179189, 32.86406250108393579, 5.444914386472304635 ) ) ;
#25104=ORIENTED_EDGE ( 'NONE', *, *, #10185, .T. ) ;
#25105=CARTESIAN_POINT ( 'NONE',  ( 2.493653234604083739E-15, 38.02343749999999289, 13.57481594606304576 ) ) ;
#25106=CARTESIAN_POINT ( 'NONE',  ( 181.8548138422182205, 34.20351562608393436, 0.000000000000000000 ) ) ;
#25107=ORIENTED_EDGE ( 'NONE', *, *, #18158, .F. ) ;
#25108=CARTESIAN_POINT ( 'NONE',  ( 198.1146977455429692, 53.90847045361284984, -15.00000000000000000 ) ) ;
#25110=ADVANCED_FACE ( 'NONE', ( #18036 ), #7054, .T. ) ;
#25116=CARTESIAN_POINT ( 'NONE',  ( 13.14518615778179544, 38.76757812608393294, -1.609821015232357215E-15 ) ) ;
#25117=CARTESIAN_POINT ( 'NONE',  ( 5.444914386472297529, 40.50390625108394005, -13.14518615778179900 ) ) ;
#25119=CARTESIAN_POINT ( 'NONE',  ( -9.598844408820458085, 36.23750000216787726, -9.598844408820458085 ) ) ;
#25120=CARTESIAN_POINT ( 'NONE',  ( -8.312177448680279460E-16, 36.93203125216787441, -13.57481594606304576 ) ) ;
#25123=( BOUNDED_CURVE ( )  B_SPLINE_CURVE ( 2, ( #24300, #15738, #4641 ),
 .UNSPECIFIED., .F., .T. ) 
 B_SPLINE_CURVE_WITH_KNOTS ( ( 3, 3 ),
 ( 0.5208333333333332593, 0.5249747582430949189 ),
 .UNSPECIFIED. ) 
 CURVE ( )  GEOMETRIC_REPRESENTATION_ITEM ( )  RATIONAL_B_SPLINE_CURVE ( ( 1.000000000000000888, 0.9697362687807569159, 0.9635368518655843539 ) ) 
 REPRESENTATION_ITEM ( '' )  );
#25124=CARTESIAN_POINT ( 'NONE',  ( 95.54126587499996504, 81.68750000136559208, -1.387778780781445676E-14 ) ) ;
#25126=CARTESIAN_POINT ( 'NONE',  ( 78.57481594606305464, 39.11484375216787157, -1.662435489736055892E-15 ) ) ;
#25128=ORIENTED_EDGE ( 'NONE', *, *, #27941, .F. ) ;
#25133=CARTESIAN_POINT ( 'NONE',  ( 116.4251840539369738, 39.56132812716787583, 5.622872871577880183 ) ) ;
#25137=CARTESIAN_POINT ( 'NONE',  ( 51.85481384221820633, 36.78320312608393294, 0.000000000000000000 ) ) ;
#25139=CARTESIAN_POINT ( 'NONE',  ( 195.0000000000000000, 31.82226562608393650, -13.14518615778179544 ) ) ;
#25142=CARTESIAN_POINT ( 'NONE',  ( 0.8389268692830608165, 53.50081894914648473, -14.99999999999999822 ) ) ;
#25143=CARTESIAN_POINT ( 'NONE',  ( 65.00000000000000000, 36.03906250000000000, -13.57481594606304576 ) ) ;
#25144=AXIS2_PLACEMENT_3D ( 'NONE', #28201, #28062, #17498 ) ;
#25145=CARTESIAN_POINT ( 'NONE',  ( 135.6228728715778686, 39.26367187716787299, -13.57481594606304753 ) ) ;
#25148=CARTESIAN_POINT ( 'NONE',  ( 208.1451861577817795, 38.71796875108393721, 5.444914386472293977 ) ) ;
#25149=ORIENTED_EDGE ( 'NONE', *, *, #9674, .F. ) ;
#25152=CARTESIAN_POINT ( 'NONE',  ( 195.0000000000000000, 50.00000000000000000, -2.255140518769849538E-14 ) ) ;
#25153=CARTESIAN_POINT ( 'NONE',  ( 9.598844408820456309, 38.32109374999999574, -9.598844408820458085 ) ) ;
#25154=CARTESIAN_POINT ( 'NONE',  ( 101.8468681455907046, 83.75000000136560629, 4.458734124999987891 ) ) ;
#25155=CARTESIAN_POINT ( 'NONE',  ( 74.59884440882045453, 40.00781250216787299, -9.598844408820458085 ) ) ;
#25156=FILL_AREA_STYLE_COLOUR ( '', #1792 ) ;
#25158=CARTESIAN_POINT ( 'NONE',  ( -5.622872871577964560, 38.46992187499999005, -13.57481594606295339 ) ) ;
#25159=SPHERICAL_SURFACE ( 'NONE', #27588, 5.000000000000000000 ) ;
#25160=CARTESIAN_POINT ( 'NONE',  ( 65.00000000000000000, 40.80156249999999574, -13.57481594606304576 ) ) ;
#25161=CARTESIAN_POINT ( 'NONE',  ( 120.4011555911795455, 33.75703124999999005, -9.598844408820458085 ) ) ;
#25164=EDGE_LOOP ( 'NONE', ( #24467, #9180, #23984 ) ) ;
#25170=CARTESIAN_POINT ( 'NONE',  ( 120.7049497278729575, 39.06523437608392868, -9.295050272127046043 ) ) ;
#25171=CARTESIAN_POINT ( 'NONE',  ( 78.14518615778179367, 39.31328125108392868, 5.444914386472293977 ) ) ;
#25172=ORIENTED_EDGE ( 'NONE', *, *, #7608, .T. ) ;
#25174=CARTESIAN_POINT ( 'NONE',  ( 61.86382637865181522, 36.00000000000000711, 12.79489613812742910 ) ) ;
#25175=CARTESIAN_POINT ( 'NONE',  ( 13.14518615778179544, 40.15664062608393436, -1.609821015232357215E-15 ) ) ;
#25178=CARTESIAN_POINT ( 'NONE',  ( 183.7351811978183207, 35.99999999999997158, 6.828991891054760011 ) ) ;
#25180=DIRECTION ( 'NONE',  ( 0.000000000000000000, -0.000000000000000000, 1.000000000000000000 ) ) ;
#25182=CARTESIAN_POINT ( 'NONE',  ( 0.000000000000000000, -7.395377635281828788, 0.000000000000000000 ) ) ;
#25184=EDGE_CURVE ( 'NONE', #18668, #11161, #22978, .T. ) ;
#25187=DIRECTION ( 'NONE',  ( -0.000000000000000000, 1.000000000000000000, -0.000000000000000000 ) ) ;
#25191=EDGE_LOOP ( 'NONE', ( #18671, #14544, #6473, #28098 ) ) ;
#25199=CARTESIAN_POINT ( 'NONE',  ( 99.99999999999995737, 83.43750000136560629, -4.458734125000016313 ) ) ;
#25200=CARTESIAN_POINT ( 'NONE',  ( 78.14518615778179367, 40.30546875108393579, 5.444914386472293977 ) ) ;
#25202=CARTESIAN_POINT ( 'NONE',  ( 65.00000000000000000, -7.395377635281828788, -7.517135062566165128E-15 ) ) ;
#25206=CARTESIAN_POINT ( 'NONE',  ( 130.0000000000000000, 35.79101562608394005, -13.14518615778179544 ) ) ;
#25207=ORIENTED_EDGE ( 'NONE', *, *, #7608, .F. ) ;
#25209=CARTESIAN_POINT ( 'NONE',  ( 96.84719886470459471, 81.56250000136559208, 3.152801135295355994 ) ) ;
#25211=CARTESIAN_POINT ( 'NONE',  ( 51.42518405393695957, 40.30546875216787583, 0.000000000000000000 ) ) ;
#25214=CARTESIAN_POINT ( 'NONE',  ( -13.57481594606304576, 39.56132812716787583, 5.622872871577880183 ) ) ;
#25219=CARTESIAN_POINT ( 'NONE',  ( 200.4449143864723055, 39.21406250108392300, 13.14518615778179189 ) ) ;
#25223=CARTESIAN_POINT ( 'NONE',  ( 130.0000000000000000, 36.78320312608393294, 13.14518615778179544 ) ) ;
#25225=CARTESIAN_POINT ( 'NONE',  ( 139.5988444088204403, 37.52734375000000000, -9.598844408820458085 ) ) ;
#25228=CARTESIAN_POINT ( 'NONE',  ( 189.5550856135277229, 32.16953125108393152, 13.14518615778179722 ) ) ;
#25237=CARTESIAN_POINT ( 'NONE',  ( 13.14518615778179900, 34.84843750108393579, -5.444914386472297529 ) ) ;
#25238=ORIENTED_EDGE ( 'NONE', *, *, #9714, .F. ) ;
#25239=CARTESIAN_POINT ( 'NONE',  ( 99.99999999999995737, 85.00000000000000000, 4.999999999999990230 ) ) ;
#25242=VERTEX_POINT ( 'NONE', #15753 ) ;
#25243=CARTESIAN_POINT ( 'NONE',  ( 200.4449143864723055, 33.65781250108393152, 13.14518615778179189 ) ) ;
#25245=CARTESIAN_POINT ( 'NONE',  ( 201.4508793426651039, 50.00000000106953735, -11.97362904075546197 ) ) ;
#25247=VERTEX_POINT ( 'NONE', #22327 ) ;
#25250=FACE_OUTER_BOUND ( 'NONE', #22548, .T. ) ;
#25252=CARTESIAN_POINT ( 'NONE',  ( -9.295050272127046043, 36.68398437608393436, -9.295050272127046043 ) ) ;
#25253=CARTESIAN_POINT ( 'NONE',  ( -5.444914386472297529, 32.46718750108393436, -13.14518615778179900 ) ) ;
#25254=AXIS2_PLACEMENT_3D ( 'NONE', #16344, #24092, #4567 ) ;
#25257=CARTESIAN_POINT ( 'NONE',  ( 78.57481594606305464, 38.22187499999999716, -1.662435489736055892E-15 ) ) ;
#25260=CARTESIAN_POINT ( 'NONE',  ( 95.54126587499996504, 81.75000000136560629, 1.846868145590724986 ) ) ;
#25266=EDGE_CURVE ( 'NONE', #2842, #4709, #2130, .T. ) ;
#25271=AXIS2_PLACEMENT_3D ( 'NONE', #4402, #13057, #6664 ) ;
#25275=CARTESIAN_POINT ( 'NONE',  ( 55.70494972787295751, 39.06523437608392868, -9.295050272127046043 ) ) ;
#25276=ORIENTED_EDGE ( 'NONE', *, *, #15137, .T. ) ;
#25278=CARTESIAN_POINT ( 'NONE',  ( 185.7049497278729575, 31.92148437608393508, -9.295050272127046043 ) ) ;
#25281=CARTESIAN_POINT ( 'NONE',  ( 65.00000000000000000, 40.40468749999999432, 13.57481594606304576 ) ) ;
#25284=CARTESIAN_POINT ( 'NONE',  ( 135.6228728715779539, 36.58476562716786873, 13.57481594606297115 ) ) ;
#25285=CARTESIAN_POINT ( 'NONE',  ( 116.4251840539369454, 33.90585937716787868, -5.622872871577873077 ) ) ;
#25286=( BOUNDED_CURVE ( )  B_SPLINE_CURVE ( 2, ( #16528, #9828, #25085, #21087, #18938, #10228, #1434, #5710, #3285 ),
 .UNSPECIFIED., .F., .F. ) 
 B_SPLINE_CURVE_WITH_KNOTS ( ( 3, 2, 2, 2, 3 ),
 ( 0.3541666666666666852, 0.3645833333333332593, 0.3749999999999998890, 0.3854166666666665741, 0.3958333333333331483 ),
 .UNSPECIFIED. ) 
 CURVE ( )  GEOMETRIC_REPRESENTATION_ITEM ( )  RATIONAL_B_SPLINE_CURVE ( ( 1.000000000000000000, 0.9238795325112867385, 1.000000000000000000, 0.9238795325112867385, 1.000000000000000000, 0.9238795325112867385, 1.000000000000000000, 0.9238795325112879597, 0.9999999999999987788 ) ) 
 REPRESENTATION_ITEM ( '' )  );
#25289=CARTESIAN_POINT ( 'NONE',  ( 195.0000000000000000, 39.36289062608393152, 13.14518615778179544 ) ) ;
#25294=CARTESIAN_POINT ( 'NONE',  ( 99.99999999999995737, 83.18750000136560629, -4.458734125000016313 ) ) ;
#25299=CARTESIAN_POINT ( 'NONE',  ( 96.46446609406721961, 80.87500000000000000, -3.535533905932755072 ) ) ;
#25301=DIRECTION ( 'NONE',  ( 0.000000000000000000, -1.000000000000000000, 0.000000000000000000 ) ) ;
#25306=CARTESIAN_POINT ( 'NONE',  ( 99.99999999999995737, 84.75000000000000000, -5.000000000000018652 ) ) ;
#25310=CARTESIAN_POINT ( 'NONE',  ( 130.0000000000000000, 31.62382812608393579, -13.14518615778179544 ) ) ;
#25311=CARTESIAN_POINT ( 'NONE',  ( 51.85481384221820633, 35.79101562608393294, 0.000000000000000000 ) ) ;
#25312=CARTESIAN_POINT ( 'NONE',  ( 52.26160984214450878, 36.00000000000000000, 3.273369733618432864 ) ) ;
#25313=CARTESIAN_POINT ( 'NONE',  ( 13.14518615778179900, 36.13828125108393863, 5.444914386472293977 ) ) ;
#25314=CARTESIAN_POINT ( 'NONE',  ( -14.99999999999999822, 80.00000000000000000, 15.00000000000000000 ) ) ;
#25317=CARTESIAN_POINT ( 'NONE',  ( 116.4251840539369596, 40.20624999999999005, 0.000000000000000000 ) ) ;
#25319=CARTESIAN_POINT ( 'NONE',  ( -13.14518615778179189, 37.42812500108393436, 5.444914386472304635 ) ) ;
#25321=LINE ( 'NONE', #10189, #6988 ) ;
#25324=CYLINDRICAL_SURFACE ( 'NONE', #2787, 3.000000000000004441 ) ;
#25335=CARTESIAN_POINT ( 'NONE',  ( 103.1528011352953342, 79.81250000136559208, 3.152801135295355106 ) ) ;
#25336=CARTESIAN_POINT ( 'NONE',  ( 65.00000000000000000, 39.75976562608394005, -13.14518615778179544 ) ) ;
#25337=( BOUNDED_CURVE ( )  B_SPLINE_CURVE ( 2, ( #26242, #12540, #166, #19680, #6700, #17110, #27829, #19542, #23544 ),
 .UNSPECIFIED., .F., .F. ) 
 B_SPLINE_CURVE_WITH_KNOTS ( ( 3, 2, 2, 2, 3 ),
 ( 0.1875000000000001388, 0.1979166666666667407, 0.2083333333333333703, 0.2187499999999999722, 0.2291666666666665741 ),
 .UNSPECIFIED. ) 
 CURVE ( )  GEOMETRIC_REPRESENTATION_ITEM ( )  RATIONAL_B_SPLINE_CURVE ( ( 0.9999999999999990008, 0.9238795325112877377, 1.000000000000000000, 0.9238795325112867385, 1.000000000000000000, 0.9238795325112867385, 1.000000000000000000, 0.9238795325112872936, 0.9999999999999994449 ) ) 
 REPRESENTATION_ITEM ( '' )  );
#25339=LINE ( 'NONE', #5825, #24594 ) ;
#25341=ADVANCED_FACE ( 'NONE', ( #20891 ), #10034, .T. ) ;
#25342=DIRECTION ( 'NONE',  ( 0.000000000000000000, -1.000000000000000000, -0.000000000000000000 ) ) ;
#25345=CARTESIAN_POINT ( 'NONE',  ( 124.5550856135277087, 31.87187500108393223, -13.14518615778179900 ) ) ;
#25346=ORIENTED_EDGE ( 'NONE', *, *, #19063, .F. ) ;
#25348=EDGE_CURVE ( 'NONE', #16116, #19665, #12438, .T. ) ;
#25350=CARTESIAN_POINT ( 'NONE',  ( 101.8468681455906903, 80.12500000136560629, -4.458734125000016313 ) ) ;
#25352=CARTESIAN_POINT ( 'NONE',  ( 116.8548138422182063, 39.80937500108392868, 5.444914386472304635 ) ) ;
#25353=CARTESIAN_POINT ( 'NONE',  ( 55.40115559117954547, 38.02343750216788010, 9.598844408820459861 ) ) ;
#25357=CARTESIAN_POINT ( 'NONE',  ( 13.57481594606304576, 39.90859375216787441, -1.662435489736055892E-15 ) ) ;
#25363=CARTESIAN_POINT ( 'NONE',  ( 202.1713913950166273, 31.30502190640808990, -11.52591746582321974 ) ) ;
#25366=CARTESIAN_POINT ( 'NONE',  ( 120.7049497278729575, 39.06523437608392868, 9.295050272127047819 ) ) ;
#25367=CARTESIAN_POINT ( 'NONE',  ( 13.14518615778179900, 32.36796875108393579, 5.444914386472293977 ) ) ;
#25371=CARTESIAN_POINT ( 'NONE',  ( 208.5748159460630688, 38.22187499999999716, -1.662435489736055892E-15 ) ) ;
#25372=EDGE_CURVE ( 'NONE', #2214, #24582, #23869, .T. ) ;
#25376=CARTESIAN_POINT ( 'NONE',  ( 78.14518615778179367, 38.51953125108393294, 5.444914386472293977 ) ) ;
#25380=( BOUNDED_CURVE ( )  B_SPLINE_CURVE ( 2, ( #26340, #24198, #13049, #20066, #17919 ),
 .UNSPECIFIED., .F., .F. ) 
 B_SPLINE_CURVE_WITH_KNOTS ( ( 3, 2, 3 ),
 ( 0.000000000000000000, 0.02500000000000002220, 0.05000000000000004441 ),
 .UNSPECIFIED. ) 
 CURVE ( )  GEOMETRIC_REPRESENTATION_ITEM ( )  RATIONAL_B_SPLINE_CURVE ( ( 1.000000000000000000, 0.9238795325112867385, 1.000000000000000000, 0.9238795325112866275, 1.000000000000000222 ) ) 
 REPRESENTATION_ITEM ( '' )  );
#25381=CARTESIAN_POINT ( 'NONE',  ( 200.6228728715777549, 39.66054687500000142, 13.57481594606318076 ) ) ;
#25383=CARTESIAN_POINT ( 'NONE',  ( -8.312177448680279460E-16, 40.00781250000000000, -13.57481594606304576 ) ) ;
#25385=CARTESIAN_POINT ( 'NONE',  ( 103.1528011352953342, 84.06250000136560629, 3.152801135295355106 ) ) ;
#25386=EDGE_CURVE ( 'NONE', #27020, #15564, #3488, .T. ) ;
#25391=CARTESIAN_POINT ( 'NONE',  ( 190.1415007095349381, 49.99999999891522151, -12.70434618648777381 ) ) ;
#25393=ORIENTED_EDGE ( 'NONE', *, *, #26948, .T. ) ;
#25396=CARTESIAN_POINT ( 'NONE',  ( 189.3771271284219608, 38.86679687716787868, 13.57481594606290720 ) ) ;
#25397=ADVANCED_FACE ( 'NONE', ( #2769 ), #22293, .T. ) ;
#25400=CARTESIAN_POINT ( 'NONE',  ( 135.4449143864723339, 39.71015625108393010, -13.14518615778179722 ) ) ;
#25401=CARTESIAN_POINT ( 'NONE',  ( -13.14518615778179544, 39.95820312608393010, 0.000000000000000000 ) ) ;
#25402=ORIENTED_EDGE ( 'NONE', *, *, #7577, .T. ) ;
#25403=CARTESIAN_POINT ( 'NONE',  ( 74.59884440882045453, 37.52734375000000000, -9.598844408820458085 ) ) ;
#25405=CARTESIAN_POINT ( 'NONE',  ( 2.493653234604083739E-15, 37.32890625216786873, 13.57481594606304576 ) ) ;
#25409=CARTESIAN_POINT ( 'NONE',  ( 101.8468681455907046, 81.37500000136563472, -4.458734125000016313 ) ) ;
#25411=CARTESIAN_POINT ( 'NONE',  ( -9.295050272127046043, 39.85898437608393152, -9.295050272127046043 ) ) ;
#25412=EDGE_CURVE ( 'NONE', #1080, #3022, #9449, .T. ) ;
#25413=CARTESIAN_POINT ( 'NONE',  ( 58.88343976028321691, 54.66944451632674173, 14.99999999999998224 ) ) ;
#25416=DIRECTION ( 'NONE',  ( 0.000000000000000000, -1.000000000000000000, 0.000000000000000000 ) ) ;
#25419=LINE ( 'NONE', #21007, #19429 ) ;
#25420=CARTESIAN_POINT ( 'NONE',  ( 219.9999999999999716, 75.00000000000000000, -10.00000000000000000 ) ) ;
#25422=CARTESIAN_POINT ( 'NONE',  ( 65.00000000000000000, 36.98164062608393721, 13.14518615778179544 ) ) ;
#25423=CARTESIAN_POINT ( 'NONE',  ( 94.99999999999995737, 79.56250000136559208, -1.387778780781445676E-14 ) ) ;
#25424=AXIS2_PLACEMENT_3D ( 'NONE', #1958, #28035, #2242 ) ;
#25429=DIRECTION ( 'NONE',  ( 0.000000000000000000, -1.000000000000000000, -0.000000000000000000 ) ) ;
#25431=CARTESIAN_POINT ( 'NONE',  ( 124.3771271284221314, 33.31054687716787299, 13.57481594606304753 ) ) ;
#25434=CARTESIAN_POINT ( 'NONE',  ( 181.8548138422182205, 37.57695312608393579, 0.000000000000000000 ) ) ;
#25435=VERTEX_POINT ( 'NONE', #15995 ) ;
#25444=VECTOR ( 'NONE', #2412, 999.9999999999998863 ) ;
#25445=CARTESIAN_POINT ( 'NONE',  ( 7.065634988760085555, 36.00000000000000000, 11.21307450592249033 ) ) ;
#25446=CARTESIAN_POINT ( 'NONE',  ( 195.0000000000000000, 50.00000000000000000, -2.255140518769849538E-14 ) ) ;
#25448=ORIENTED_EDGE ( 'NONE', *, *, #25372, .F. ) ;
#25453=CARTESIAN_POINT ( 'NONE',  ( 130.0000000000000000, 39.75976562608394005, -13.14518615778179544 ) ) ;
#25454=CARTESIAN_POINT ( 'NONE',  ( 55.70494972787295751, 37.27929687608393294, -9.295050272127046043 ) ) ;
#25455=DIRECTION ( 'NONE',  ( 0.8660254037844418162, -0.4999999999999947264, -0.000000000000000000 ) ) ;
#25456=CARTESIAN_POINT ( 'NONE',  ( 9.295050272127046043, 34.69960937608393436, -9.295050272127046043 ) ) ;
#25457=CARTESIAN_POINT ( 'NONE',  ( 181.8975291782780914, 36.00000000000001421, -1.608626461598034130 ) ) ;
#25459=CARTESIAN_POINT ( 'NONE',  ( 55.40115559117954547, 37.72578124999999005, -9.598844408820458085 ) ) ;
#25460=LINE ( 'NONE', #3799, #11705 ) ;
#25461=EDGE_CURVE ( 'NONE', #778, #22877, #11451, .T. ) ;
#25462=CARTESIAN_POINT ( 'NONE',  ( -20.00000000000000355, 75.00000000000000000, -14.99999999999999822 ) ) ;
#25463=MECHANICAL_DESIGN_GEOMETRIC_PRESENTATION_REPRESENTATION('',(#2261),#24551);
#25464=CARTESIAN_POINT ( 'NONE',  ( 9.295050272127046043, 38.66835937608393436, -9.295050272127046043 ) ) ;
#25465=CARTESIAN_POINT ( 'NONE',  ( 143.4541126562309046, 35.99999999999999289, 0.6772748633552372333 ) ) ;
#25467=FACE_OUTER_BOUND ( 'NONE', #26435, .T. ) ;
#25478=CARTESIAN_POINT ( 'NONE',  ( 95.54126587499996504, 81.43750000136559208, -1.387778780781445676E-14 ) ) ;
#25479=CARTESIAN_POINT ( 'NONE',  ( 59.55508561352770158, 36.93203125108394147, 13.14518615778179722 ) ) ;
#25485=CARTESIAN_POINT ( 'NONE',  ( 120.7049497278729575, 32.91367187608393152, 9.295050272127047819 ) ) ;
#25486=ORIENTED_EDGE ( 'NONE', *, *, #20539, .F. ) ;
#25487=CARTESIAN_POINT ( 'NONE',  ( 1.417506129906585004E-15, 36.00000000000000000, -11.57481594606304398 ) ) ;
#25491=CARTESIAN_POINT ( 'NONE',  ( 51.42518405393695957, 36.38632812716788578, 5.622872871577880183 ) ) ;
#25493=CARTESIAN_POINT ( 'NONE',  ( -8.312177448680279460E-16, 34.55078125216787299, -13.57481594606304576 ) ) ;
#25498=CARTESIAN_POINT ( 'NONE',  ( 200.4449143864723055, 38.42031250108393436, 13.14518615778179189 ) ) ;
#25501=CARTESIAN_POINT ( 'NONE',  ( 116.8548138422182205, 38.22187500108393721, 5.444914386472304635 ) ) ;
#25503=( BOUNDED_CURVE ( )  B_SPLINE_CURVE ( 2, ( #11534, #18259, #14105, #22395, #26967, #16106, #5013, #3295, #9836 ),
 .UNSPECIFIED., .F., .F. ) 
 B_SPLINE_CURVE_WITH_KNOTS ( ( 3, 2, 2, 2, 3 ),
 ( 0.3541666666666666852, 0.3645833333333332593, 0.3749999999999998890, 0.3854166666666665741, 0.3958333333333331483 ),
 .UNSPECIFIED. ) 
 CURVE ( )  GEOMETRIC_REPRESENTATION_ITEM ( )  RATIONAL_B_SPLINE_CURVE ( ( 1.000000000000000000, 0.9238795325112867385, 1.000000000000000000, 0.9238795325112867385, 1.000000000000000000, 0.9238795325112867385, 1.000000000000000000, 0.9238795325112879597, 0.9999999999999987788 ) ) 
 REPRESENTATION_ITEM ( '' )  );
#25506=DIRECTION ( 'NONE',  ( -0.000000000000000000, 1.000000000000000000, -0.000000000000000000 ) ) ;
#25508=CARTESIAN_POINT ( 'NONE',  ( 195.0000000000000000, 37.22968749999999716, 13.57481594606304576 ) ) ;
#25511=CARTESIAN_POINT ( 'NONE',  ( 70.44491438647230552, 40.00781250108393294, 13.14518615778179189 ) ) ;
#25517=CARTESIAN_POINT ( 'NONE',  ( 13.57481594606304931, 39.75976562499999289, 5.622872871577869525 ) ) ;
#25518=CARTESIAN_POINT ( 'NONE',  ( 143.1451861577818079, 40.35507812608393863, -1.609821015232357215E-15 ) ) ;
#25520=ORIENTED_EDGE ( 'NONE', *, *, #23099, .F. ) ;
#25521=CARTESIAN_POINT ( 'NONE',  ( 104.4587341249999781, 82.12500000136560629, 1.846868145590721655 ) ) ;
#25522=DIRECTION ( 'NONE',  ( -0.000000000000000000, 1.000000000000000000, -0.000000000000000000 ) ) ;
#25524=APPLICATION_CONTEXT ( 'automotive_design' ) ;
#25526=CARTESIAN_POINT ( 'NONE',  ( 126.2025481310420076, 54.08938259242987101, -15.00000000000000178 ) ) ;
#25531=CARTESIAN_POINT ( 'NONE',  ( 189.3771271284221314, 37.27929687716787299, 13.57481594606304753 ) ) ;
#25535=CARTESIAN_POINT ( 'NONE',  ( 195.3286002765670446, 53.49358765999039633, 14.99999999999994671 ) ) ;
#25536=CARTESIAN_POINT ( 'NONE',  ( 139.2950502721270425, 38.07304687608393579, -9.295050272127046043 ) ) ;
#25537=CARTESIAN_POINT ( 'NONE',  ( 13.14518615778179544, 33.01289062608393010, -1.609821015232357215E-15 ) ) ;
#25539=CARTESIAN_POINT ( 'NONE',  ( 55.40115559117954547, 37.72578124999999005, -9.598844408820458085 ) ) ;
#25542=DIRECTION ( 'NONE',  ( -0.000000000000000000, 1.000000000000000000, -0.000000000000000000 ) ) ;
#25546=CARTESIAN_POINT ( 'NONE',  ( 98.15313185440923860, 83.50000000136560629, -4.458734125000016313 ) ) ;
#25548=CARTESIAN_POINT ( 'NONE',  ( 9.295050272127047819, 38.66835937608393436, 9.295050272127046043 ) ) ;
#25550=CARTESIAN_POINT ( 'NONE',  ( 61.13458562458681200, 54.10683252460148651, 14.99999999999998046 ) ) ;
#25551=ORIENTED_EDGE ( 'NONE', *, *, #6983, .F. ) ;
#25555=CARTESIAN_POINT ( 'NONE',  ( 208.1451861577818079, 36.38632812608393863, -1.609821015232357215E-15 ) ) ;
#25559=CARTESIAN_POINT ( 'NONE',  ( 78.14518615778179367, 39.56132812608393579, -1.609821015232357215E-15 ) ) ;
#25560=CARTESIAN_POINT ( 'NONE',  ( 71.11656023971681861, 54.66944451632674884, -15.00000000000000000 ) ) ;
#25563=CARTESIAN_POINT ( 'NONE',  ( 116.4251840539369596, 37.82499999999999574, 0.000000000000000000 ) ) ;
#25564=CARTESIAN_POINT ( 'NONE',  ( 196.8875287258763649, 53.66306546785488507, 14.99999999999994671 ) ) ;
#25565=CARTESIAN_POINT ( 'NONE',  ( 143.5748159460630404, 35.09648437716787583, 5.622872871577869525 ) ) ;
#25566=CARTESIAN_POINT ( 'NONE',  ( 130.0000000000000000, 36.00000000000000000, -1.503427012513233026E-14 ) ) ;
#25569=CARTESIAN_POINT ( 'NONE',  ( 208.1451861577818079, 38.76757812608393294, -1.609821015232357215E-15 ) ) ;
#25570=EDGE_LOOP ( 'NONE', ( #3309, #24324 ) ) ;
#25571=ORIENTED_EDGE ( 'NONE', *, *, #16104, .T. ) ;
#25573=CARTESIAN_POINT ( 'NONE',  ( 0.000000000000000000, 50.00000000000000000, 0.000000000000000000 ) ) ;
#25575=DIRECTION ( 'NONE',  ( -0.000000000000000000, 1.000000000000000000, -0.000000000000000000 ) ) ;
#25579=LINE ( 'NONE', #14313, #16203 ) ;
#25580=CARTESIAN_POINT ( 'NONE',  ( 96.46446609406721961, 82.87500000000000000, -3.535533905932755072 ) ) ;
#25581=CARTESIAN_POINT ( 'NONE',  ( 133.8783852973911905, 32.03609435653363136, -13.57481594606304576 ) ) ;
#25586=CARTESIAN_POINT ( 'NONE',  ( 133.7556399192858976, 31.58960996655074993, -13.14518615778179544 ) ) ;
#25587=CARTESIAN_POINT ( 'NONE',  ( 65.00000000000000000, 37.97382812608393721, -13.14518615778179544 ) ) ;
#25588=CARTESIAN_POINT ( 'NONE',  ( 208.1451861577818079, 32.21914062608393436, -1.609821015232357215E-15 ) ) ;
#25590=CARTESIAN_POINT ( 'NONE',  ( -9.295050272127044266, 36.68398437608392726, 9.295050272127047819 ) ) ;
#25592=CARTESIAN_POINT ( 'NONE',  ( 195.2703369776649254, 36.00000000000000000, 13.14949859323919412 ) ) ;
#25593=CARTESIAN_POINT ( 'NONE',  ( 130.0000000000000000, 40.40468749999999432, 13.57481594606304576 ) ) ;
#25594=CARTESIAN_POINT ( 'NONE',  ( 9.295050272127047819, 39.26367187608393294, 9.295050272127046043 ) ) ;
#25595=CARTESIAN_POINT ( 'NONE',  ( 3.039397050802530753, 53.88964894337311762, 14.99999999999999645 ) ) ;
#25605=CIRCLE ( 'NONE', #25144, 13.57481594606304398 ) ;
#25608=CARTESIAN_POINT ( 'NONE',  ( 98.15313185440925281, 81.62500000136560629, 4.458734124999987891 ) ) ;
#25609=CARTESIAN_POINT ( 'NONE',  ( 51.85481384221820633, 38.42031250108393436, 5.444914386472304635 ) ) ;
#25612=( BOUNDED_CURVE ( )  B_SPLINE_CURVE ( 2, ( #2095, #19474, #10627, #26317, #10763, #4655, #98, #24034, #11179 ),
 .UNSPECIFIED., .F., .F. ) 
 B_SPLINE_CURVE_WITH_KNOTS ( ( 3, 2, 2, 2, 3 ),
 ( 0.1458333333333336757, 0.1562500000000002776, 0.1666666666666669072, 0.1770833333333335369, 0.1875000000000001388 ),
 .UNSPECIFIED. ) 
 CURVE ( )  GEOMETRIC_REPRESENTATION_ITEM ( )  RATIONAL_B_SPLINE_CURVE ( ( 0.9999999999999975575, 0.9238795325112891810, 1.000000000000000000, 0.9238795325112867385, 1.000000000000000000, 0.9238795325112867385, 1.000000000000000000, 0.9238795325112857393, 1.000000000000001110 ) ) 
 REPRESENTATION_ITEM ( '' )  );
#25615=DIRECTION ( 'NONE',  ( 0.000000000000000000, 0.000000000000000000, 1.000000000000000000 ) ) ;
#25617=CARTESIAN_POINT ( 'NONE',  ( 116.8548138422182205, 32.02070312608393010, 0.000000000000000000 ) ) ;
#25623=CARTESIAN_POINT ( 'NONE',  ( 120.7049497278729575, 40.45429687608393721, -9.295050272127046043 ) ) ;
#25624=CARTESIAN_POINT ( 'NONE',  ( 51.42518405393695957, 38.66835937716786731, -5.622872871577873077 ) ) ;
#25626=CARTESIAN_POINT ( 'NONE',  ( 13.57481594606304576, 35.93984375216787441, -1.662435489736055892E-15 ) ) ;
#25627=ORIENTED_EDGE ( 'NONE', *, *, #1184, .T. ) ;
#25631=CARTESIAN_POINT ( 'NONE',  ( 181.8548138422181921, 38.91640625108393436, -5.444914386472297529 ) ) ;
#25632=CARTESIAN_POINT ( 'NONE',  ( 124.5550856135277087, 38.02343750108394005, -13.14518615778179722 ) ) ;
#25633=DIRECTION ( 'NONE',  ( 0.000000000000000000, 0.000000000000000000, 1.000000000000000000 ) ) ;
#25638=CARTESIAN_POINT ( 'NONE',  ( 200.6228728715778686, 37.57695312499998863, -13.57481594606304753 ) ) ;
#25640=CARTESIAN_POINT ( 'NONE',  ( 125.2199608011490284, 36.00000000000002842, 12.25280873422854278 ) ) ;
#25642=CARTESIAN_POINT ( 'NONE',  ( 51.85481384221820633, 39.80937500108392868, 5.444914386472304635 ) ) ;
#25644=DIRECTION ( 'NONE',  ( 0.000000000000000000, 1.000000000000000000, 0.000000000000000000 ) ) ;
#25647=CARTESIAN_POINT ( 'NONE',  ( 13.57481594606304753, 40.65273437499998721, -5.622872871577873077 ) ) ;
#25648=CARTESIAN_POINT ( 'NONE',  ( 139.2950502721270425, 39.66054687608393436, -9.295050272127046043 ) ) ;
#25650=CARTESIAN_POINT ( 'NONE',  ( 95.54126587499996504, 84.68750000136560629, -1.387778780781445676E-14 ) ) ;
#25656=CARTESIAN_POINT ( 'NONE',  ( 65.00000000000000000, 34.99726562608393721, -13.14518615778179544 ) ) ;
#25664=CARTESIAN_POINT ( 'NONE',  ( 181.4251840539369596, 37.92421875216787441, 0.000000000000000000 ) ) ;
#25666=CARTESIAN_POINT ( 'NONE',  ( 65.00000000000000000, 36.13828125216787157, -13.57481594606304576 ) ) ;
#25667=CARTESIAN_POINT ( 'NONE',  ( 198.8030543732578224, 54.09082899096448926, 14.99999999999994671 ) ) ;
#25668=CARTESIAN_POINT ( 'NONE',  ( 135.4449143864723339, 38.91640625108393436, -13.14518615778179722 ) ) ;
#25669=CARTESIAN_POINT ( 'NONE',  ( 13.14518615778179900, 38.02343750108395426, -5.444914386472297529 ) ) ;
#25671=CARTESIAN_POINT ( 'NONE',  ( 65.00000000000000000, 38.42031249999999432, -13.57481594606304576 ) ) ;
#25674=EDGE_CURVE ( 'NONE', #2105, #6018, #19292, .T. ) ;
#25681=DIRECTION ( 'NONE',  ( 0.000000000000000000, 0.000000000000000000, 1.000000000000000000 ) ) ;
#25683=DIRECTION ( 'NONE',  ( 0.000000000000000000, 0.000000000000000000, -1.000000000000000000 ) ) ;
#25686=CARTESIAN_POINT ( 'NONE',  ( 97.92893218813451028, 82.31250000273122680, 4.999999999999989342 ) ) ;
#25690=CARTESIAN_POINT ( 'NONE',  ( 78.14518615778180788, 38.71796875108393721, 5.444914386472293977 ) ) ;
#25691=EDGE_CURVE ( 'NONE', #4294, #9852, #21134, .T. ) ;
#25692=CARTESIAN_POINT ( 'NONE',  ( 94.99999999999995737, 83.18750000273119838, 2.071067811865466624 ) ) ;
#25693=CARTESIAN_POINT ( 'NONE',  ( -13.57481594606304576, 39.41249999999999432, 0.000000000000000000 ) ) ;
#25696=AXIS2_PLACEMENT_3D ( 'NONE', #3372, #1662, #27740 ) ;
#25697=CARTESIAN_POINT ( 'NONE',  ( -9.180175813648018490, 55.00000000000000000, -15.00000000000000000 ) ) ;
#25698=CARTESIAN_POINT ( 'NONE',  ( 94.99999999999995737, 81.18750000273119838, 2.071067811865466624 ) ) ;
#25699=EDGE_CURVE ( 'NONE', #24259, #11568, #14325, .T. ) ;
#25700=CARTESIAN_POINT ( 'NONE',  ( 130.0000000000000000, 35.74140625216787015, 13.57481594606304576 ) ) ;
#25702=B_SPLINE_CURVE_WITH_KNOTS ( 'NONE', 3,
 ( #4705, #15804, #4851, #26074, #13221, #6543, #15223, #8972, #19661, #26222, #4422, #13515, #17519, #2715, #2572, #17660, #10950, #11375, #13076, #8829, #6681, #15367, #24083, #4559, #21953, #2431, #19803, #287, #26368, #16519, #20804 ),
 .UNSPECIFIED., .F., .F.,
 ( 4, 2, 2, 2, 2, 2, 2, 2, 2, 2, 1, 2, 2, 2, 2, 4 ),
 ( 0.000000000000000000, 0.001656255954913766690, 0.003312511909827533380, 0.004968767864741300069, 0.005796895842198182547, 0.006625023819655066759, 0.008281279774568852531, 0.009937535729482641772, 0.01325004763931021852, 0.01490630359422400603, 0.01656255954913779180, 0.01821881550405158104, 0.01987507145896536681, 0.02318758336879294182, 0.02484383932370672760, 0.02650009527862051337 ),
 .UNSPECIFIED. ) ;
#25703=CARTESIAN_POINT ( 'NONE',  ( 78.14518615778179367, 40.30546875108393579, 5.444914386472293977 ) ) ;
#25704=DIRECTION ( 'NONE',  ( -0.000000000000000000, 1.000000000000000000, -0.000000000000000000 ) ) ;
#25705=CARTESIAN_POINT ( 'NONE',  ( 181.8548138422181921, 36.03906250108394005, 5.444914386472304635 ) ) ;
#25706=ORIENTED_EDGE ( 'NONE', *, *, #6175, .F. ) ;
#25710=DIRECTION ( 'NONE',  ( 0.000000000000000000, 1.000000000000000000, 3.469446951953611231E-16 ) ) ;
#25712=CARTESIAN_POINT ( 'NONE',  ( 95.54126587499996504, 83.43750000136560629, -1.387778780781445676E-14 ) ) ;
#25715=AXIS2_PLACEMENT_3D ( 'NONE', #14954, #1738, #17387 ) ;
#25716=CARTESIAN_POINT ( 'NONE',  ( 11.20653150213496296, 36.00000000000000000, 7.323573988461853368 ) ) ;
#25718=ORIENTED_EDGE ( 'NONE', *, *, #18399, .F. ) ;
#25723=CARTESIAN_POINT ( 'NONE',  ( 143.1451861577818079, 35.54296875108394715, 5.444914386472293977 ) ) ;
#25724=CARTESIAN_POINT ( 'NONE',  ( 55.70494972787295751, 36.68398437608392726, 9.295050272127047819 ) ) ;
#25725=ADVANCED_FACE ( 'NONE', ( #3887 ), #21275, .T. ) ;
#25726=CARTESIAN_POINT ( 'NONE',  ( 198.7556399192858976, 31.58960996655074993, -13.14518615778179544 ) ) ;
#25727=CARTESIAN_POINT ( 'NONE',  ( 57.93163431200125757, 35.99999999999999289, 11.09140360074102993 ) ) ;
#25728=CARTESIAN_POINT ( 'NONE',  ( -13.14518615778179900, 36.53515625108392584, -5.444914386472297529 ) ) ;
#25729=CARTESIAN_POINT ( 'NONE',  ( 131.6025331306099986, 53.60343507247939954, -15.00000000000000000 ) ) ;
#25730=DIRECTION ( 'NONE',  ( 0.000000000000000000, 0.000000000000000000, -1.000000000000000000 ) ) ;
#25731=CARTESIAN_POINT ( 'NONE',  ( -18.00000000000000711, 52.00000000000000711, -12.99999999999999822 ) ) ;
#25733=CARTESIAN_POINT ( 'NONE',  ( -5.444914386472297529, 37.22968750108393721, -13.14518615778179900 ) ) ;
#25739=VERTEX_POINT ( 'NONE', #8715 ) ;
#25743=ORIENTED_EDGE ( 'NONE', *, *, #26938, .F. ) ;
#25748=DIRECTION ( 'NONE',  ( 0.000000000000000000, -0.000000000000000000, 1.000000000000000000 ) ) ;
#25749=CARTESIAN_POINT ( 'NONE',  ( 103.1528011352953342, 84.31250000136560629, -3.152801135295383084 ) ) ;
#25750=CARTESIAN_POINT ( 'NONE',  ( 78.14518615778179367, 38.76757812608393294, -1.609821015232357215E-15 ) ) ;
#25752=CARTESIAN_POINT ( 'NONE',  ( 5.444914386472297529, 40.30546875108393579, -13.14518615778179722 ) ) ;
#25756=CARTESIAN_POINT ( 'NONE',  ( 116.4251840539369596, 40.99999999999999289, 0.000000000000000000 ) ) ;
#25758=CARTESIAN_POINT ( 'NONE',  ( 65.00000000000000000, 50.00000000000000000, -7.517135062566165128E-15 ) ) ;
#25761=CARTESIAN_POINT ( 'NONE',  ( 130.0000000000000000, 35.98945312608393010, 13.14518615778179544 ) ) ;
#25762=CARTESIAN_POINT ( 'NONE',  ( 78.57481594606304043, 36.68398437716788152, 5.622872871577869525 ) ) ;
#25764=CARTESIAN_POINT ( 'NONE',  ( 9.598844408820459861, 34.25312500216787015, 9.598844408820456309 ) ) ;
#25765=AXIS2_PLACEMENT_3D ( 'NONE', #10909, #8509, #10632 ) ;
#25766=EDGE_LOOP ( 'NONE', ( #27118, #4920, #23176, #15261, #6373, #17131, #17868, #251, #326, #25238, #2492, #20019, #19342, #26093, #11551 ) ) ;
#25769=CARTESIAN_POINT ( 'NONE',  ( 208.1451861577817795, 37.82500000108392868, -5.444914386472297529 ) ) ;
#25771=CARTESIAN_POINT ( 'NONE',  ( 124.5550856135277087, 39.61093750108393152, -13.14518615778179722 ) ) ;
#25776=CARTESIAN_POINT ( 'NONE',  ( 51.42518405393695957, 36.98164062499999005, -5.622872871577872189 ) ) ;
#25779=CARTESIAN_POINT ( 'NONE',  ( 208.5748159460630120, 36.58476562499999574, 5.622872871577869525 ) ) ;
#25780=CARTESIAN_POINT ( 'NONE',  ( 51.42518405393695957, 39.36289062499999858, -5.622872871577872189 ) ) ;
#25782=CARTESIAN_POINT ( 'NONE',  ( 65.00000000000000000, 38.37070312608393152, 13.14518615778179544 ) ) ;
#25784=DIRECTION ( 'NONE',  ( 0.000000000000000000, 0.000000000000000000, -1.000000000000000000 ) ) ;
#25786=AXIS2_PLACEMENT_3D ( 'NONE', #3031, #1050, #7434 ) ;
#25787=CARTESIAN_POINT ( 'NONE',  ( 116.4251840539369596, 39.41249999999999432, 0.000000000000000000 ) ) ;
#25788=CARTESIAN_POINT ( 'NONE',  ( -13.57481594606304753, 40.15664062500000142, -5.622872871577873077 ) ) ;
#25789=CARTESIAN_POINT ( 'NONE',  ( 139.2950502721270425, 39.46210937608393721, 9.295050272127046043 ) ) ;
#25790=EDGE_LOOP ( 'NONE', ( #7035, #14924, #16208, #27960 ) ) ;
#25791=CARTESIAN_POINT ( 'NONE',  ( 96.84719886470459471, 84.56250000136560629, -3.152801135295383084 ) ) ;
#25792=CARTESIAN_POINT ( 'NONE',  ( 130.0000000000000000, 39.71015625216787015, 13.57481594606304576 ) ) ;
#25794=CYLINDRICAL_SURFACE ( 'NONE', #12934, 5.000000000000000888 ) ;
#25795=CARTESIAN_POINT ( 'NONE',  ( 78.14518615778179367, 34.74921875108395142, 5.444914386472293977 ) ) ;
#25798=CARTESIAN_POINT ( 'NONE',  ( 133.8654143754132235, 54.10683252460147941, -15.00000000000000000 ) ) ;
#25800=ORIENTED_EDGE ( 'NONE', *, *, #22015, .T. ) ;
#25803=CARTESIAN_POINT ( 'NONE',  ( 181.4251840539369596, 37.97382812716787726, 5.622872871577880183 ) ) ;
#25806=DIRECTION ( 'NONE',  ( -0.000000000000000000, 1.000000000000000000, -0.000000000000000000 ) ) ;
#25808=CARTESIAN_POINT ( 'NONE',  ( 139.2950502721270425, 40.25585937608393294, 9.295050272127046043 ) ) ;
#25809=CARTESIAN_POINT ( 'NONE',  ( 13.14518615778179900, 37.13046875108393863, 5.444914386472293977 ) ) ;
#25811=ORIENTED_EDGE ( 'NONE', *, *, #21552, .F. ) ;
#25812=CARTESIAN_POINT ( 'NONE',  ( 139.2950502721270425, 36.28710937608393294, -9.295050272127046043 ) ) ;
#25813=CARTESIAN_POINT ( 'NONE',  ( 55.40115559117954547, 37.13046874999999147, 9.598844408820459861 ) ) ;
#25819=CYLINDRICAL_SURFACE ( 'NONE', #21364, 5.000000000000004441 ) ;
#25820=AXIS2_PLACEMENT_3D ( 'NONE', #22204, #11344, #19634 ) ;
#25823=CARTESIAN_POINT ( 'NONE',  ( -8.049105076161786076E-16, 38.17226562608394147, -13.14518615778179544 ) ) ;
#25825=ORIENTED_EDGE ( 'NONE', *, *, #17318, .F. ) ;
#25827=CYLINDRICAL_SURFACE ( 'NONE', #2539, 5.000000000000000888 ) ;
#25829=CARTESIAN_POINT ( 'NONE',  ( -9.180175813647995398, 55.00000000000000000, 15.00000000000000000 ) ) ;
#25830=CARTESIAN_POINT ( 'NONE',  ( 65.00000000000000000, 36.43593749999999432, 13.57481594606304576 ) ) ;
#25831=( BOUNDED_SURFACE ( )  B_SPLINE_SURFACE ( 1, 2, ( 
 ( #25650, #1455, #25791, #22977, #21106, #18958, #12244, #14396, #6134, #21391, #25385, #4001, #1594, #14664, #7854, #1312, #1868, #27666, #14799, #23113, #12666, #20972, #16686, #27395, #23523, #3588, #10534, #8128, #16825, #8263, #23385, #19240, #3442, #21247, #19098, #9982, #27940, #27807, #20835, #5999, #16949, #25521, #14257, #3857, #12517, #18692, #16549, #8399, #23249, #17088, #14536, #1728, #10110, #12109, #7987, #18824, #27531, #3726, #10392, #4701, #15220, #23797, #4420, #8826, #6410, #19799, #9110, #13073, #4275, #17804, #26218, #6268, #13362, #12933, #10806, #14943, #8969, #19658, #17515, #21666, #23663 ),
 ( #2143, #19520, #4138, #17657, #140, #6678, #26072, #2288, #2567, #6822, #26364, #15364, #12801, #21522, #22089, #24078, #15079, #2, #4556, #13217, #19376, #8686, #2001, #283, #15513, #23938, #21811, #17376, #10668, #17232, #25935, #6541, #24222, #11229, #10946, #28080, #19946, #424, #8544, #21950, #2428, #11089, #2979, #18233, #17944, #7386, #1147, #9534, #2843, #24652, #24358, #16079, #26508, #570, #5125, #9673, #13655, #9814, #6964, #13792, #11654, #24504, #26654, #18376, #5415, #9388, #16230, #22514, #26942, #20092, #13511, #14083, #20377, #27081, #7102, #24929, #4990, #712, #11370, #7533, #9252 ) ),
 .UNSPECIFIED., .F., .F., .F. ) 
 B_SPLINE_SURFACE_WITH_KNOTS ( ( 2, 2 ),
 ( 3, 2, 2, 2, 2, 2, 2, 2, 2, 2, 2, 2, 2, 2, 2, 2, 2, 2, 2, 2, 2, 2, 2, 2, 2, 2, 2, 2, 2, 2, 2, 2, 2, 2, 2, 2, 2, 2, 2, 2, 3 ),
 ( 0.000000000000000000, 1.000000000000000000 ),
 ( 0.000000000000000000, 0.02500000000000000139, 0.05000000000000000278, 0.07499999999999999722, 0.1000000000000000056, 0.1250000000000000000, 0.1499999999999999944, 0.1749999999999999889, 0.2000000000000000111, 0.2250000000000000056, 0.2500000000000000000, 0.2750000000000000222, 0.2999999999999999889, 0.3250000000000000111, 0.3499999999999999778, 0.3750000000000000000, 0.4000000000000000222, 0.4249999999999999889, 0.4500000000000000111, 0.4749999999999999778, 0.5000000000000000000, 0.5250000000000000222, 0.5500000000000000444, 0.5749999999999999556, 0.5999999999999999778, 0.6250000000000000000, 0.6500000000000000222, 0.6750000000000000444, 0.6999999999999999556, 0.7249999999999999778, 0.7500000000000000000, 0.7750000000000000222, 0.8000000000000000444, 0.8249999999999999556, 0.8499999999999999778, 0.8750000000000000000, 0.9000000000000000222, 0.9250000000000000444, 0.9499999999999999556, 0.9749999999999999778, 1.000000000000000000 ),
 .UNSPECIFIED. ) 
 GEOMETRIC_REPRESENTATION_ITEM ( )  RATIONAL_B_SPLINE_SURFACE ( (
 ( 1.000000000000000000, 0.9238795325112867385, 1.000000000000000000, 0.9238795325112867385, 1.000000000000000000, 0.9238795325112867385, 1.000000000000000000, 0.9238795325112867385, 1.000000000000000000, 0.9238795325112867385, 1.000000000000000000, 0.9238795325112867385, 1.000000000000000000, 0.9238795325112867385, 1.000000000000000000, 0.9238795325112867385, 1.000000000000000000, 0.9238795325112867385, 1.000000000000000000, 0.9238795325112867385, 1.000000000000000000, 0.9238795325112867385, 1.000000000000000000, 0.9238795325112867385, 1.000000000000000000, 0.9238795325112867385, 1.000000000000000000, 0.9238795325112867385, 1.000000000000000000, 0.9238795325112867385, 1.000000000000000000, 0.9238795325112867385, 1.000000000000000000, 0.9238795325112867385, 1.000000000000000000, 0.9238795325112867385, 1.000000000000000000, 0.9238795325112867385, 1.000000000000000000, 0.9238795325112867385, 1.000000000000000000, 0.9238795325112867385, 1.000000000000000000, 0.9238795325112867385, 1.000000000000000000, 0.9238795325112867385, 1.000000000000000000, 0.9238795325112867385, 1.000000000000000000, 0.9238795325112867385, 1.000000000000000000, 0.9238795325112867385, 1.000000000000000000, 0.9238795325112867385, 1.000000000000000000, 0.9238795325112867385, 1.000000000000000000, 0.9238795325112867385, 1.000000000000000000, 0.9238795325112867385, 1.000000000000000000, 0.9238795325112867385, 1.000000000000000000, 0.9238795325112867385, 1.000000000000000000, 0.9238795325112867385, 1.000000000000000000, 0.9238795325112867385, 1.000000000000000000, 0.9238795325112867385, 1.000000000000000000, 0.9238795325112867385, 1.000000000000000000, 0.9238795325112867385, 1.000000000000000000, 0.9238795325112867385, 1.000000000000000000, 0.9238795325112867385, 1.000000000000000000, 0.9238795325112867385, 1.000000000000000000),
 ( 1.000000000000000000, 0.9238795325112867385, 1.000000000000000000, 0.9238795325112867385, 1.000000000000000000, 0.9238795325112867385, 1.000000000000000000, 0.9238795325112867385, 1.000000000000000000, 0.9238795325112867385, 1.000000000000000000, 0.9238795325112867385, 1.000000000000000000, 0.9238795325112867385, 1.000000000000000000, 0.9238795325112867385, 1.000000000000000000, 0.9238795325112867385, 1.000000000000000000, 0.9238795325112867385, 1.000000000000000000, 0.9238795325112867385, 1.000000000000000000, 0.9238795325112867385, 1.000000000000000000, 0.9238795325112867385, 1.000000000000000000, 0.9238795325112867385, 1.000000000000000000, 0.9238795325112867385, 1.000000000000000000, 0.9238795325112867385, 1.000000000000000000, 0.9238795325112867385, 1.000000000000000000, 0.9238795325112867385, 1.000000000000000000, 0.9238795325112867385, 1.000000000000000000, 0.9238795325112867385, 1.000000000000000000, 0.9238795325112867385, 1.000000000000000000, 0.9238795325112867385, 1.000000000000000000, 0.9238795325112867385, 1.000000000000000000, 0.9238795325112867385, 1.000000000000000000, 0.9238795325112867385, 1.000000000000000000, 0.9238795325112867385, 1.000000000000000000, 0.9238795325112867385, 1.000000000000000000, 0.9238795325112867385, 1.000000000000000000, 0.9238795325112867385, 1.000000000000000000, 0.9238795325112867385, 1.000000000000000000, 0.9238795325112867385, 1.000000000000000000, 0.9238795325112867385, 1.000000000000000000, 0.9238795325112867385, 1.000000000000000000, 0.9238795325112867385, 1.000000000000000000, 0.9238795325112867385, 1.000000000000000000, 0.9238795325112867385, 1.000000000000000000, 0.9238795325112867385, 1.000000000000000000, 0.9238795325112867385, 1.000000000000000000, 0.9238795325112867385, 1.000000000000000000, 0.9238795325112867385, 1.000000000000000000) ) ) 
 REPRESENTATION_ITEM ( '' )  SURFACE ( )  );
#25832=CARTESIAN_POINT ( 'NONE',  ( 208.1451861577818079, 40.15664062608393436, -1.609821015232357215E-15 ) ) ;
#25833=ORIENTED_EDGE ( 'NONE', *, *, #21171, .F. ) ;
#25834=DIRECTION ( 'NONE',  ( 0.000000000000000000, 0.000000000000000000, 1.000000000000000000 ) ) ;
#25836=CARTESIAN_POINT ( 'NONE',  ( 61.96060294919745814, 53.88964894337311051, -14.99999999999999822 ) ) ;
#25839=CARTESIAN_POINT ( 'NONE',  ( -2.276146844545014591, 51.46995505939283788, -14.99999999999999822 ) ) ;
#25841=CARTESIAN_POINT ( 'NONE',  ( 120.4011555911795455, 33.85625000216787583, -9.598844408820458085 ) ) ;
#25842=CARTESIAN_POINT ( 'NONE',  ( 70.44491438647230552, 40.50390625108394005, -13.14518615778179900 ) ) ;
#25845=CARTESIAN_POINT ( 'NONE',  ( 208.1451861577817795, 33.26093750108393721, -5.444914386472297529 ) ) ;
#25846=ORIENTED_EDGE ( 'NONE', *, *, #6873, .F. ) ;
#25852=EDGE_CURVE ( 'NONE', #23414, #1457, #5492, .T. ) ;
#25854=CARTESIAN_POINT ( 'NONE',  ( 51.85481384221820633, 40.55351562608393579, 0.000000000000000000 ) ) ;
#25855=CARTESIAN_POINT ( 'NONE',  ( 95.54126587499996504, 82.37500000136563472, -1.846868145590750077 ) ) ;
#25856=CARTESIAN_POINT ( 'NONE',  ( 200.4449143864723055, 37.62656250108393152, 13.14518615778179189 ) ) ;
#25857=CARTESIAN_POINT ( 'NONE',  ( 139.5988444088204687, 39.80937500216786873, 9.598844408820456309 ) ) ;
#25858=CARTESIAN_POINT ( 'NONE',  ( 181.4251840539369596, 40.65273437608393436, 0.000000000000000000 ) ) ;
#25862=VECTOR ( 'NONE', #24751, 1000.000000000000000 ) ;
#25868=( BOUNDED_CURVE ( )  B_SPLINE_CURVE ( 2, ( #1918, #6183, #3773, #28129, #21438 ),
 .UNSPECIFIED., .F., .T. ) 
 B_SPLINE_CURVE_WITH_KNOTS ( ( 3, 2, 3 ),
 ( 0.000000000000000000, 0.01041666666666679446, 0.02083333333333358892 ),
 .UNSPECIFIED. ) 
 CURVE ( )  GEOMETRIC_REPRESENTATION_ITEM ( )  RATIONAL_B_SPLINE_CURVE ( ( 1.000000000000000000, 0.9238795325112867385, 1.000000000000000000, 0.9238795325112848511, 1.000000000000001776 ) ) 
 REPRESENTATION_ITEM ( '' )  );
#25870=CARTESIAN_POINT ( 'NONE',  ( 124.5550856135277087, 35.34453125108393579, 13.14518615778179722 ) ) ;
#25871=CARTESIAN_POINT ( 'NONE',  ( 74.29505027212704249, 34.50117187608393010, 9.295050272127046043 ) ) ;
#25872=CARTESIAN_POINT ( 'NONE',  ( 208.1451861577818079, 37.18007812608393436, -1.609821015232357215E-15 ) ) ;
#25875=CARTESIAN_POINT ( 'NONE',  ( 5.444914386472302859, 34.45156250108393436, 13.14518615778179189 ) ) ;
#25876=CARTESIAN_POINT ( 'NONE',  ( 134.9250267836615080, 49.99999999893073266, -12.67776588291936690 ) ) ;
#25877=CARTESIAN_POINT ( 'NONE',  ( 187.2214956318787245, 35.99999999999997868, 10.60546543669477515 ) ) ;
#25880=CARTESIAN_POINT ( 'NONE',  ( -13.14518615778179189, 39.01562500108393294, 5.444914386472304635 ) ) ;
#25884=CARTESIAN_POINT ( 'NONE',  ( 63.86123188289986530, 50.00000000043846882, 13.56816686242530601 ) ) ;
#25885=ORIENTED_EDGE ( 'NONE', *, *, #5672, .T. ) ;
#25887=CARTESIAN_POINT ( 'NONE',  ( 78.04200858115000017, 36.00000000000000000, -3.640726557253424200 ) ) ;
#25888=ORIENTED_EDGE ( 'NONE', *, *, #21004, .F. ) ;
#25889=CARTESIAN_POINT ( 'NONE',  ( 120.4011555911795455, 40.90078124999999432, -9.598844408820458085 ) ) ;
#25895=CARTESIAN_POINT ( 'NONE',  ( 104.4587341249999781, 82.12500000136560629, 1.846868145590721655 ) ) ;
#25896=CARTESIAN_POINT ( 'NONE',  ( 78.14518615778179367, 37.22968750108393721, -5.444914386472297529 ) ) ;
#25898=CARTESIAN_POINT ( 'NONE',  ( -9.295050272127046043, 39.66054687608393436, -9.295050272127046043 ) ) ;
#25899=CARTESIAN_POINT ( 'NONE',  ( 195.0000000000000000, 36.00000000000000000, -2.255140518769849538E-14 ) ) ;
#25900=CARTESIAN_POINT ( 'NONE',  ( -18.00000000000000355, 52.00000000000000711, 13.00000000000000178 ) ) ;
#25902=CARTESIAN_POINT ( 'NONE',  ( 135.6228728715778971, 40.45429687500001137, 13.57481594606304576 ) ) ;
#25903=EDGE_LOOP ( 'NONE', ( #27674, #9398, #9183, #8497 ) ) ;
#25905=DIRECTION ( 'NONE',  ( 0.000000000000000000, 0.000000000000000000, 1.000000000000000000 ) ) ;
#25906=CARTESIAN_POINT ( 'NONE',  ( 99.99999999999995737, 80.18750000136559208, -4.458734125000016313 ) ) ;
#25907=CARTESIAN_POINT ( 'NONE',  ( 120.7049497278729575, 35.89023437608393152, 9.295050272127047819 ) ) ;
#25908=CARTESIAN_POINT ( 'NONE',  ( 55.40115559117954547, 36.23750000216787726, -9.598844408820458085 ) ) ;
#25909=CARTESIAN_POINT ( 'NONE',  ( 102.0710678118654187, 83.31249999999998579, 5.000000000000011546 ) ) ;
#25910=CARTESIAN_POINT ( 'NONE',  ( -8.312177448680279460E-16, 36.93203125216787441, -13.57481594606304576 ) ) ;
#25914=( BOUNDED_CURVE ( )  B_SPLINE_CURVE ( 2, ( #21568, #27706, #21711, #25692, #10290, #8170, #8445, #14986, #8303 ),
 .UNSPECIFIED., .F., .F. ) 
 B_SPLINE_CURVE_WITH_KNOTS ( ( 3, 2, 2, 2, 3 ),
 ( 0.1500000000000001332, 0.1750000000000001554, 0.2000000000000001776, 0.2250000000000001998, 0.2500000000000002220 ),
 .UNSPECIFIED. ) 
 CURVE ( )  GEOMETRIC_REPRESENTATION_ITEM ( )  RATIONAL_B_SPLINE_CURVE ( ( 0.9999999999999995559, 0.9238795325112871826, 1.000000000000000000, 0.9238795325112867385, 1.000000000000000000, 0.9238795325112867385, 1.000000000000000000, 0.9238795325112860723, 1.000000000000000666 ) ) 
 REPRESENTATION_ITEM ( '' )  );
#25915=CARTESIAN_POINT ( 'NONE',  ( 208.1451861577818079, 38.56914062608393579, -1.609821015232357215E-15 ) ) ;
#25917=CARTESIAN_POINT ( 'NONE',  ( 120.7049497278729575, 36.48554687608393721, -9.295050272127046043 ) ) ;
#25919=CARTESIAN_POINT ( 'NONE',  ( 214.9999999999999716, 80.00000000000000000, -15.00000000000000000 ) ) ;
#25920=CARTESIAN_POINT ( 'NONE',  ( 130.3247243111959790, 53.49346745874645137, 14.99999999999996447 ) ) ;
#25924=CARTESIAN_POINT ( 'NONE',  ( 208.5748159460630688, 39.01562500000000000, -1.662435489736055892E-15 ) ) ;
#25925=LINE ( 'NONE', #17220, #11276 ) ;
#25927=CARTESIAN_POINT ( 'NONE',  ( 78.14518615778179367, 37.77539062608393294, -1.609821015232357215E-15 ) ) ;
#25932=CARTESIAN_POINT ( 'NONE',  ( 9.598844408820456309, 35.14609374999999858, -9.598844408820458085 ) ) ;
#25935=CARTESIAN_POINT ( 'NONE',  ( 96.46446609406721961, 83.12500000000000000, 3.535533905932727539 ) ) ;
#25939=CARTESIAN_POINT ( 'NONE',  ( 208.5748159460630688, 37.52734375216787299, -1.662435489736055892E-15 ) ) ;
#25940=CARTESIAN_POINT ( 'NONE',  ( 78.14518615778179367, 34.00507812608393721, -1.609821015232357215E-15 ) ) ;
#25941=EDGE_LOOP ( 'NONE', ( #13830, #23253, #26759, #11301 ) ) ;
#25945=CARTESIAN_POINT ( 'NONE',  ( 219.9999999999999716, 55.00000000000000000, 14.99999999999994316 ) ) ;
#25947=CARTESIAN_POINT ( 'NONE',  ( 208.5748159460630688, 36.73359375216787015, -1.662435489736055892E-15 ) ) ;
#25948=( BOUNDED_CURVE ( )  B_SPLINE_CURVE ( 2, ( #7212, #13904, #11483, #7356, #22632, #2815, #11767, #5524, #20491 ),
 .UNSPECIFIED., .F., .T. ) 
 B_SPLINE_CURVE_WITH_KNOTS ( ( 3, 2, 2, 2, 3 ),
 ( 0.8500000000000007550, 0.8750000000000008882, 0.9000000000000009104, 0.9250000000000009326, 0.9500000000000009548 ),
 .UNSPECIFIED. ) 
 CURVE ( )  GEOMETRIC_REPRESENTATION_ITEM ( )  RATIONAL_B_SPLINE_CURVE ( ( 0.9999999999999976685, 0.9238795325112890700, 1.000000000000000000, 0.9238795325112867385, 1.000000000000000000, 0.9238795325112867385, 1.000000000000000000, 0.9238795325112837409, 1.000000000000003109 ) ) 
 REPRESENTATION_ITEM ( '' )  );
#25950=CARTESIAN_POINT ( 'NONE',  ( -20.00000000000000355, 55.00000000000000000, -10.00000000000000000 ) ) ;
#25952=CARTESIAN_POINT ( 'NONE',  ( 120.7049497278729575, 39.85898437608393152, -9.295050272127046043 ) ) ;
#25953=CARTESIAN_POINT ( 'NONE',  ( -5.444914386472297529, 39.01562500108394005, -13.14518615778179900 ) ) ;
#25955=CARTESIAN_POINT ( 'NONE',  ( 120.7049497278729575, 33.50898437608393010, 9.295050272127047819 ) ) ;
#25956=CARTESIAN_POINT ( 'NONE',  ( 59.37712712842213136, 35.59257812499999574, 13.57481594606304753 ) ) ;
#25957=DIRECTION ( 'NONE',  ( 0.000000000000000000, 0.000000000000000000, 1.000000000000000000 ) ) ;
#25959=CARTESIAN_POINT ( 'NONE',  ( 196.6855116490827697, 35.99999999999997868, 13.05727741351676130 ) ) ;
#25964=DIRECTION ( 'NONE',  ( 0.000000000000000000, 0.000000000000000000, 1.000000000000000000 ) ) ;
#25972=LINE ( 'NONE', #23835, #16588 ) ;
#25973=EDGE_CURVE ( 'NONE', #26178, #4636, #4563, .T. ) ;
#25974=CARTESIAN_POINT ( 'NONE',  ( 208.1451861577817795, 37.72578125108393721, 5.444914386472293977 ) ) ;
#25975=VERTEX_POINT ( 'NONE', #15894 ) ;
#25979=ORIENTED_EDGE ( 'NONE', *, *, #12250, .F. ) ;
#25984=CARTESIAN_POINT ( 'NONE',  ( 130.0000000000000000, 39.56132812608393579, -13.14518615778179544 ) ) ;
#25986=CARTESIAN_POINT ( 'NONE',  ( 104.9999999999999716, 81.68750000273119838, -2.071067811865491937 ) ) ;
#25988=AXIS2_PLACEMENT_3D ( 'NONE', #23703, #14842, #23840 ) ;
#25989=CARTESIAN_POINT ( 'NONE',  ( 189.5550856135277229, 34.25312500108393010, -13.14518615778179900 ) ) ;
#25994=CARTESIAN_POINT ( 'NONE',  ( 78.14518615778180788, 39.31328125108392868, 5.444914386472293977 ) ) ;
#25996=CARTESIAN_POINT ( 'NONE',  ( 208.1451861577818079, 38.56914062608393579, -1.609821015232357215E-15 ) ) ;
#26006=CARTESIAN_POINT ( 'NONE',  ( 120.7049497278729575, 36.08867187608393579, 9.295050272127047819 ) ) ;
#26007=CARTESIAN_POINT ( 'NONE',  ( 70.44491438647230552, 32.36796875108393579, -13.14518615778179900 ) ) ;
#26008=CARTESIAN_POINT ( 'NONE',  ( 185.7049497278729575, 37.47773437608393010, -9.295050272127046043 ) ) ;
#26011=CARTESIAN_POINT ( 'NONE',  ( -9.295050272127046043, 31.72304687608393081, -9.295050272127046043 ) ) ;
#26012=CARTESIAN_POINT ( 'NONE',  ( 133.8639252651224467, 54.10645156200379802, -14.99999999999999467 ) ) ;
#26016=CARTESIAN_POINT ( 'NONE',  ( -5.444914386472297529, 36.43593750108392726, -13.14518615778179900 ) ) ;
#26017=LINE ( 'NONE', #23882, #16084 ) ;
#26018=CARTESIAN_POINT ( 'NONE',  ( 104.9999999999999716, 79.68750000273119838, -2.071067811865491937 ) ) ;
#26019=CARTESIAN_POINT ( 'NONE',  ( 56.22739075386999730, 50.37415326813798089, 14.99999999999999112 ) ) ;
#26020=EDGE_LOOP ( 'NONE', ( #7593, #23008, #22192, #2364 ) ) ;
#26022=ORIENTED_EDGE ( 'NONE', *, *, #8955, .F. ) ;
#26027=CYLINDRICAL_SURFACE ( 'NONE', #25424, 3.000000000000004441 ) ;
#26028=CARTESIAN_POINT ( 'NONE',  ( 104.4587341249999639, 81.18750000136559208, -1.442382525525748735E-14 ) ) ;
#26029=CARTESIAN_POINT ( 'NONE',  ( 51.85481384221819923, 36.73359375108393010, -5.444914386472297529 ) ) ;
#26033=ORIENTED_EDGE ( 'NONE', *, *, #17472, .F. ) ;
#26034=CARTESIAN_POINT ( 'NONE',  ( 102.0710678118653618, 80.43750000273118417, 5.000000000000031086 ) ) ;
#26037=CARTESIAN_POINT ( 'NONE',  ( 143.5748159460630688, 36.63437499999999858, -1.662435489736055892E-15 ) ) ;
#26038=ORIENTED_EDGE ( 'NONE', *, *, #26373, .F. ) ;
#26042=CARTESIAN_POINT ( 'NONE',  ( 143.1451861577818079, 37.77539062608393294, -1.609821015232357215E-15 ) ) ;
#26044=CARTESIAN_POINT ( 'NONE',  ( 51.42518405393695957, 32.36796875216787583, 0.000000000000000000 ) ) ;
#26046=CARTESIAN_POINT ( 'NONE',  ( -13.57481594606304753, 36.28710937716787299, -5.622872871577873077 ) ) ;
#26047=EDGE_CURVE ( 'NONE', #2435, #10403, #14376, .T. ) ;
#26050=CARTESIAN_POINT ( 'NONE',  ( 208.1451861577817795, 36.93203125108394147, 5.444914386472293977 ) ) ;
#26051=CARTESIAN_POINT ( 'NONE',  ( 214.9999999999999716, 55.00000000000000000, -9.999999999999998224 ) ) ;
#26054=CARTESIAN_POINT ( 'NONE',  ( 189.3771271284220177, 37.77539062716787299, -13.57481594606295339 ) ) ;
#26061=CARTESIAN_POINT ( 'NONE',  ( 181.4251840539369596, 33.01289062500000426, -5.622872871577873077 ) ) ;
#26064=CARTESIAN_POINT ( 'NONE',  ( 55.70494972787295751, 34.30273437608393294, 9.295050272127047819 ) ) ;
#26066=CARTESIAN_POINT ( 'NONE',  ( 130.0000000000000000, 36.00000000000000000, -1.503427012513233026E-14 ) ) ;
#26069=CARTESIAN_POINT ( 'NONE',  ( 13.57481594606304576, 37.42812499999999432, -1.662435489736055892E-15 ) ) ;
#26070=CARTESIAN_POINT ( 'NONE',  ( -20.00000000000000000, 80.00000000000000000, 15.00000000000000178 ) ) ;
#26072=CARTESIAN_POINT ( 'NONE',  ( 103.5355339059327093, 84.62500000000000000, -3.535533905932755072 ) ) ;
#26074=CARTESIAN_POINT ( 'NONE',  ( 67.00729701006973471, 35.99999999999998579, -13.40042260803721419 ) ) ;
#26079=CARTESIAN_POINT ( 'NONE',  ( 55.70494972787295751, 34.30273437608393294, -9.295050272127046043 ) ) ;
#26082=ADVANCED_FACE ( 'NONE', ( #18336 ), #27043, .T. ) ;
#26088=CARTESIAN_POINT ( 'NONE',  ( 181.4251840539369596, 37.18007812716787441, 5.622872871577880183 ) ) ;
#26090=CARTESIAN_POINT ( 'NONE',  ( 51.63999894807758295, 40.42949218912590936, 0.000000000000000000 ) ) ;
#26091=CARTESIAN_POINT ( 'NONE',  ( 195.9830651850982406, 49.99999999949031348, 13.54930971656779626 ) ) ;
#26092=CARTESIAN_POINT ( 'NONE',  ( 208.5748159460630688, 39.90859375216787441, -1.662435489736055892E-15 ) ) ;
#26093=ORIENTED_EDGE ( 'NONE', *, *, #648, .T. ) ;
#26094=CARTESIAN_POINT ( 'NONE',  ( 2.414731522848535132E-15, 38.56914062608393579, 13.14518615778179544 ) ) ;
#26095=CARTESIAN_POINT ( 'NONE',  ( 120.7049497278729575, 35.69179687608393436, -9.295050272127046043 ) ) ;
#26096=CARTESIAN_POINT ( 'NONE',  ( 78.57481594606305464, 34.25312499999999716, -1.662435489736055892E-15 ) ) ;
#26099=CIRCLE ( 'NONE', #16994, 5.000000000000000888 ) ;
#26102=CARTESIAN_POINT ( 'NONE',  ( 96.46446615806316061, 80.00000000000000000, -3.535533969928681852 ) ) ;
#26104=CARTESIAN_POINT ( 'NONE',  ( 96.84719886470459471, 80.56250000136559208, -3.152801135295383084 ) ) ;
#26106=CARTESIAN_POINT ( 'NONE',  ( 13.14518615778179900, 35.54296875108394715, 5.444914386472293977 ) ) ;
#26109=CARTESIAN_POINT ( 'NONE',  ( -20.00000000000000355, 55.00000000000000000, -9.999999999999998224 ) ) ;
#26110=CYLINDRICAL_SURFACE ( 'NONE', #1626, 13.57481594606304398 ) ;
#26112=CARTESIAN_POINT ( 'NONE',  ( 189.5550856135277229, 37.52734375108393294, 13.14518615778179722 ) ) ;
#26114=ORIENTED_EDGE ( 'NONE', *, *, #10025, .T. ) ;
#26122=CARTESIAN_POINT ( 'NONE',  ( 130.0000000000000000, 39.16445312608392726, 13.14518615778179544 ) ) ;
#26123=CARTESIAN_POINT ( 'NONE',  ( -9.295050272127044266, 40.05742187608393579, 9.295050272127047819 ) ) ;
#26125=CARTESIAN_POINT ( 'NONE',  ( 65.00000000000000000, 39.36289062608393152, 13.14518615778179544 ) ) ;
#26128=CARTESIAN_POINT ( 'NONE',  ( 181.8548138422181921, 33.55859375108393294, -5.444914386472297529 ) ) ;
#26131=ORIENTED_EDGE ( 'NONE', *, *, #21153, .T. ) ;
#26134=CARTESIAN_POINT ( 'NONE',  ( 55.70494972787295751, 39.66054687608393436, -9.295050272127046043 ) ) ;
#26135=CARTESIAN_POINT ( 'NONE',  ( 95.54126587499996504, 81.50000000136560629, 1.846868145590724986 ) ) ;
#26136=CARTESIAN_POINT ( 'NONE',  ( 200.4449143864723055, 39.51171875108393294, -13.14518615778179722 ) ) ;
#26138=CARTESIAN_POINT ( 'NONE',  ( 186.2416656076466097, 50.00000000000000000, 10.38725784495168192 ) ) ;
#26140=CARTESIAN_POINT ( 'NONE',  ( 185.7049497278729575, 40.65273437608393436, -9.295050272127046043 ) ) ;
#26147=CARTESIAN_POINT ( 'NONE',  ( 124.5550856135277087, 35.84062500108394289, -13.14518615778179900 ) ) ;
#26148=CARTESIAN_POINT ( 'NONE',  ( 74.29505027212704249, 32.91367187608393152, 9.295050272127046043 ) ) ;
#26149=CARTESIAN_POINT ( 'NONE',  ( 204.2950502721270425, 37.87460937608393863, 9.295050272127046043 ) ) ;
#26150=CARTESIAN_POINT ( 'NONE',  ( 204.1801758136480203, 55.00000000000000000, 14.99999999999994671 ) ) ;
#26152=CARTESIAN_POINT ( 'NONE',  ( 126.1969456267529921, 54.09082899096177499, -15.00000000000000355 ) ) ;
#26153=DIRECTION ( 'NONE',  ( 0.000000000000000000, -1.000000000000000000, 0.000000000000000000 ) ) ;
#26154=FACE_OUTER_BOUND ( 'NONE', #6617, .T. ) ;
#26156=CARTESIAN_POINT ( 'NONE',  ( 13.14518615778179544, 36.18789062608393436, -1.609821015232357215E-15 ) ) ;
#26158=CARTESIAN_POINT ( 'NONE',  ( 104.9999999999999716, 79.62500000273119838, -1.449011120738813565E-14 ) ) ;
#26160=ADVANCED_FACE ( 'NONE', ( #26659 ), #13659, .T. ) ;
#26164=ORIENTED_EDGE ( 'NONE', *, *, #618, .T. ) ;
#26170=CARTESIAN_POINT ( 'NONE',  ( 96.84719886470459471, 80.81250000136559208, 3.152801135295355994 ) ) ;
#26171=CARTESIAN_POINT ( 'NONE',  ( 78.14518615778179367, 33.95546875108393436, 5.444914386472293977 ) ) ;
#26173=CARTESIAN_POINT ( 'NONE',  ( 9.295050272127046043, 37.08085937608393579, -9.295050272127046043 ) ) ;
#26177=CARTESIAN_POINT ( 'NONE',  ( 130.0000000000000000, 37.22968749999999716, 13.57481594606304576 ) ) ;
#26178=VERTEX_POINT ( 'NONE', #11233 ) ;
#26182=CARTESIAN_POINT ( 'NONE',  ( 130.0000000000000000, 37.97382812608393721, -13.14518615778179544 ) ) ;
#26183=CARTESIAN_POINT ( 'NONE',  ( 78.57481594606305464, 32.76484375216787015, -1.662435489736055892E-15 ) ) ;
#26186=CARTESIAN_POINT ( 'NONE',  ( -13.57481594606304576, 32.36796875216787583, 0.000000000000000000 ) ) ;
#26190=CARTESIAN_POINT ( 'NONE',  ( 185.7049497278729575, 33.50898437608393010, 9.295050272127047819 ) ) ;
#26192=CIRCLE ( 'NONE', #4348, 5.000000000000000888 ) ;
#26194=EDGE_LOOP ( 'NONE', ( #21726, #26691, #7457, #8181 ) ) ;
#26195=CARTESIAN_POINT ( 'NONE',  ( 181.4251840539369596, 40.15664062499999432, -5.622872871577872189 ) ) ;
#26199=CYLINDRICAL_SURFACE ( 'NONE', #25271, 13.57481594606304398 ) ;
#26203=EDGE_CURVE ( 'NONE', #18001, #15330, #25702, .T. ) ;
#26204=CARTESIAN_POINT ( 'NONE',  ( 195.0000000000000000, 35.64218749999999147, 13.57481594606304576 ) ) ;
#26207=CARTESIAN_POINT ( 'NONE',  ( 51.85481384221820633, 34.25312500108393010, 5.444914386472304635 ) ) ;
#26213=CARTESIAN_POINT ( 'NONE',  ( 13.57481594606304931, 35.79101562499999289, 5.622872871577869525 ) ) ;
#26214=CARTESIAN_POINT ( 'NONE',  ( 135.4449143864723055, 38.61875000108393152, 13.14518615778179189 ) ) ;
#26215=EDGE_CURVE ( 'NONE', #4003, #24599, #6549, .T. ) ;
#26216=ORIENTED_EDGE ( 'NONE', *, *, #23255, .F. ) ;
#26217=ORIENTED_EDGE ( 'NONE', *, *, #2565, .T. ) ;
#26218=CARTESIAN_POINT ( 'NONE',  ( 103.1528011352953342, 80.31250000136559208, -3.152801135295383084 ) ) ;
#26219=CARTESIAN_POINT ( 'NONE',  ( 94.99999999999995737, 83.18750000273119838, 2.071067811865466624 ) ) ;
#26222=CARTESIAN_POINT ( 'NONE',  ( 63.18349958271478073, 36.00000000000000711, -13.35830014193481929 ) ) ;
#26225=CARTESIAN_POINT ( 'NONE',  ( 59.55508561352770158, 35.04687500108393294, -13.14518615778179900 ) ) ;
#26226=VERTEX_POINT ( 'NONE', #24933 ) ;
#26232=CARTESIAN_POINT ( 'NONE',  ( 189.3771271284221314, 34.89804687716787868, 13.57481594606304753 ) ) ;
#26233=CIRCLE ( 'NONE', #13929, 13.57481594606304398 ) ;
#26235=CARTESIAN_POINT ( 'NONE',  ( -13.57481594606304576, 40.99999999999999289, 0.000000000000000000 ) ) ;
#26236=EDGE_CURVE ( 'NONE', #4294, #4960, #20214, .T. ) ;
#26237=DIRECTION ( 'NONE',  ( -0.000000000000000000, 1.000000000000000000, 0.000000000000000000 ) ) ;
#26239=CARTESIAN_POINT ( 'NONE',  ( 9.295050272127046043, 37.27929687608394005, -9.295050272127046043 ) ) ;
#26240=CARTESIAN_POINT ( 'NONE',  ( 143.1451861577818079, 34.55078125108393294, 5.444914386472293977 ) ) ;
#26241=CARTESIAN_POINT ( 'NONE',  ( 59.37712712842213136, 36.08867187500000284, -13.57481594606304753 ) ) ;
#26242=CARTESIAN_POINT ( 'NONE',  ( -8.312177448680279460E-16, 38.51953125216787299, -13.57481594606304576 ) ) ;
#26244=DIRECTION ( 'NONE',  ( 7.228014483236696740E-18, 0.000000000000000000, 1.000000000000000000 ) ) ;
#26246=ADVANCED_FACE ( 'NONE', ( #16236 ), #9298, .T. ) ;
#26249=CARTESIAN_POINT ( 'NONE',  ( -8.312177448680279460E-16, 40.80156249999999574, -13.57481594606304576 ) ) ;
#26251=CARTESIAN_POINT ( 'NONE',  ( -13.14518615778179544, 35.19570312608393436, 0.000000000000000000 ) ) ;
#26252=EDGE_CURVE ( 'NONE', #16430, #19618, #23134, .T. ) ;
#26257=AXIS2_PLACEMENT_3D ( 'NONE', #7192, #15889, #26894 ) ;
#26260=CARTESIAN_POINT ( 'NONE',  ( 208.1451861577817795, 38.61875000108393152, -5.444914386472297529 ) ) ;
#26263=LINE ( 'NONE', #6722, #13986 ) ;
#26268=CARTESIAN_POINT ( 'NONE',  ( 135.6228728715778686, 32.91367187716787157, -13.57481594606304753 ) ) ;
#26269=CARTESIAN_POINT ( 'NONE',  ( 217.9999999999999716, 52.00000000000000711, 0.000000000000000000 ) ) ;
#26272=CARTESIAN_POINT ( 'NONE',  ( 55.70494972787295751, 39.06523437608392868, -9.295050272127046043 ) ) ;
#26273=DIRECTION ( 'NONE',  ( 0.000000000000000000, -1.000000000000000000, 0.000000000000000000 ) ) ;
#26274=CARTESIAN_POINT ( 'NONE',  ( 200.4449143864723055, 33.85625000108393579, 13.14518615778179189 ) ) ;
#26283=CARTESIAN_POINT ( 'NONE',  ( 96.84719886470459471, 82.31250000136559208, -3.152801135295383084 ) ) ;
#26284=CARTESIAN_POINT ( 'NONE',  ( 185.7049497278729575, 38.07304687608393579, -9.295050272127046043 ) ) ;
#26287=FACE_OUTER_BOUND ( 'NONE', #14845, .T. ) ;
#26290=VERTEX_POINT ( 'NONE', #20453 ) ;
#26295=CARTESIAN_POINT ( 'NONE',  ( 143.1451861577818079, 37.13046875108393863, 5.444914386472293977 ) ) ;
#26296=AXIS2_PLACEMENT_3D ( 'NONE', #17983, #21987, #17845 ) ;
#26297=CARTESIAN_POINT ( 'NONE',  ( 51.85481384221820633, 33.45937500108392726, 5.444914386472304635 ) ) ;
#26298=CARTESIAN_POINT ( 'NONE',  ( 181.8548138422181921, 38.32109375108394289, -5.444914386472297529 ) ) ;
#26301=CARTESIAN_POINT ( 'NONE',  ( -9.295050272127044266, 32.71523437608393436, 9.295050272127047819 ) ) ;
#26302=CARTESIAN_POINT ( 'NONE',  ( 130.8389268692911571, 53.50081894914646341, -15.00000000000000000 ) ) ;
#26303=CARTESIAN_POINT ( 'NONE',  ( 143.5748159460630688, 39.90859375216787441, -1.662435489736055892E-15 ) ) ;
#26304=CARTESIAN_POINT ( 'NONE',  ( 2.493653234604083739E-15, 39.61093749999999147, 13.57481594606304576 ) ) ;
#26308=VERTEX_POINT ( 'NONE', #11585 ) ;
#26311=ORIENTED_EDGE ( 'NONE', *, *, #8641, .F. ) ;
#26314=CARTESIAN_POINT ( 'NONE',  ( 123.8822400544581228, 54.65941425415167032, 14.99999999999996980 ) ) ;
#26317=CARTESIAN_POINT ( 'NONE',  ( 116.4251840539369738, 38.76757812716787299, 5.622872871577880183 ) ) ;
#26318=CARTESIAN_POINT ( 'NONE',  ( 103.1528011352953342, 80.31250000136559208, -3.152801135295383084 ) ) ;
#26319=CARTESIAN_POINT ( 'NONE',  ( 65.00000000000000000, 34.99726562608393721, -13.14518615778179544 ) ) ;
#26321=CARTESIAN_POINT ( 'NONE',  ( -9.295050272127046043, 38.07304687608393579, -9.295050272127046043 ) ) ;
#26324=CARTESIAN_POINT ( 'NONE',  ( 195.0000000000000000, -7.395377635281828788, -2.255140518769849538E-14 ) ) ;
#26326=CARTESIAN_POINT ( 'NONE',  ( 116.4251840539369596, 38.66835937499999432, 5.622872871577880183 ) ) ;
#26331=CARTESIAN_POINT ( 'NONE',  ( 116.8548138422182063, 37.42812500108393436, 5.444914386472304635 ) ) ;
#26332=CARTESIAN_POINT ( 'NONE',  ( 74.59884440882045453, 34.25312500216787015, 9.598844408820456309 ) ) ;
#26333=ORIENTED_EDGE ( 'NONE', *, *, #14339, .F. ) ;
#26335=CARTESIAN_POINT ( 'NONE',  ( 104.9999999999999716, 83.50000000000000000, -1.449011120738813565E-14 ) ) ;
#26336=CARTESIAN_POINT ( 'NONE',  ( -13.57481594606304576, 34.00507812716787015, 5.622872871577880183 ) ) ;
#26337=AXIS2_PLACEMENT_3D ( 'NONE', #3326, #1063, #7053 ) ;
#26340=CARTESIAN_POINT ( 'NONE',  ( 94.99999999999995737, 85.00000000000000000, -1.387778780781445676E-14 ) ) ;
#26341=AXIS2_PLACEMENT_3D ( 'NONE', #5977, #6621, #15594 ) ;
#26342=CARTESIAN_POINT ( 'NONE',  ( 200.4449143864723055, 35.54296875108393294, -13.14518615778179900 ) ) ;
#26343=DIRECTION ( 'NONE',  ( 0.000000000000000000, -1.000000000000000000, 0.000000000000000000 ) ) ;
#26345=CARTESIAN_POINT ( 'NONE',  ( 195.0000000000000000, 39.21406249999999716, -13.57481594606304576 ) ) ;
#26347=CARTESIAN_POINT ( 'NONE',  ( 200.6228728715780107, 36.78320312499999289, -13.57481594606290898 ) ) ;
#26352=CARTESIAN_POINT ( 'NONE',  ( 208.5748159460630688, 34.25312499999999716, -1.662435489736055892E-15 ) ) ;
#26354=CARTESIAN_POINT ( 'NONE',  ( 99.99999999999995737, 81.87500000273119838, -5.000000000000018652 ) ) ;
#26356=CARTESIAN_POINT ( 'NONE',  ( 70.44491438647230552, 35.24531250108393010, 13.14518615778179189 ) ) ;
#26361=CARTESIAN_POINT ( 'NONE',  ( -9.598844408820454532, 37.13046874999999147, 9.598844408820459861 ) ) ;
#26362=CARTESIAN_POINT ( 'NONE',  ( 135.4449143864723055, 36.23750000108393721, 13.14518615778179189 ) ) ;
#26363=VERTEX_POINT ( 'NONE', #14010 ) ;
#26364=CARTESIAN_POINT ( 'NONE',  ( 103.5355339059327093, 84.37500000000000000, 3.535533905932726206 ) ) ;
#26365=CARTESIAN_POINT ( 'NONE',  ( 96.46446609406721961, 83.00000000273119838, -3.535533905932755072 ) ) ;
#26367=AXIS2_PLACEMENT_3D ( 'NONE', #742, #24387, #13540 ) ;
#26368=CARTESIAN_POINT ( 'NONE',  ( 51.82584278307725612, 36.00000000000001421, 0.03826467346021202032 ) ) ;
#26370=CARTESIAN_POINT ( 'NONE',  ( 78.14518615778179367, 33.26093750108393721, -5.444914386472297529 ) ) ;
#26372=ORIENTED_EDGE ( 'NONE', *, *, #2185, .F. ) ;
#26373=EDGE_CURVE ( 'NONE', #6096, #15330, #24964, .T. ) ;
#26374=CARTESIAN_POINT ( 'NONE',  ( 130.0000000000000000, 38.91640625216786731, 13.57481594606304576 ) ) ;
#26378=DIRECTION ( 'NONE',  ( -1.000000000000000000, -0.000000000000000000, -0.000000000000000000 ) ) ;
#26380=CARTESIAN_POINT ( 'NONE',  ( 208.5748159460630120, 33.60820312716787583, -5.622872871577873077 ) ) ;
#26384=CARTESIAN_POINT ( 'NONE',  ( 116.8548138422182205, 37.52734375108393294, -5.444914386472297529 ) ) ;
#26385=CARTESIAN_POINT ( 'NONE',  ( -13.14518615778179189, 35.24531250108393721, 5.444914386472304635 ) ) ;
#26387=CARTESIAN_POINT ( 'NONE',  ( 139.2950502721270425, 36.08867187608392868, 9.295050272127046043 ) ) ;
#26388=CARTESIAN_POINT ( 'NONE',  ( 78.57481594606304043, 34.20351562499999432, 5.622872871577869525 ) ) ;
#26390=VECTOR ( 'NONE', #22803, 1000.000000000000000 ) ;
#26391=EDGE_CURVE ( 'NONE', #10301, #9895, #15407, .T. ) ;
#26393=CARTESIAN_POINT ( 'NONE',  ( 130.0000000000000000, 36.03906250000000000, -13.57481594606304576 ) ) ;
#26398=CARTESIAN_POINT ( 'NONE',  ( -13.14518615778179900, 37.52734375108393294, -5.444914386472297529 ) ) ;
#26404=CARTESIAN_POINT ( 'NONE',  ( 200.4449143864723055, 38.42031250108393436, 13.14518615778179189 ) ) ;
#26409=CIRCLE ( 'NONE', #12282, 11.57481594606304398 ) ;
#26410=VERTEX_POINT ( 'NONE', #19697 ) ;
#26415=CARTESIAN_POINT ( 'NONE',  ( 120.7049497278729575, 39.85898437608393152, 9.295050272127047819 ) ) ;
#26416=CARTESIAN_POINT ( 'NONE',  ( 5.444914386472297529, 40.50390625108394005, -13.14518615778179722 ) ) ;
#26418=CARTESIAN_POINT ( 'NONE',  ( 59.55508561352770158, 39.01562500108394005, -13.14518615778179900 ) ) ;
#26419=CARTESIAN_POINT ( 'NONE',  ( 61.95539054307062088, 53.89089363584123760, -15.00000000000000000 ) ) ;
#26420=CARTESIAN_POINT ( 'NONE',  ( 204.5988444088204687, 40.50390624999999289, 9.598844408820456309 ) ) ;
#26421=ADVANCED_FACE ( 'NONE', ( #19417 ), #12840, .F. ) ;
#26427=CARTESIAN_POINT ( 'NONE',  ( 51.85481384221820633, 40.50390625108394005, -5.444914386472297529 ) ) ;
#26428=CARTESIAN_POINT ( 'NONE',  ( 103.1528011352953342, 82.06250000136559208, -3.152801135295383084 ) ) ;
#26429=CARTESIAN_POINT ( 'NONE',  ( 208.1451861577818079, 40.15664062608393436, -1.609821015232357215E-15 ) ) ;
#26433=CARTESIAN_POINT ( 'NONE',  ( 185.7049497278729575, 38.46992187608393721, 9.295050272127047819 ) ) ;
#26435=EDGE_LOOP ( 'NONE', ( #21669, #8583, #22378, #14082 ) ) ;
#26439=CARTESIAN_POINT ( 'NONE',  ( 143.1451861577818079, 32.41757812608393863, -1.609821015232357215E-15 ) ) ;
#26440=CARTESIAN_POINT ( 'NONE',  ( 55.70494972787295751, 34.30273437608393294, 9.295050272127047819 ) ) ;
#26441=CARTESIAN_POINT ( 'NONE',  ( 200.4449143864723055, 38.61875000108393152, 13.14518615778179189 ) ) ;
#26444=CARTESIAN_POINT ( 'NONE',  ( 2.414731522848535132E-15, 32.02070312608393010, 13.14518615778179544 ) ) ;
#26448=CARTESIAN_POINT ( 'NONE',  ( 65.00000000000000000, 40.80156249999999574, -13.57481594606304576 ) ) ;
#26453=VECTOR ( 'NONE', #27686, 1000.000000000000000 ) ;
#26455=SHAPE_REPRESENTATION_RELATIONSHIP ( 'NONE' , 'NONE' ,  #14045, #2892 ) ;
#26456=EDGE_LOOP ( 'NONE', ( #23335, #6910, #20724, #26311 ) ) ;
#26458=ORIENTED_EDGE ( 'NONE', *, *, #7139, .F. ) ;
#26461=CARTESIAN_POINT ( 'NONE',  ( 69.15728635496172672, 36.00000000000000000, -12.92256159328856135 ) ) ;
#26463=FACE_BOUND ( 'NONE', #25570, .T. ) ;
#26464=CARTESIAN_POINT ( 'NONE',  ( 99.99999999999995737, 82.93750000136560629, 4.458734124999988779 ) ) ;
#26465=CARTESIAN_POINT ( 'NONE',  ( 78.14518615778179367, 36.33671875108394289, 5.444914386472293977 ) ) ;
#26467=CARTESIAN_POINT ( 'NONE',  ( -5.444914386472299306, 39.11484375108393863, 13.14518615778179722 ) ) ;
#26471=CARTESIAN_POINT ( 'NONE',  ( 143.5748159460630404, 37.47773437500001137, -5.622872871577873077 ) ) ;
#26472=ORIENTED_EDGE ( 'NONE', *, *, #8793, .F. ) ;
#26473=ORIENTED_EDGE ( 'NONE', *, *, #27991, .T. ) ;
#26478=CARTESIAN_POINT ( 'NONE',  ( 135.4449143864723055, 33.16171875108393152, -13.14518615778179900 ) ) ;
#26479=CARTESIAN_POINT ( 'NONE',  ( 70.62287287157786864, 32.91367187716787157, -13.57481594606304753 ) ) ;
#26481=DIRECTION ( 'NONE',  ( -0.000000000000000000, -1.000000000000000000, -0.000000000000000000 ) ) ;
#26482=CARTESIAN_POINT ( 'NONE',  ( 5.622872871577878406, 33.40976562716787157, 13.57481594606304576 ) ) ;
#26483=CARTESIAN_POINT ( 'NONE',  ( 59.37712712842203189, 37.97382812499999716, 13.57481594606295161 ) ) ;
#26486=CARTESIAN_POINT ( 'NONE',  ( 208.1451861577817795, 33.75703125108393010, 5.444914386472293977 ) ) ;
#26487=FACE_OUTER_BOUND ( 'NONE', #1222, .T. ) ;
#26488=CARTESIAN_POINT ( 'NONE',  ( 131.1371678245417627, 36.00000000000000000, 13.09590655363595602 ) ) ;
#26489=CARTESIAN_POINT ( 'NONE',  ( 208.5748159460630688, 39.01562500000000000, -1.662435489736055892E-15 ) ) ;
#26491=CARTESIAN_POINT ( 'NONE',  ( 138.3922152916384221, 55.00000000000001421, 14.99999999999997158 ) ) ;
#26493=LINE ( 'NONE', #20077, #16170 ) ;
#26496=CARTESIAN_POINT ( 'NONE',  ( 185.4011555911795313, 35.34453124999998863, -9.598844408820458085 ) ) ;
#26497=CARTESIAN_POINT ( 'NONE',  ( -8.312177448680279460E-16, 36.13828125216787157, -13.57481594606304576 ) ) ;
#26499=CARTESIAN_POINT ( 'NONE',  ( 65.00000000000000000, 34.79882812608393294, -13.14518615778179544 ) ) ;
#26500=EDGE_CURVE ( 'NONE', #21442, #21964, #11280, .T. ) ;
#26505=CARTESIAN_POINT ( 'NONE',  ( -5.622872871577873077, 36.88242187499999858, -13.57481594606304753 ) ) ;
#26506=CARTESIAN_POINT ( 'NONE',  ( 116.8548138422182063, 38.42031250108393436, 5.444914386472304635 ) ) ;
#26508=CARTESIAN_POINT ( 'NONE',  ( 99.99999999999995737, 81.75000000000000000, -5.000000000000018652 ) ) ;
#26509=DIRECTION ( 'NONE',  ( 0.000000000000000000, 0.000000000000000000, 1.000000000000000000 ) ) ;
#26510=CARTESIAN_POINT ( 'NONE',  ( 99.99999999999995737, 80.87500000273119838, -5.000000000000018652 ) ) ;
#26514=CARTESIAN_POINT ( 'NONE',  ( 51.85481384221819923, 31.97109375108393436, -5.444914386472297529 ) ) ;
#26515=ORIENTED_EDGE ( 'NONE', *, *, #14922, .T. ) ;
#26516=FACE_OUTER_BOUND ( 'NONE', #2566, .T. ) ;
#26519=ORIENTED_EDGE ( 'NONE', *, *, #24830, .T. ) ;
#26521=CARTESIAN_POINT ( 'NONE',  ( 195.0000000000000000, 33.75703125216787726, -13.57481594606304576 ) ) ;
#26525=CARTESIAN_POINT ( 'NONE',  ( 135.4449143864723339, 36.23750000108393721, 13.14518615778179189 ) ) ;
#26526=ORIENTED_EDGE ( 'NONE', *, *, #11191, .F. ) ;
#26527=CARTESIAN_POINT ( 'NONE',  ( 2.414731522848535132E-15, 33.80664062608393294, 13.14518615778179544 ) ) ;
#26529=CARTESIAN_POINT ( 'NONE',  ( 51.42518405393695957, 35.44374999999999432, 0.000000000000000000 ) ) ;
#26532=CARTESIAN_POINT ( 'NONE',  ( 207.5314254911195349, 35.99999999999997868, -5.200562670744174554 ) ) ;
#26535=CARTESIAN_POINT ( 'NONE',  ( 195.0000000000000000, -7.395377635281828788, -2.255140518769849538E-14 ) ) ;
#26536=DIRECTION ( 'NONE',  ( 0.000000000000000000, 0.000000000000000000, 1.000000000000000000 ) ) ;
#26538=CARTESIAN_POINT ( 'NONE',  ( -9.295050272127044266, 36.08867187608393579, 9.295050272127047819 ) ) ;
#26539=CIRCLE ( 'NONE', #5593, 11.57481594606304398 ) ;
#26541=ORIENTED_EDGE ( 'NONE', *, *, #18597, .T. ) ;
#26543=( BOUNDED_SURFACE ( )  B_SPLINE_SURFACE ( 1, 2, ( 
 ( #27695, #4309, #21420, #1479, #28111, #8157, #6028, #10135, #4170, #23553, #4030, #21274, #6163, #6439, #10700, #21557, #12695, #18847, #25411, #8575, #14563, #19406, #19273, #5893, #27972, #23278, #18985, #3751, #23693, #14974, #19129, #27836, #16849, #12413, #21133, #1618, #3886, #17265, #15108, #1757, #10276, #23829, #25548, #14692, #23412, #1898, #12547, #10564, #8430, #8290, #17119, #16982, #25823, #6297, #19831, #19551, #11261, #21699, #23971, #316, #4879, #8857, #5021, #2174, #9003, #26398, #19688, #21843, #13543, #601, #4587, #11404, #17695, #22121, #15253, #8714, #9280, #6853, #22265, #2319, #20123, #175, #24110, #6571, #2739, #4450, #17977, #15542, #24250, #15689, #2600, #26686, #10836, #459, #26538, #17406, #7133, #6995, #32, #13393, #21979, #13104, #10976, #4733, #19981, #26106, #17548, #15830, #2455, #24536, #13247, #9141, #26251, #6711, #15398, #11117, #17834, #24391, #7419, #25237, #22403, #5160, #22692, #20260, #5303, #16547, #746, #22547, #3439, #13686, #15969, #18551, #7852, #27116, #12106, #11832, #9565, #895, #13967, #20696, #11543, #9419, #27255, #2872, #20556, #1179, #18409, #3162, #3016, #1037, #14254, #7714, #11685, #14113, #22837, #9708, #7566, #16406, #16260, #25103, #24960, #20409, #3303, #5446, #18690, #11973, #18268, #1309, #26974, #5589, #18118, #24683, #20832, #9980, #9845, #27393, #16114, #26833, #7278, #22975, #13823, #24819, #14533 ),
 ( #14394, #12661, #10530, #1453, #4135, #19236, #12242, #25647, #5996, #18822, #16684, #19095, #27803, #20970, #7985, #12798, #14661, #25788, #16821, #6131, #25383, #5727, #27663, #27529, #10108, #25517, #1725, #21519, #23382, #23247, #3854, #8259, #5862, #27937, #8541, #12515, #3724, #17227, #14796, #23110, #1998, #12386, #10246, #3584, #8396, #16946, #23520, #21244, #10387, #10665, #6265, #17085, #3998, #21104, #1592, #19373, #18955, #21388, #8125, #1865, #14938, #23660, #28077, #2667, #24075, #9107, #13069, #9249, #6407, #4553, #2425, #23935, #26069, #17801, #4844, #8822, #15655, #13213, #26361, #19516, #12930, #13507, #21947, #26505, #6538, #24355, #4415, #136, #10803, #6961, #8683, #22228, #11085, #19795, #19942, #6819, #2707, #15076, #4698, #2563, #21662, #11367, #11226, #4271, #17653, #26213, #17373, #15216, #279, #8965, #2139, #21806, #20089, #6674, #567, #17512, #15509, #2284, #25932, #19654, #10942, #15361, #24219, #13359, #23794, #22086, #421, #16076, #20518, #18081, #3268, #20796, #24784, #15932, #1276, #9669, #17941, #16367, #24649, #22510, #26651, #20658, #3129, #1000, #9531, #13931, #14220, #18516, #1143, #11795, #7099, #15797, #25068, #2840, #27221, #7529, #4987, #16225, #11508, #7240, #13652, #11936, #9810, #7383, #5265, #5122, #24500, #709, #9384, #20374, #7675, #5555, #18229, #22367, #3401, #22938, #12071, #2976, #18372, #26794, #22658, #27077, #13789 ) ),
 .UNSPECIFIED., .F., .F., .F. ) 
 B_SPLINE_SURFACE_WITH_KNOTS ( ( 2, 2 ),
 ( 3, 2, 2, 2, 2, 2, 2, 2, 2, 2, 2, 2, 2, 2, 2, 2, 2, 2, 2, 2, 2, 2, 2, 2, 2, 2, 2, 2, 2, 2, 2, 2, 2, 2, 2, 2, 2, 2, 2, 2, 2, 2, 2, 2, 2, 2, 2, 2, 2, 2, 2, 2, 2, 2, 2, 2, 2, 2, 2, 2, 2, 2, 2, 2, 2, 2, 2, 2, 2, 2, 2, 2, 2, 2, 2, 2, 2, 2, 2, 2, 2, 2, 2, 2, 2, 2, 2, 2, 2, 2, 2, 3 ),
 ( 0.000000000000000000, 1.000000000000000000 ),
 ( 0.000000000000000000, 0.01041666666666666609, 0.02083333333333333218, 0.03125000000000000000, 0.04166666666666666435, 0.05208333333333333565, 0.06250000000000000000, 0.07291666666666667129, 0.08333333333333332871, 0.09375000000000000000, 0.1041666666666666713, 0.1145833333333333287, 0.1250000000000000000, 0.1354166666666666574, 0.1458333333333333426, 0.1562500000000000000, 0.1666666666666666574, 0.1770833333333333426, 0.1875000000000000000, 0.1979166666666666574, 0.2083333333333333426, 0.2187500000000000000, 0.2291666666666666574, 0.2395833333333333426, 0.2500000000000000000, 0.2604166666666666852, 0.2708333333333333148, 0.2812500000000000000, 0.2916666666666666852, 0.3020833333333333148, 0.3125000000000000000, 0.3229166666666666852, 0.3333333333333333148, 0.3437500000000000000, 0.3541666666666666852, 0.3645833333333333148, 0.3750000000000000000, 0.3854166666666666852, 0.3958333333333333148, 0.4062500000000000000, 0.4166666666666666852, 0.4270833333333333148, 0.4375000000000000000, 0.4479166666666666852, 0.4583333333333333148, 0.4687500000000000000, 0.4791666666666666852, 0.4895833333333333148, 0.5000000000000000000, 0.5104166666666666297, 0.5208333333333333703, 0.5312500000000000000, 0.5416666666666666297, 0.5520833333333333703, 0.5625000000000000000, 0.5729166666666666297, 0.5833333333333333703, 0.5937500000000000000, 0.6041666666666666297, 0.6145833333333333703, 0.6250000000000000000, 0.6354166666666666297, 0.6458333333333333703, 0.6562500000000000000, 0.6666666666666666297, 0.6770833333333333703, 0.6875000000000000000, 0.6979166666666666297, 0.7083333333333333703, 0.7187500000000000000, 0.7291666666666666297, 0.7395833333333333703, 0.7500000000000000000, 0.7604166666666666297, 0.7708333333333333703, 0.7812500000000000000, 0.7916666666666666297, 0.8020833333333333703, 0.8125000000000000000, 0.8229166666666666297, 0.8333333333333333703, 0.8437500000000000000, 0.8541666666666666297, 0.8645833333333333703, 0.8750000000000000000, 0.8854166666666666297, 0.8958333333333333703, 0.9062500000000000000, 0.9166666666666666297, 0.9270833333333333703, 0.9375000000000000000, 0.9448586968893691873 ),
 .UNSPECIFIED. ) 
 GEOMETRIC_REPRESENTATION_ITEM ( )  RATIONAL_B_SPLINE_SURFACE ( (
 ( 1.000000000000000000, 0.9238795325112867385, 1.000000000000000000, 0.9238795325112867385, 1.000000000000000000, 0.9238795325112867385, 1.000000000000000000, 0.9238795325112867385, 1.000000000000000000, 0.9238795325112867385, 1.000000000000000000, 0.9238795325112867385, 1.000000000000000000, 0.9238795325112867385, 1.000000000000000000, 0.9238795325112867385, 1.000000000000000000, 0.9238795325112867385, 1.000000000000000000, 0.9238795325112867385, 1.000000000000000000, 0.9238795325112867385, 1.000000000000000000, 0.9238795325112867385, 1.000000000000000000, 0.9238795325112867385, 1.000000000000000000, 0.9238795325112867385, 1.000000000000000000, 0.9238795325112867385, 1.000000000000000000, 0.9238795325112867385, 1.000000000000000000, 0.9238795325112867385, 1.000000000000000000, 0.9238795325112867385, 1.000000000000000000, 0.9238795325112867385, 1.000000000000000000, 0.9238795325112867385, 1.000000000000000000, 0.9238795325112867385, 1.000000000000000000, 0.9238795325112867385, 1.000000000000000000, 0.9238795325112867385, 1.000000000000000000, 0.9238795325112867385, 1.000000000000000000, 0.9238795325112867385, 1.000000000000000000, 0.9238795325112867385, 1.000000000000000000, 0.9238795325112867385, 1.000000000000000000, 0.9238795325112867385, 1.000000000000000000, 0.9238795325112867385, 1.000000000000000000, 0.9238795325112867385, 1.000000000000000000, 0.9238795325112867385, 1.000000000000000000, 0.9238795325112867385, 1.000000000000000000, 0.9238795325112867385, 1.000000000000000000, 0.9238795325112867385, 1.000000000000000000, 0.9238795325112867385, 1.000000000000000000, 0.9238795325112867385, 1.000000000000000000, 0.9238795325112867385, 1.000000000000000000, 0.9238795325112867385, 1.000000000000000000, 0.9238795325112867385, 1.000000000000000000, 0.9238795325112867385, 1.000000000000000000, 0.9238795325112867385, 1.000000000000000000, 0.9238795325112867385, 1.000000000000000000, 0.9238795325112867385, 1.000000000000000000, 0.9238795325112867385, 1.000000000000000000, 0.9238795325112867385, 1.000000000000000000, 0.9238795325112867385, 1.000000000000000000, 0.9238795325112867385, 1.000000000000000000, 0.9238795325112867385, 1.000000000000000000, 0.9238795325112867385, 1.000000000000000000, 0.9238795325112867385, 1.000000000000000000, 0.9238795325112867385, 1.000000000000000000, 0.9238795325112867385, 1.000000000000000000, 0.9238795325112867385, 1.000000000000000000, 0.9238795325112867385, 1.000000000000000000, 0.9238795325112867385, 1.000000000000000000, 0.9238795325112867385, 1.000000000000000000, 0.9238795325112867385, 1.000000000000000000, 0.9238795325112867385, 1.000000000000000000, 0.9238795325112867385, 1.000000000000000000, 0.9238795325112867385, 1.000000000000000000, 0.9238795325112867385, 1.000000000000000000, 0.9238795325112867385, 1.000000000000000000, 0.9238795325112867385, 1.000000000000000000, 0.9238795325112867385, 1.000000000000000000, 0.9238795325112867385, 1.000000000000000000, 0.9238795325112867385, 1.000000000000000000, 0.9238795325112867385, 1.000000000000000000, 0.9238795325112867385, 1.000000000000000000, 0.9238795325112867385, 1.000000000000000000, 0.9238795325112867385, 1.000000000000000000, 0.9238795325112867385, 1.000000000000000000, 0.9238795325112867385, 1.000000000000000000, 0.9238795325112867385, 1.000000000000000000, 0.9238795325112867385, 1.000000000000000000, 0.9238795325112867385, 1.000000000000000000, 0.9238795325112867385, 1.000000000000000000, 0.9238795325112867385, 1.000000000000000000, 0.9238795325112867385, 1.000000000000000000, 0.9238795325112867385, 1.000000000000000000, 0.9238795325112867385, 1.000000000000000000, 0.9238795325112867385, 1.000000000000000000, 0.9238795325112867385, 1.000000000000000000, 0.9238795325112867385, 1.000000000000000000, 0.9238795325112867385, 1.000000000000000000, 0.9238795325112867385, 1.000000000000000000, 0.9238795325112867385, 1.000000000000000000, 0.9238795325112867385, 1.000000000000000000, 0.9238795325112867385, 1.000000000000000000, 0.9238795325112867385, 1.000000000000000000, 0.9238795325112867385, 1.000000000000000000, 0.9462258450566536361, 0.9684275698016389100),
 ( 1.000000000000000000, 0.9238795325112867385, 1.000000000000000000, 0.9238795325112867385, 1.000000000000000000, 0.9238795325112867385, 1.000000000000000000, 0.9238795325112867385, 1.000000000000000000, 0.9238795325112867385, 1.000000000000000000, 0.9238795325112867385, 1.000000000000000000, 0.9238795325112867385, 1.000000000000000000, 0.9238795325112867385, 1.000000000000000000, 0.9238795325112867385, 1.000000000000000000, 0.9238795325112867385, 1.000000000000000000, 0.9238795325112867385, 1.000000000000000000, 0.9238795325112867385, 1.000000000000000000, 0.9238795325112867385, 1.000000000000000000, 0.9238795325112867385, 1.000000000000000000, 0.9238795325112867385, 1.000000000000000000, 0.9238795325112867385, 1.000000000000000000, 0.9238795325112867385, 1.000000000000000000, 0.9238795325112867385, 1.000000000000000000, 0.9238795325112867385, 1.000000000000000000, 0.9238795325112867385, 1.000000000000000000, 0.9238795325112867385, 1.000000000000000000, 0.9238795325112867385, 1.000000000000000000, 0.9238795325112867385, 1.000000000000000000, 0.9238795325112867385, 1.000000000000000000, 0.9238795325112867385, 1.000000000000000000, 0.9238795325112867385, 1.000000000000000000, 0.9238795325112867385, 1.000000000000000000, 0.9238795325112867385, 1.000000000000000000, 0.9238795325112867385, 1.000000000000000000, 0.9238795325112867385, 1.000000000000000000, 0.9238795325112867385, 1.000000000000000000, 0.9238795325112867385, 1.000000000000000000, 0.9238795325112867385, 1.000000000000000000, 0.9238795325112867385, 1.000000000000000000, 0.9238795325112867385, 1.000000000000000000, 0.9238795325112867385, 1.000000000000000000, 0.9238795325112867385, 1.000000000000000000, 0.9238795325112867385, 1.000000000000000000, 0.9238795325112867385, 1.000000000000000000, 0.9238795325112867385, 1.000000000000000000, 0.9238795325112867385, 1.000000000000000000, 0.9238795325112867385, 1.000000000000000000, 0.9238795325112867385, 1.000000000000000000, 0.9238795325112867385, 1.000000000000000000, 0.9238795325112867385, 1.000000000000000000, 0.9238795325112867385, 1.000000000000000000, 0.9238795325112867385, 1.000000000000000000, 0.9238795325112867385, 1.000000000000000000, 0.9238795325112867385, 1.000000000000000000, 0.9238795325112867385, 1.000000000000000000, 0.9238795325112867385, 1.000000000000000000, 0.9238795325112867385, 1.000000000000000000, 0.9238795325112867385, 1.000000000000000000, 0.9238795325112867385, 1.000000000000000000, 0.9238795325112867385, 1.000000000000000000, 0.9238795325112867385, 1.000000000000000000, 0.9238795325112867385, 1.000000000000000000, 0.9238795325112867385, 1.000000000000000000, 0.9238795325112867385, 1.000000000000000000, 0.9238795325112867385, 1.000000000000000000, 0.9238795325112867385, 1.000000000000000000, 0.9238795325112867385, 1.000000000000000000, 0.9238795325112867385, 1.000000000000000000, 0.9238795325112867385, 1.000000000000000000, 0.9238795325112867385, 1.000000000000000000, 0.9238795325112867385, 1.000000000000000000, 0.9238795325112867385, 1.000000000000000000, 0.9238795325112867385, 1.000000000000000000, 0.9238795325112867385, 1.000000000000000000, 0.9238795325112867385, 1.000000000000000000, 0.9238795325112867385, 1.000000000000000000, 0.9238795325112867385, 1.000000000000000000, 0.9238795325112867385, 1.000000000000000000, 0.9238795325112867385, 1.000000000000000000, 0.9238795325112867385, 1.000000000000000000, 0.9238795325112867385, 1.000000000000000000, 0.9238795325112867385, 1.000000000000000000, 0.9238795325112867385, 1.000000000000000000, 0.9238795325112867385, 1.000000000000000000, 0.9238795325112867385, 1.000000000000000000, 0.9238795325112867385, 1.000000000000000000, 0.9238795325112867385, 1.000000000000000000, 0.9238795325112867385, 1.000000000000000000, 0.9238795325112867385, 1.000000000000000000, 0.9238795325112867385, 1.000000000000000000, 0.9238795325112867385, 1.000000000000000000, 0.9238795325112867385, 1.000000000000000000, 0.9238795325112867385, 1.000000000000000000, 0.9238795325112867385, 1.000000000000000000, 0.9238795325112867385, 1.000000000000000000, 0.9462258450566536361, 0.9684275698016389100) ) ) 
 REPRESENTATION_ITEM ( '' )  SURFACE ( )  );
#26546=CARTESIAN_POINT ( 'NONE',  ( 208.1451861577817795, 35.44375000108393436, -5.444914386472297529 ) ) ;
#26555=CARTESIAN_POINT ( 'NONE',  ( 116.8548138422182205, 39.75976562608393294, 0.000000000000000000 ) ) ;
#26556=CARTESIAN_POINT ( 'NONE',  ( 5.444914386472302859, 39.41250000108393436, 13.14518615778179189 ) ) ;
#26558=ORIENTED_EDGE ( 'NONE', *, *, #26215, .F. ) ;
#26560=CARTESIAN_POINT ( 'NONE',  ( 78.14518615778179367, 38.81718750108393579, -5.444914386472297529 ) ) ;
#26561=CARTESIAN_POINT ( 'NONE',  ( 65.83892686928035687, 53.50081894914647052, -15.00000000000000000 ) ) ;
#26563=CARTESIAN_POINT ( 'NONE',  ( 200.6228728715778686, 40.45429687500001137, 13.57481594606304576 ) ) ;
#26564=DIRECTION ( 'NONE',  ( -0.000000000000000000, -1.000000000000000000, -0.000000000000000000 ) ) ;
#26569=CARTESIAN_POINT ( 'NONE',  ( 51.85481384221821344, 37.42812500108393436, 5.444914386472304635 ) ) ;
#26571=CARTESIAN_POINT ( 'NONE',  ( -13.09590655363597733, 36.00000000000000000, 1.137167824541468031 ) ) ;
#26576=CARTESIAN_POINT ( 'NONE',  ( 181.8548138422182205, 38.37070312608393152, 0.000000000000000000 ) ) ;
#26579=AXIS2_PLACEMENT_3D ( 'NONE', #25182, #27340, #3379 ) ;
#26582=ORIENTED_EDGE ( 'NONE', *, *, #6192, .T. ) ;
#26583=CARTESIAN_POINT ( 'NONE',  ( 124.5550856135277087, 32.66562500108393863, -13.14518615778179900 ) ) ;
#26584=CARTESIAN_POINT ( 'NONE',  ( 189.3771271284220745, 36.98164062716787015, -13.57481594606304753 ) ) ;
#26585=ADVANCED_FACE ( 'NONE', ( #3141 ), #18040, .T. ) ;
#26586=CARTESIAN_POINT ( 'NONE',  ( 195.0000000000000000, 34.20351562608394147, -13.14518615778179544 ) ) ;
#26587=ORIENTED_EDGE ( 'NONE', *, *, #13803, .T. ) ;
#26589=CARTESIAN_POINT ( 'NONE',  ( -8.049105076161786076E-16, 31.62382812608393579, -13.14518615778179544 ) ) ;
#26592=CARTESIAN_POINT ( 'NONE',  ( 74.59884440882045453, 40.50390624999999289, 9.598844408820456309 ) ) ;
#26594=( BOUNDED_CURVE ( )  B_SPLINE_CURVE ( 2, ( #12377, #14654, #7976, #5719, #23102, #25780, #8389, #17075, #23239 ),
 .UNSPECIFIED., .F., .F. ) 
 B_SPLINE_CURVE_WITH_KNOTS ( ( 3, 2, 2, 2, 3 ),
 ( 0.1458333333333336757, 0.1562500000000002776, 0.1666666666666669072, 0.1770833333333335369, 0.1875000000000001388 ),
 .UNSPECIFIED. ) 
 CURVE ( )  GEOMETRIC_REPRESENTATION_ITEM ( )  RATIONAL_B_SPLINE_CURVE ( ( 0.9999999999999975575, 0.9238795325112891810, 1.000000000000000000, 0.9238795325112867385, 1.000000000000000000, 0.9238795325112867385, 1.000000000000000000, 0.9238795325112857393, 1.000000000000001110 ) ) 
 REPRESENTATION_ITEM ( '' )  );
#26597=CARTESIAN_POINT ( 'NONE',  ( 68.80305437324149409, 54.09082899096177499, 14.99999999999997868 ) ) ;
#26604=CARTESIAN_POINT ( 'NONE',  ( 137.6219635341832088, 54.91641323977227529, 14.99999999999996092 ) ) ;
#26609=CARTESIAN_POINT ( 'NONE',  ( 59.55508561352770158, 35.84062500108394289, -13.14518615778179900 ) ) ;
#26611=CARTESIAN_POINT ( 'NONE',  ( -9.295050272127046043, 37.27929687608393294, -9.295050272127046043 ) ) ;
#26614=CARTESIAN_POINT ( 'NONE',  ( 8.201446187642728702, 50.69246985422709173, 14.99999999999930012 ) ) ;
#26616=CARTESIAN_POINT ( 'NONE',  ( 130.0000000000000000, 36.43593749999999432, 13.57481594606304576 ) ) ;
#26617=ORIENTED_EDGE ( 'NONE', *, *, #8960, .F. ) ;
#26618=ADVANCED_FACE ( 'NONE', ( #18168 ), #9466, .T. ) ;
#26620=CARTESIAN_POINT ( 'NONE',  ( 130.0000000000000000, 37.32890625216786873, 13.57481594606304576 ) ) ;
#26624=CARTESIAN_POINT ( 'NONE',  ( 143.1451861577818079, 32.96328125108393436, 5.444914386472293977 ) ) ;
#26625=CARTESIAN_POINT ( 'NONE',  ( 78.57481594606304043, 33.60820312716787583, -5.622872871577873077 ) ) ;
#26627=CARTESIAN_POINT ( 'NONE',  ( -5.622872871577873077, 31.72304687716787441, 13.57481594606304753 ) ) ;
#26632=CARTESIAN_POINT ( 'NONE',  ( 195.0000000000000000, 32.81445312608393294, 13.14518615778179544 ) ) ;
#26636=CARTESIAN_POINT ( 'NONE',  ( 99.99999999999995737, 83.25000000000000000, 4.999999999999990230 ) ) ;
#26639=CARTESIAN_POINT ( 'NONE',  ( 143.5748159460630688, 38.27148437500000711, -5.622872871577873966 ) ) ;
#26642=CARTESIAN_POINT ( 'NONE',  ( 195.0000000000000000, 33.26093749999999716, 13.57481594606304576 ) ) ;
#26647=CARTESIAN_POINT ( 'NONE',  ( 51.85481384221819923, 36.53515625108392584, -5.444914386472297529 ) ) ;
#26651=CARTESIAN_POINT ( 'NONE',  ( 2.493653234604083739E-15, 34.05468749999999289, 13.57481594606304576 ) ) ;
#26652=CARTESIAN_POINT ( 'NONE',  ( 124.5550856135277087, 39.01562500108394005, -13.14518615778179900 ) ) ;
#26653=ORIENTED_EDGE ( 'NONE', *, *, #5500, .F. ) ;
#26654=CARTESIAN_POINT ( 'NONE',  ( 96.46446609406721961, 81.12500000000000000, 3.535533905932727539 ) ) ;
#26655=AXIS2_PLACEMENT_3D ( 'NONE', #28032, #10199, #8498 ) ;
#26657=CARTESIAN_POINT ( 'NONE',  ( 96.46446609406721961, 82.25000000273119838, 3.535533905932727539 ) ) ;
#26659=FACE_OUTER_BOUND ( 'NONE', #9058, .T. ) ;
#26661=CARTESIAN_POINT ( 'NONE',  ( 55.40115559117954547, 39.51171874999999289, 9.598844408820459861 ) ) ;
#26662=CIRCLE ( 'NONE', #720, 13.57481594606304398 ) ;
#26668=CARTESIAN_POINT ( 'NONE',  ( 189.3771271284221314, 33.01289062716787726, -13.57481594606304753 ) ) ;
#26671=CARTESIAN_POINT ( 'NONE',  ( 217.9999999999999716, 78.00000000000000000, -13.00000000000000000 ) ) ;
#26672=DIRECTION ( 'NONE',  ( 0.000000000000000000, -1.000000000000000000, -0.000000000000000000 ) ) ;
#26673=CARTESIAN_POINT ( 'NONE',  ( 5.444914386472302859, 35.44375000108393436, 13.14518615778179189 ) ) ;
#26675=CARTESIAN_POINT ( 'NONE',  ( 68.87838529739120474, 32.03609435653363136, -13.57481594606304576 ) ) ;
#26677=CARTESIAN_POINT ( 'NONE',  ( 119.2131532318157952, 36.00000000000000000, 7.561388982944516002 ) ) ;
#26684=CARTESIAN_POINT ( 'NONE',  ( 104.9999999999999716, 83.62500000273119838, -1.449011120738813565E-14 ) ) ;
#26686=CARTESIAN_POINT ( 'NONE',  ( 5.444914386472302859, 36.23750000108393721, 13.14518615778179189 ) ) ;
#26688=CARTESIAN_POINT ( 'NONE',  ( 2.493653234604083739E-15, 38.02343749999999289, 13.57481594606304576 ) ) ;
#26690=CARTESIAN_POINT ( 'NONE',  ( 195.0000000000000000, 34.40195312608393152, 13.14518615778179544 ) ) ;
#26691=ORIENTED_EDGE ( 'NONE', *, *, #5336, .T. ) ;
#26692=CARTESIAN_POINT ( 'NONE',  ( 203.2113140151944890, 50.68678854790359622, -14.99999999999862332 ) ) ;
#26695=VERTEX_POINT ( 'NONE', #25281 ) ;
#26698=VECTOR ( 'NONE', #14055, 1000.000000000000000 ) ;
#26699=CARTESIAN_POINT ( 'NONE',  ( 99.99999999999995737, 79.37500000273119838, 4.999999999999990230 ) ) ;
#26700=CARTESIAN_POINT ( 'NONE',  ( 130.0000000000000000, 36.78320312608393294, 13.14518615778179544 ) ) ;
#26701=CARTESIAN_POINT ( 'NONE',  ( 9.295050272127046043, 40.45429687608393721, -9.295050272127046043 ) ) ;
#26702=CARTESIAN_POINT ( 'NONE',  ( -9.295050272127044266, 36.68398437608392726, 9.295050272127047819 ) ) ;
#26704=CARTESIAN_POINT ( 'NONE',  ( 70.44491438647230552, 36.53515625108393294, -13.14518615778179900 ) ) ;
#26705=CARTESIAN_POINT ( 'NONE',  ( 63.10781664291035753, 53.66387243068089674, -15.00000000000000000 ) ) ;
#26707=CARTESIAN_POINT ( 'NONE',  ( 189.5550856135277229, 32.96328125108393436, 13.14518615778179722 ) ) ;
#26708=CARTESIAN_POINT ( 'NONE',  ( 65.00000000000000000, 38.42031249999999432, -13.57481594606304576 ) ) ;
#26713=CIRCLE ( 'NONE', #23976, 5.000000000000004441 ) ;
#26715=CARTESIAN_POINT ( 'NONE',  ( 0.000000000000000000, -7.395377635281828788, 0.000000000000000000 ) ) ;
#26716=DIRECTION ( 'NONE',  ( 1.040834085586084257E-15, 0.000000000000000000, 1.000000000000000000 ) ) ;
#26720=CARTESIAN_POINT ( 'NONE',  ( 195.0000000000000000, 38.17226562608394147, -13.14518615778179544 ) ) ;
#26727=CARTESIAN_POINT ( 'NONE',  ( 130.0000000000000000, 33.40976562608393863, -13.14518615778179544 ) ) ;
#26728=CARTESIAN_POINT ( 'NONE',  ( 189.3771271284220177, 37.27929687716785878, 13.57481594606295161 ) ) ;
#26729=CARTESIAN_POINT ( 'NONE',  ( 181.8548138422181921, 32.76484375108393010, -5.444914386472297529 ) ) ;
#26733=AXIS2_PLACEMENT_3D ( 'NONE', #15824, #15536, #13537 ) ;
#26735=CARTESIAN_POINT ( 'NONE',  ( 65.00000000000000000, 36.53515625216787299, 13.57481594606304576 ) ) ;
#26739=CARTESIAN_POINT ( 'NONE',  ( 195.0000000000000000, 50.00000000000000000, -13.57481594606306707 ) ) ;
#26740=CARTESIAN_POINT ( 'NONE',  ( 189.5550856135277229, 40.10703125108393152, 13.14518615778179722 ) ) ;
#26743=ORIENTED_EDGE ( 'NONE', *, *, #1669, .F. ) ;
#26744=CARTESIAN_POINT ( 'NONE',  ( -0.1722897647759079331, 36.00000000000000000, -13.51468191220838122 ) ) ;
#26746=CARTESIAN_POINT ( 'NONE',  ( 143.5748159460630688, 38.32109375216786873, -1.662435489736055892E-15 ) ) ;
#26747=EDGE_CURVE ( 'NONE', #15111, #18823, #14438, .T. ) ;
#26749=CARTESIAN_POINT ( 'NONE',  ( -2.297960586008104045, 36.00000000000001421, 12.97104423350682900 ) ) ;
#26750=CARTESIAN_POINT ( 'NONE',  ( 74.29505027212704249, 32.31835937608393294, 9.295050272127046043 ) ) ;
#26753=CARTESIAN_POINT ( 'NONE',  ( -13.14518615778179189, 39.01562500108393294, 5.444914386472304635 ) ) ;
#26756=CARTESIAN_POINT ( 'NONE',  ( -9.180175813647990068, 50.00000000000000000, 9.999999999999998224 ) ) ;
#26758=CARTESIAN_POINT ( 'NONE',  ( 116.4251840539369454, 34.60039062499999574, -5.622872871577873077 ) ) ;
#26759=ORIENTED_EDGE ( 'NONE', *, *, #6735, .F. ) ;
#26764=CARTESIAN_POINT ( 'NONE',  ( 120.7049497278729575, 34.89804687608393152, -9.295050272127046043 ) ) ;
#26765=CARTESIAN_POINT ( 'NONE',  ( 55.40115559117954547, 31.67343750216787512, 9.598844408820459861 ) ) ;
#26766=EDGE_CURVE ( 'NONE', #467, #5516, #3630, .T. ) ;
#26769=CARTESIAN_POINT ( 'NONE',  ( 51.42518405393695957, 37.13046875216787868, 0.000000000000000000 ) ) ;
#26770=CARTESIAN_POINT ( 'NONE',  ( -5.444914386472299306, 39.90859375108393436, 13.14518615778179722 ) ) ;
#26774=CARTESIAN_POINT ( 'NONE',  ( 204.2950502721270425, 33.70742187608393436, 9.295050272127046043 ) ) ;
#26775=DIRECTION ( 'NONE',  ( -5.551115123125783491E-15, 0.000000000000000000, -1.000000000000000000 ) ) ;
#26777=EDGE_CURVE ( 'NONE', #11583, #18595, #13101, .T. ) ;
#26779=DIRECTION ( 'NONE',  ( -0.000000000000000000, -1.000000000000000000, -0.000000000000000000 ) ) ;
#26780=CARTESIAN_POINT ( 'NONE',  ( -8.312177448680279460E-16, 36.83281249999999574, -13.57481594606304576 ) ) ;
#26783=CARTESIAN_POINT ( 'NONE',  ( 135.6228728715777834, 38.37070312499999858, -13.57481594606313990 ) ) ;
#26789=CARTESIAN_POINT ( 'NONE',  ( 103.1528011352953342, 83.06250000136560629, -3.152801135295383084 ) ) ;
#26790=CARTESIAN_POINT ( 'NONE',  ( 74.29505027212704249, 32.31835937608393294, -9.295050272127046043 ) ) ;
#26794=CARTESIAN_POINT ( 'NONE',  ( -5.622872871577873077, 32.11992187499999574, -13.57481594606304753 ) ) ;
#26795=CARTESIAN_POINT ( 'NONE',  ( 120.7049497278729575, 36.68398437608393436, -9.295050272127046043 ) ) ;
#26796=ORIENTED_EDGE ( 'NONE', *, *, #5823, .T. ) ;
#26798=CARTESIAN_POINT ( 'NONE',  ( 104.4587341249999781, 83.87500000136560629, 1.846868145590721655 ) ) ;
#26800=CARTESIAN_POINT ( 'NONE',  ( 51.42518405393695957, 39.51171875216787299, 0.000000000000000000 ) ) ;
#26801=AXIS2_PLACEMENT_3D ( 'NONE', #4231, #25748, #6230 ) ;
#26803=CARTESIAN_POINT ( 'NONE',  ( 65.00000000000000000, 32.21914062608393436, 13.14518615778179544 ) ) ;
#26804=PRODUCT_DEFINITION_FORMATION_WITH_SPECIFIED_SOURCE ( 'ANY', '', #7403, .NOT_KNOWN. ) ;
#26807=DIRECTION ( 'NONE',  ( -0.000000000000000000, 1.000000000000000000, -0.000000000000000000 ) ) ;
#26809=ORIENTED_EDGE ( 'NONE', *, *, #11267, .F. ) ;
#26812=CARTESIAN_POINT ( 'NONE',  ( 200.6228728715778686, 34.20351562716788862, 13.57481594606304576 ) ) ;
#26813=VERTEX_POINT ( 'NONE', #22133 ) ;
#26818=CARTESIAN_POINT ( 'NONE',  ( 13.14518615778179900, 34.84843750108393579, -5.444914386472297529 ) ) ;
#26820=CARTESIAN_POINT ( 'NONE',  ( 65.00000000000000000, 32.86406249999999574, -13.57481594606304576 ) ) ;
#26833=CARTESIAN_POINT ( 'NONE',  ( -13.14518615778179900, 31.97109375108393436, -5.444914386472297529 ) ) ;
#26835=CARTESIAN_POINT ( 'NONE',  ( -5.622872871577965448, 37.97382812499999716, 13.57481594606295161 ) ) ;
#26836=CARTESIAN_POINT ( 'NONE',  ( -5.622872871577920151, 36.08867187500000284, -13.57481594606300135 ) ) ;
#26837=CARTESIAN_POINT ( 'NONE',  ( 195.0000000000000000, 36.78320312608393294, 13.14518615778179544 ) ) ;
#26838=ORIENTED_EDGE ( 'NONE', *, *, #5660, .F. ) ;
#26839=CARTESIAN_POINT ( 'NONE',  ( 194.2802394038907323, 53.51499872091920906, -14.99999999999999645 ) ) ;
#26844=AXIS2_PLACEMENT_3D ( 'NONE', #8635, #24028, #23608 ) ;
#26846=CARTESIAN_POINT ( 'NONE',  ( 130.0000000000000000, 40.00781250000000000, -13.57481594606304576 ) ) ;
#26847=STYLED_ITEM ( 'NONE', ( #5508 ), #7448 ) ;
#26848=CARTESIAN_POINT ( 'NONE',  ( 116.8548138422182205, 36.58476562608393579, 0.000000000000000000 ) ) ;
#26849=CARTESIAN_POINT ( 'NONE',  ( -13.14518615778179189, 39.21406250108392300, 5.444914386472304635 ) ) ;
#26850=CARTESIAN_POINT ( 'NONE',  ( -13.14518615778179544, 34.20351562608393436, 0.000000000000000000 ) ) ;
#26853=CARTESIAN_POINT ( 'NONE',  ( -5.622872871577804688, 36.48554687716787726, 13.57481594606311504 ) ) ;
#26855=CARTESIAN_POINT ( 'NONE',  ( 181.4251840539369596, 39.46210937499999005, 5.622872871577880183 ) ) ;
#26856=ORIENTED_EDGE ( 'NONE', *, *, #9121, .T. ) ;
#26857=CARTESIAN_POINT ( 'NONE',  ( 74.43200616963319760, 36.00000000000000000, 9.391769196591081226 ) ) ;
#26861=CARTESIAN_POINT ( 'NONE',  ( 70.44491438647229131, 36.33671875108393579, -13.14518615778179722 ) ) ;
#26863=CARTESIAN_POINT ( 'NONE',  ( 195.0000000000000000, 36.38632812608393152, -13.14518615778179544 ) ) ;
#26868=CARTESIAN_POINT ( 'NONE',  ( 200.4449143864723055, 37.32890625108393579, -13.14518615778179722 ) ) ;
#26870=ORIENTED_EDGE ( 'NONE', *, *, #20317, .F. ) ;
#26873=EDGE_LOOP ( 'NONE', ( #11722, #7751, #10589, #23390 ) ) ;
#26874=CARTESIAN_POINT ( 'NONE',  ( 133.7556399192858976, 31.78804746655075419, -13.14518615778179544 ) ) ;
#26876=ORIENTED_EDGE ( 'NONE', *, *, #18574, .T. ) ;
#26877=CARTESIAN_POINT ( 'NONE',  ( 185.7049497278729575, 32.91367187608393152, 9.295050272127047819 ) ) ;
#26880=CARTESIAN_POINT ( 'NONE',  ( 9.180175813647991845, 55.00000000000000000, -15.00000000000000000 ) ) ;
#26882=CARTESIAN_POINT ( 'NONE',  ( 135.6228728715778971, 38.96601562716787015, 13.57481594606304576 ) ) ;
#26887=CARTESIAN_POINT ( 'NONE',  ( 208.1451861577817795, 40.30546875108393579, 5.444914386472293977 ) ) ;
#26889=ORIENTED_EDGE ( 'NONE', *, *, #14429, .T. ) ;
#26890=CARTESIAN_POINT ( 'NONE',  ( -9.078091922698781957, 36.00000000000000711, -9.794392408849049048 ) ) ;
#26893=CARTESIAN_POINT ( 'NONE',  ( -9.713547494049105779, 35.99999999999998579, 8.898183052316493757 ) ) ;
#26894=DIRECTION ( 'NONE',  ( -2.385244779468110248E-16, 0.000000000000000000, -1.000000000000000000 ) ) ;
#26900=CARTESIAN_POINT ( 'NONE',  ( 143.5748159460630688, 40.55351562499999574, 5.622872871577868636 ) ) ;
#26901=CARTESIAN_POINT ( 'NONE',  ( 143.5748159460630404, 33.40976562499999858, 5.622872871577869525 ) ) ;
#26902=VERTEX_POINT ( 'NONE', #18672 ) ;
#26903=CYLINDRICAL_SURFACE ( 'NONE', #18134, 4.999999999999999112 ) ;
#26904=EDGE_CURVE ( 'NONE', #15733, #26226, #18161, .T. ) ;
#26908=CARTESIAN_POINT ( 'NONE',  ( 135.4449143864723055, 32.86406250108392868, 13.14518615778179189 ) ) ;
#26909=CARTESIAN_POINT ( 'NONE',  ( 78.14518615778179367, 38.51953125108393294, 5.444914386472293977 ) ) ;
#26911=LINE ( 'NONE', #542, #9768 ) ;
#26912=CARTESIAN_POINT ( 'NONE',  ( 13.14518615778179900, 38.61875000108393152, -5.444914386472297529 ) ) ;
#26918=CARTESIAN_POINT ( 'NONE',  ( 103.5355339059327093, 82.50000000273119838, 3.535533905932726206 ) ) ;
#26919=CARTESIAN_POINT ( 'NONE',  ( 195.0000000000000000, -7.395377635281828788, -2.255140518769849538E-14 ) ) ;
#26921=CARTESIAN_POINT ( 'NONE',  ( 116.9040934463640156, 36.00000000000000000, 1.137167824541468031 ) ) ;
#26922=CARTESIAN_POINT ( 'NONE',  ( 133.6286142932849259, 36.00000000000002132, -13.08307257738123219 ) ) ;
#26923=EDGE_CURVE ( 'NONE', #13869, #18001, #14944, .T. ) ;
#26934=CARTESIAN_POINT ( 'NONE',  ( 99.99999999999995737, 82.18750000136559208, -4.458734125000016313 ) ) ;
#26935=CARTESIAN_POINT ( 'NONE',  ( 51.85481384221819923, 32.56640625108394005, -5.444914386472297529 ) ) ;
#26938=EDGE_CURVE ( 'NONE', #10403, #26695, #22215, .T. ) ;
#26939=CARTESIAN_POINT ( 'NONE',  ( 2.493653234604083739E-15, 37.22968749999999716, 13.57481594606304576 ) ) ;
#26940=CARTESIAN_POINT ( 'NONE',  ( 130.0000000000000000, 34.60039062608393579, 13.14518615778179544 ) ) ;
#26941=ORIENTED_EDGE ( 'NONE', *, *, #1016, .T. ) ;
#26942=CARTESIAN_POINT ( 'NONE',  ( 99.99999999999995737, 80.75000000000000000, -5.000000000000018652 ) ) ;
#26943=EDGE_CURVE ( 'NONE', #24277, #17678, #25123, .T. ) ;
#26945=CARTESIAN_POINT ( 'NONE',  ( 96.84719886470459471, 84.31250000136560629, -3.152801135295383084 ) ) ;
#26947=CARTESIAN_POINT ( 'NONE',  ( 116.4251840539369738, 38.66835937499999432, 5.622872871577880183 ) ) ;
#26948=EDGE_CURVE ( 'NONE', #12117, #1457, #17745, .T. ) ;
#26950=CARTESIAN_POINT ( 'NONE',  ( 74.59884440882045453, 39.71015624999999716, 9.598844408820456309 ) ) ;
#26951=CARTESIAN_POINT ( 'NONE',  ( 13.57481594606304931, 37.47773437716787726, 5.622872871577869525 ) ) ;
#26953=CARTESIAN_POINT ( 'NONE',  ( 184.4540428948961335, 35.99999999999997868, -8.172591786207139108 ) ) ;
#26955=EDGE_CURVE ( 'NONE', #13505, #11663, #23609, .T. ) ;
#26956=ORIENTED_EDGE ( 'NONE', *, *, #2185, .T. ) ;
#26958=CARTESIAN_POINT ( 'NONE',  ( 195.0000000000000000, 39.95820312608393010, 13.14518615778179544 ) ) ;
#26962=CARTESIAN_POINT ( 'NONE',  ( -8.049105076161786076E-16, 34.20351562608394147, -13.14518615778179544 ) ) ;
#26963=CARTESIAN_POINT ( 'NONE',  ( 135.4449143864723055, 33.16171875108393152, -13.14518615778179900 ) ) ;
#26967=CARTESIAN_POINT ( 'NONE',  ( 78.57481594606305464, 36.73359375216787015, -1.662435489736055892E-15 ) ) ;
#26973=FACE_OUTER_BOUND ( 'NONE', #7310, .T. ) ;
#26974=CARTESIAN_POINT ( 'NONE',  ( 13.14518615778179544, 32.41757812608393863, -1.609821015232357215E-15 ) ) ;
#26975=VERTEX_POINT ( 'NONE', #4783 ) ;
#26976=CARTESIAN_POINT ( 'NONE',  ( 195.0000000000000000, -7.395377635281828788, -13.57481594606306707 ) ) ;
#26980=ADVANCED_FACE ( 'NONE', ( #26154 ), #23878, .T. ) ;
#26981=CARTESIAN_POINT ( 'NONE',  ( 204.2950502721270425, 37.08085937608393579, -9.295050272127046043 ) ) ;
#26982=ORIENTED_EDGE ( 'NONE', *, *, #12095, .F. ) ;
#26983=CARTESIAN_POINT ( 'NONE',  ( -5.622872871577804688, 37.18007812499999432, 13.57481594606311504 ) ) ;
#26985=ORIENTED_EDGE ( 'NONE', *, *, #14200, .F. ) ;
#26990=CARTESIAN_POINT ( 'NONE',  ( 130.0000000000000000, 38.37070312608393152, 13.14518615778179544 ) ) ;
#26991=CARTESIAN_POINT ( 'NONE',  ( 9.295050272127046043, 38.07304687608393579, -9.295050272127046043 ) ) ;
#26992=CARTESIAN_POINT ( 'NONE',  ( -5.444914386472299306, 36.73359375108393010, 13.14518615778179722 ) ) ;
#26994=CARTESIAN_POINT ( 'NONE',  ( 64.27612806197501527, 53.51529642094997996, -14.99999999999999822 ) ) ;
#26996=AXIS2_PLACEMENT_3D ( 'NONE', #9329, #9194, #17888 ) ;
#26997=CARTESIAN_POINT ( 'NONE',  ( -13.57481594606304398, 37.18007812716787441, 5.622872871577880183 ) ) ;
#27000=CARTESIAN_POINT ( 'NONE',  ( 78.14518615778179367, 36.98164062608393010, -1.609821015232357215E-15 ) ) ;
#27003=CARTESIAN_POINT ( 'NONE',  ( -15.00000000000000355, 75.00000000000000000, -9.999999999999998224 ) ) ;
#27008=CARTESIAN_POINT ( 'NONE',  ( 208.1451861577818079, 37.13046875108393863, 5.444914386472293977 ) ) ;
#27013=ORIENTED_EDGE ( 'NONE', *, *, #19102, .F. ) ;
#27014=CARTESIAN_POINT ( 'NONE',  ( 120.7049497278729575, 31.92148437608393508, -9.295050272127046043 ) ) ;
#27015=CARTESIAN_POINT ( 'NONE',  ( 78.14518615778180788, 40.30546875108393579, 5.444914386472293977 ) ) ;
#27016=CYLINDRICAL_SURFACE ( 'NONE', #19152, 11.57481594606304398 ) ;
#27018=CARTESIAN_POINT ( 'NONE',  ( 181.8548138422181921, 34.45156250108394147, 5.444914386472304635 ) ) ;
#27019=( BOUNDED_CURVE ( )  B_SPLINE_CURVE ( 2, ( #6694, #24376, #2727, #10821, #26092, #4293, #161, #6557, #13530 ),
 .UNSPECIFIED., .F., .F. ) 
 B_SPLINE_CURVE_WITH_KNOTS ( ( 3, 2, 2, 2, 3 ),
 ( 0.02083333333333358892, 0.03125000000000020123, 0.04166666666666681007, 0.05208333333333342585, 0.06250000000000004163 ),
 .UNSPECIFIED. ) 
 CURVE ( )  GEOMETRIC_REPRESENTATION_ITEM ( )  RATIONAL_B_SPLINE_CURVE ( ( 0.9999999999999981126, 0.9238795325112886259, 1.000000000000000000, 0.9238795325112867385, 1.000000000000000000, 0.9238795325112867385, 1.000000000000000000, 0.9238795325112864054, 1.000000000000000222 ) ) 
 REPRESENTATION_ITEM ( '' )  );
#27020=VERTEX_POINT ( 'NONE', #26735 ) ;
#27021=CARTESIAN_POINT ( 'NONE',  ( 65.00000000000000000, 37.62656249999999858, -13.57481594606304576 ) ) ;
#27024=CARTESIAN_POINT ( 'NONE',  ( 139.5988444088204403, 38.42031250216787441, -9.598844408820458085 ) ) ;
#27027=CARTESIAN_POINT ( 'NONE',  ( 71.41286667625729478, 50.00000000108468612, 11.99502265407483570 ) ) ;
#27028=ORIENTED_EDGE ( 'NONE', *, *, #8879, .F. ) ;
#27029=VERTEX_POINT ( 'NONE', #82 ) ;
#27032=ORIENTED_EDGE ( 'NONE', *, *, #23377, .F. ) ;
#27033=CARTESIAN_POINT ( 'NONE',  ( 3.628614293284873948, 36.00000000000000711, -13.08307257738123219 ) ) ;
#27036=CARTESIAN_POINT ( 'NONE',  ( 181.4251840539369596, 40.25585937716787299, -5.622872871577872189 ) ) ;
#27040=CARTESIAN_POINT ( 'NONE',  ( -13.57481594606304576, 38.61874999999999147, 0.000000000000000000 ) ) ;
#27041=FACE_OUTER_BOUND ( 'NONE', #8508, .T. ) ;
#27042=CARTESIAN_POINT ( 'NONE',  ( 2.276146844546785175, 51.46995505939283788, 15.00000000000000178 ) ) ;
#27043=SPHERICAL_SURFACE ( 'NONE', #1956, 5.000000000000000000 ) ;
#27044=CARTESIAN_POINT ( 'NONE',  ( 139.5988444088204687, 33.36015624999999574, 9.598844408820456309 ) ) ;
#27045=ORIENTED_EDGE ( 'NONE', *, *, #18240, .T. ) ;
#27049=CARTESIAN_POINT ( 'NONE',  ( 143.1451861577818079, 32.26875000108393721, -5.444914386472297529 ) ) ;
#27050=CARTESIAN_POINT ( 'NONE',  ( 78.14518615778179367, 39.41250000108393436, -5.444914386472297529 ) ) ;
#27051=DIRECTION ( 'NONE',  ( 0.000000000000000000, 0.000000000000000000, 1.000000000000000000 ) ) ;
#27052=CARTESIAN_POINT ( 'NONE',  ( -9.295050272127046043, 38.07304687608393579, -9.295050272127046043 ) ) ;
#27057=EDGE_CURVE ( 'NONE', #25242, #20160, #21752, .T. ) ;
#27059=CARTESIAN_POINT ( 'NONE',  ( 208.1451861577818079, 32.21914062608393436, -1.609821015232357215E-15 ) ) ;
#27060=FACE_OUTER_BOUND ( 'NONE', #21739, .T. ) ;
#27063=CARTESIAN_POINT ( 'NONE',  ( 181.4251840539369596, 39.41249999999999432, 0.000000000000000000 ) ) ;
#27065=CARTESIAN_POINT ( 'NONE',  ( 200.6228728715777549, 38.96601562716787015, 13.57481594606318076 ) ) ;
#27073=CARTESIAN_POINT ( 'NONE',  ( 59.55508561352770158, 33.26093750108393721, -13.14518615778179900 ) ) ;
#27074=DIRECTION ( 'NONE',  ( -0.000000000000000000, 1.000000000000000000, -0.000000000000000000 ) ) ;
#27077=CARTESIAN_POINT ( 'NONE',  ( 3.878385297391210518, 32.03609435653363136, -13.57481594606304576 ) ) ;
#27079=CARTESIAN_POINT ( 'NONE',  ( 135.4449143864723055, 34.65000000108393863, 13.14518615778179189 ) ) ;
#27081=CARTESIAN_POINT ( 'NONE',  ( 104.9999999999999574, 80.43750000000001421, 2.071067811865462627 ) ) ;
#27083=CARTESIAN_POINT ( 'NONE',  ( 104.9999999999999716, 79.62500000273119838, -1.449011120738813565E-14 ) ) ;
#27085=CARTESIAN_POINT ( 'NONE',  ( 59.37712712842213136, 39.66054687716786731, 13.57481594606304753 ) ) ;
#27086=ADVANCED_FACE ( 'NONE', ( #2227 ), #12368, .T. ) ;
#27089=CARTESIAN_POINT ( 'NONE',  ( 185.7049497278729575, 31.72304687608393081, -9.295050272127046043 ) ) ;
#27094=ORIENTED_EDGE ( 'NONE', *, *, #22226, .T. ) ;
#27096=CARTESIAN_POINT ( 'NONE',  ( 189.3771271284221314, 32.21914062716787441, -13.57481594606304753 ) ) ;
#27100=CARTESIAN_POINT ( 'NONE',  ( 143.1451861577818079, 40.15664062608393436, -1.609821015232357215E-15 ) ) ;
#27103=CARTESIAN_POINT ( 'NONE',  ( 130.0000000000000000, 31.62382812608393579, -13.14518615778179544 ) ) ;
#27109=CARTESIAN_POINT ( 'NONE',  ( -13.57481594606304398, 37.97382812716787726, 5.622872871577880183 ) ) ;
#27110=AXIS2_PLACEMENT_3D ( 'NONE', #13762, #24477, #22485 ) ;
#27116=CARTESIAN_POINT ( 'NONE',  ( 5.444914386472297529, 34.15390625108393863, -13.14518615778179900 ) ) ;
#27118=ORIENTED_EDGE ( 'NONE', *, *, #1638, .T. ) ;
#27122=CARTESIAN_POINT ( 'NONE',  ( 181.8548138422181921, 35.74140625108393721, -5.444914386472297529 ) ) ;
#27123=ORIENTED_EDGE ( 'NONE', *, *, #3260, .F. ) ;
#27124=CARTESIAN_POINT ( 'NONE',  ( 198.8639252651224467, 54.10645156200647676, -14.99999999999999645 ) ) ;
#27129=AXIS2_PLACEMENT_3D ( 'NONE', #8980, #26378, #2952 ) ;
#27131=DIRECTION ( 'NONE',  ( -0.000000000000000000, 1.000000000000000000, -0.000000000000000000 ) ) ;
#27133=CARTESIAN_POINT ( 'NONE',  ( 124.5550856135277087, 36.73359375108393010, 13.14518615778179722 ) ) ;
#27134=CARTESIAN_POINT ( 'NONE',  ( -9.295050272127046043, 38.27148437608393294, -9.295050272127046043 ) ) ;
#27135=CARTESIAN_POINT ( 'NONE',  ( 2.414731522848535132E-15, 33.60820312608392868, 13.14518615778179544 ) ) ;
#27136=EDGE_CURVE ( 'NONE', #18595, #16904, #28040, .T. ) ;
#27146=CARTESIAN_POINT ( 'NONE',  ( 55.70494972787295751, 38.07304687608393579, -9.295050272127046043 ) ) ;
#27147=CARTESIAN_POINT ( 'NONE',  ( -13.57481594606304753, 38.66835937716787441, -5.622872871577872189 ) ) ;
#27149=CARTESIAN_POINT ( 'NONE',  ( 189.5550856135277229, 36.43593750108394147, -13.14518615778179722 ) ) ;
#27161=CARTESIAN_POINT ( 'NONE',  ( 65.00000000000000000, 40.15664062608393436, 13.14518615778179544 ) ) ;
#27163=CARTESIAN_POINT ( 'NONE',  ( 185.7049497278729575, 34.50117187608393721, 9.295050272127047819 ) ) ;
#27164=ORIENTED_EDGE ( 'NONE', *, *, #1041, .T. ) ;
#27165=DIRECTION ( 'NONE',  ( 0.000000000000000000, 1.000000000000000000, 0.000000000000000000 ) ) ;
#27166=CARTESIAN_POINT ( 'NONE',  ( 6.902378573780021398, 51.13402819307184188, -15.00000000000129141 ) ) ;
#27169=CARTESIAN_POINT ( 'NONE',  ( 116.4251840539369596, 37.92421875216787441, 0.000000000000000000 ) ) ;
#27170=VECTOR ( 'NONE', #18291, 1000.000000000000000 ) ;
#27173=CARTESIAN_POINT ( 'NONE',  ( 181.8548138422182205, 39.16445312608393436, 0.000000000000000000 ) ) ;
#27177=AXIS2_PLACEMENT_3D ( 'NONE', #27500, #21213, #25905 ) ;
#27179=CARTESIAN_POINT ( 'NONE',  ( 208.5748159460630688, 38.17226562499999432, 5.622872871577868636 ) ) ;
#27180=CARTESIAN_POINT ( 'NONE',  ( 181.4251840539369596, 40.30546875216787583, 0.000000000000000000 ) ) ;
#27181=CARTESIAN_POINT ( 'NONE',  ( 65.00000000000000000, 32.21914062608393436, 13.14518615778179544 ) ) ;
#27184=CARTESIAN_POINT ( 'NONE',  ( 13.57481594606304753, 40.65273437499999432, -5.622872871577873966 ) ) ;
#27188=CARTESIAN_POINT ( 'NONE',  ( 143.5748159460630688, 34.25312499999999716, -1.662435489736055892E-15 ) ) ;
#27189=ORIENTED_EDGE ( 'NONE', *, *, #19777, .F. ) ;
#27190=DIRECTION ( 'NONE',  ( 0.000000000000000000, 1.000000000000000000, 0.000000000000000000 ) ) ;
#27191=( BOUNDED_CURVE ( )  B_SPLINE_CURVE ( 2, ( #8500, #19472, #8776, #6360, #19610, #2659, #15034, #8640, #17758 ),
 .UNSPECIFIED., .F., .F. ) 
 B_SPLINE_CURVE_WITH_KNOTS ( ( 3, 2, 2, 2, 3 ),
 ( 0.2291666666666665741, 0.2395833333333332316, 0.2499999999999998335, 0.2604166666666665186, 0.2708333333333330928 ),
 .UNSPECIFIED. ) 
 CURVE ( )  GEOMETRIC_REPRESENTATION_ITEM ( )  RATIONAL_B_SPLINE_CURVE ( ( 1.000000000000000666, 0.9238795325112861834, 1.000000000000000000, 0.9238795325112867385, 1.000000000000000000, 0.9238795325112867385, 1.000000000000000000, 0.9238795325112884038, 0.9999999999999983347 ) ) 
 REPRESENTATION_ITEM ( '' )  );
#27196=CARTESIAN_POINT ( 'NONE',  ( 124.5550856135277087, 38.22187500108393010, -13.14518615778179900 ) ) ;
#27197=CARTESIAN_POINT ( 'NONE',  ( 78.57481594606305464, 31.97109375216787441, -1.662435489736055892E-15 ) ) ;
#27198=CARTESIAN_POINT ( 'NONE',  ( 5.622872871577780707, 37.67617187716787441, -13.57481594606313990 ) ) ;
#27199=CARTESIAN_POINT ( 'NONE',  ( 5.444914386472302859, 39.21406250108392300, 13.14518615778179189 ) ) ;
#27201=CARTESIAN_POINT ( 'NONE',  ( 59.37712712842213136, 37.67617187499999432, -13.57481594606304753 ) ) ;
#27203=CARTESIAN_POINT ( 'NONE',  ( 200.6228728715779823, 40.75195312499999289, -13.57481594606294095 ) ) ;
#27204=FACE_OUTER_BOUND ( 'NONE', #9030, .T. ) ;
#27205=CARTESIAN_POINT ( 'NONE',  ( 137.0656349887609053, 35.99999999999999289, 11.21307450592200539 ) ) ;
#27208=CARTESIAN_POINT ( 'NONE',  ( 181.4251840539369596, 39.36289062499999858, -5.622872871577872189 ) ) ;
#27209=DIRECTION ( 'NONE',  ( -0.000000000000000000, 1.000000000000000000, -0.000000000000000000 ) ) ;
#27213=CARTESIAN_POINT ( 'NONE',  ( 189.3771271284221314, 32.91367187499999858, -13.57481594606304753 ) ) ;
#27216=CARTESIAN_POINT ( 'NONE',  ( 96.84719886470459471, 84.31250000136560629, -3.152801135295383084 ) ) ;
#27217=CARTESIAN_POINT ( 'NONE',  ( 65.00000000000000000, 31.62382812608393579, -13.14518615778179544 ) ) ;
#27221=CARTESIAN_POINT ( 'NONE',  ( 9.598844408820459861, 33.36015624999999574, 9.598844408820456309 ) ) ;
#27223=CARTESIAN_POINT ( 'NONE',  ( 135.4449143864723055, 33.85625000108393579, 13.14518615778179189 ) ) ;
#27226=EDGE_CURVE ( 'NONE', #18595, #11873, #18678, .T. ) ;
#27227=CARTESIAN_POINT ( 'NONE',  ( 130.0000000000000000, -7.395377635281828788, -1.503427012513233026E-14 ) ) ;
#27228=CARTESIAN_POINT ( 'NONE',  ( 99.99999999999995737, 81.68750000136559208, 4.458734124999988779 ) ) ;
#27230=CARTESIAN_POINT ( 'NONE',  ( 195.0000000000000000, 37.62656249999999858, -13.57481594606304576 ) ) ;
#27232=CARTESIAN_POINT ( 'NONE',  ( 195.0000000000000000, 39.75976562608394005, -13.14518615778179544 ) ) ;
#27233=CARTESIAN_POINT ( 'NONE',  ( -5.622872871577873077, 38.86679687716788578, 13.57481594606304753 ) ) ;
#27238=CARTESIAN_POINT ( 'NONE',  ( 181.8548138422182205, 40.55351562608393579, 0.000000000000000000 ) ) ;
#27242=CARTESIAN_POINT ( 'NONE',  ( -5.444914386472299306, 32.16953125108393152, 13.14518615778179722 ) ) ;
#27244=CARTESIAN_POINT ( 'NONE',  ( 59.37712712842213136, 32.41757812499999858, 13.57481594606304753 ) ) ;
#27249=CARTESIAN_POINT ( 'NONE',  ( 2.493653234604083739E-15, 38.12265625216787157, 13.57481594606304576 ) ) ;
#27255=CARTESIAN_POINT ( 'NONE',  ( -9.295050272127044266, 33.70742187608393436, 9.295050272127047819 ) ) ;
#27257=ORIENTED_EDGE ( 'NONE', *, *, #7391, .T. ) ;
#27260=CARTESIAN_POINT ( 'NONE',  ( 2.493653234604083739E-15, 37.22968749999999716, 13.57481594606304576 ) ) ;
#27262=CARTESIAN_POINT ( 'NONE',  ( 189.5550856135277229, 34.05468750108393294, -13.14518615778179900 ) ) ;
#27264=CARTESIAN_POINT ( 'NONE',  ( 202.1154903918443608, 49.99999999945652718, -11.58166858714790592 ) ) ;
#27269=CARTESIAN_POINT ( 'NONE',  ( 189.3771271284221314, 39.36289062716787157, -13.57481594606304753 ) ) ;
#27271=AXIS2_PLACEMENT_3D ( 'NONE', #14904, #23625, #16648 ) ;
#27273=CARTESIAN_POINT ( 'NONE',  ( 13.14518615778179544, 36.38632812608393863, -1.609821015232357215E-15 ) ) ;
#27274=CARTESIAN_POINT ( 'NONE',  ( -8.049105076161786076E-16, 31.62382812608393579, -13.14518615778179544 ) ) ;
#27277=ORIENTED_EDGE ( 'NONE', *, *, #1683, .T. ) ;
#27278=CARTESIAN_POINT ( 'NONE',  ( -9.598844408820458085, 37.03125000216787299, -9.598844408820458085 ) ) ;
#27281=CARTESIAN_POINT ( 'NONE',  ( 95.54126587499996504, 82.62500000136560629, -1.846868145590750077 ) ) ;
#27283=CARTESIAN_POINT ( 'NONE',  ( 181.4251840539369596, 38.66835937499999432, 5.622872871577880183 ) ) ;
#27284=ORIENTED_EDGE ( 'NONE', *, *, #14023, .F. ) ;
#27287=EDGE_CURVE ( 'NONE', #22301, #20134, #14783, .T. ) ;
#27290=CARTESIAN_POINT ( 'NONE',  ( 200.4449143864723055, 36.23750000108393721, 13.14518615778179189 ) ) ;
#27296=CARTESIAN_POINT ( 'NONE',  ( 78.14518615778180788, 37.92421875108393436, 5.444914386472293977 ) ) ;
#27297=ADVANCED_FACE ( 'NONE', ( #7699 ), #16392, .T. ) ;
#27299=CARTESIAN_POINT ( 'NONE',  ( 201.9444263933115167, 31.75150625057403175, -11.16113171639042356 ) ) ;
#27301=CARTESIAN_POINT ( 'NONE',  ( 78.57481594606305464, 37.42812499999999432, -1.662435489736055892E-15 ) ) ;
#27302=CARTESIAN_POINT ( 'NONE',  ( 1.138768117104975941, 50.00000000043849013, -13.56816686242529357 ) ) ;
#27305=CARTESIAN_POINT ( 'NONE',  ( 130.0000000000000000, 38.91640625216786731, 13.57481594606304576 ) ) ;
#27309=CARTESIAN_POINT ( 'NONE',  ( 200.4449143864723055, 37.82500000108392868, 13.14518615778179189 ) ) ;
#27310=VERTEX_POINT ( 'NONE', #14518 ) ;
#27313=CARTESIAN_POINT ( 'NONE',  ( 4.157286354961724939, 36.00000000000000000, -12.92256159328856135 ) ) ;
#27314=CARTESIAN_POINT ( 'NONE',  ( 9.598844408820459861, 39.71015624999999716, 9.598844408820456309 ) ) ;
#27316=CARTESIAN_POINT ( 'NONE',  ( 99.99999999999995737, 84.18750000136560629, -4.458734125000016313 ) ) ;
#27317=CARTESIAN_POINT ( 'NONE',  ( 78.14518615778179367, 32.36796875108393579, 5.444914386472293977 ) ) ;
#27320=CARTESIAN_POINT ( 'NONE',  ( -8.312177448680279460E-16, 38.42031249999999432, -13.57481594606304576 ) ) ;
#27322=CYLINDRICAL_SURFACE ( 'NONE', #15911, 13.57481594606304398 ) ;
#27323=CARTESIAN_POINT ( 'NONE',  ( 143.5748159460630404, 34.20351562499999432, 5.622872871577869525 ) ) ;
#27324=EDGE_LOOP ( 'NONE', ( #11272, #19433, #15979, #27123 ) ) ;
#27325=CARTESIAN_POINT ( 'NONE',  ( 99.99999999999995737, 78.00000000000000000, 2.999999999999990674 ) ) ;
#27329=CARTESIAN_POINT ( 'NONE',  ( 135.4449143864723055, 39.71015625108393010, -13.14518615778179900 ) ) ;
#27330=CARTESIAN_POINT ( 'NONE',  ( 65.00000000000000000, 39.56132812608393579, -13.14518615778179544 ) ) ;
#27331=ADVANCED_FACE ( 'NONE', ( #14242 ), #5714, .F. ) ;
#27333=CARTESIAN_POINT ( 'NONE',  ( -13.14518615778179544, 39.75976562608393294, 0.000000000000000000 ) ) ;
#27335=DIRECTION ( 'NONE',  ( -0.000000000000000000, 1.000000000000000000, -0.000000000000000000 ) ) ;
#27337=CIRCLE ( 'NONE', #7289, 13.57481594606304398 ) ;
#27338=FACE_OUTER_BOUND ( 'NONE', #15934, .T. ) ;
#27339=CARTESIAN_POINT ( 'NONE',  ( 102.0710678118654329, 82.81250000273118417, -5.000000000000004441 ) ) ;
#27340=DIRECTION ( 'NONE',  ( -0.000000000000000000, 1.000000000000000000, -0.000000000000000000 ) ) ;
#27343=CARTESIAN_POINT ( 'NONE',  ( 129.0044387749465216, 36.00000000000000000, -13.45766439703019302 ) ) ;
#27345=CARTESIAN_POINT ( 'NONE',  ( 99.99999999999995737, 85.00000000000000000, 4.999999999999990230 ) ) ;
#27348=ORIENTED_EDGE ( 'NONE', *, *, #4251, .F. ) ;
#27355=CARTESIAN_POINT ( 'NONE',  ( 96.84719886470459471, 79.56250000136559208, 3.152801135295355994 ) ) ;
#27356=CARTESIAN_POINT ( 'NONE',  ( 59.55508561352770158, 31.97109375108393436, 13.14518615778179722 ) ) ;
#27360=CARTESIAN_POINT ( 'NONE',  ( 143.5748159460630688, 38.96601562499999005, 5.622872871577868636 ) ) ;
#27362=CARTESIAN_POINT ( 'NONE',  ( 120.7049497278729575, 35.89023437608393152, -9.295050272127046043 ) ) ;
#27364=CARTESIAN_POINT ( 'NONE',  ( 3.865414375413191106, 54.10683252460150783, -15.00000000000000533 ) ) ;
#27365=CYLINDRICAL_SURFACE ( 'NONE', #7123, 13.57481594606304398 ) ;
#27366=CARTESIAN_POINT ( 'NONE',  ( 98.15313185440925281, 82.62500000136560629, 4.458734124999987891 ) ) ;
#27367=CARTESIAN_POINT ( 'NONE',  ( 124.3771271284221598, 38.76757812499998579, 13.57481594606308128 ) ) ;
#27369=CARTESIAN_POINT ( 'NONE',  ( 2.493653234604083739E-15, 38.12265625216787157, 13.57481594606304576 ) ) ;
#27372=ORIENTED_EDGE ( 'NONE', *, *, #4038, .F. ) ;
#27374=CARTESIAN_POINT ( 'NONE',  ( 204.2950502721270425, 40.05742187608392868, 9.295050272127046043 ) ) ;
#27377=CARTESIAN_POINT ( 'NONE',  ( 139.2950502721270425, 37.67617187608393436, 9.295050272127046043 ) ) ;
#27378=LINE ( 'NONE', #5713, #3602 ) ;
#27379=EDGE_CURVE ( 'NONE', #20261, #15363, #122, .T. ) ;
#27383=CARTESIAN_POINT ( 'NONE',  ( 195.0000000000000000, 40.40468749999999432, 13.57481594606304576 ) ) ;
#27385=CARTESIAN_POINT ( 'NONE',  ( 131.1371678245417627, 36.00000000000000000, 13.09590655363595602 ) ) ;
#27393=CARTESIAN_POINT ( 'NONE',  ( -13.14518615778179189, 32.07031250108393294, 5.444914386472304635 ) ) ;
#27394=EDGE_LOOP ( 'NONE', ( #6659, #11525, #19416, #20707, #6334, #19816 ) ) ;
#27395=CARTESIAN_POINT ( 'NONE',  ( 104.4587341249999781, 83.25000000136560629, -1.846868145590750299 ) ) ;
#27397=CARTESIAN_POINT ( 'NONE',  ( 189.5550856135277229, 33.55859375108393294, 13.14518615778179722 ) ) ;
#27399=CARTESIAN_POINT ( 'NONE',  ( -13.57481594606304398, 37.08085937499999574, 5.622872871577880183 ) ) ;
#27401=VERTEX_POINT ( 'NONE', #17497 ) ;
#27404=CARTESIAN_POINT ( 'NONE',  ( 99.99999999999995737, 85.00000000000000000, -1.387778780781445676E-14 ) ) ;
#27406=CARTESIAN_POINT ( 'NONE',  ( 13.14518615778179722, 37.13046875108393863, 5.444914386472293977 ) ) ;
#27407=CARTESIAN_POINT ( 'NONE',  ( 13.14518615778179900, 33.75703125108393010, 5.444914386472293977 ) ) ;
#27412=CARTESIAN_POINT ( 'NONE',  ( 98.15313185440923860, 81.50000000136560629, -4.458734125000016313 ) ) ;
#27414=CARTESIAN_POINT ( 'NONE',  ( 74.59884440882045453, 39.21406250216787015, -9.598844408820458085 ) ) ;
#27424=VERTEX_POINT ( 'NONE', #24061 ) ;
#27425=CARTESIAN_POINT ( 'NONE',  ( 55.70494972787295751, 36.68398437608393436, -9.295050272127046043 ) ) ;
#27431=CARTESIAN_POINT ( 'NONE',  ( -7.089417272331180797, 49.99999999943663909, -11.59823041029098256 ) ) ;
#27432=CARTESIAN_POINT ( 'NONE',  ( 143.5748159460630688, 36.78320312716788010, -5.622872871577873966 ) ) ;
#27433=CARTESIAN_POINT ( 'NONE',  ( 130.0000000000000000, 37.32890625216786873, 13.57481594606304576 ) ) ;
#27435=EDGE_CURVE ( 'NONE', #1080, #20134, #27712, .T. ) ;
#27437=CARTESIAN_POINT ( 'NONE',  ( 195.0000000000000000, 37.37851562608393863, -13.14518615778179544 ) ) ;
#27439=EDGE_CURVE ( 'NONE', #21288, #439, #4399, .T. ) ;
#27440=ORIENTED_EDGE ( 'NONE', *, *, #20510, .F. ) ;
#27443=CARTESIAN_POINT ( 'NONE',  ( 96.46446609406721961, 83.87500000000000000, -3.535533905932755072 ) ) ;
#27446=CARTESIAN_POINT ( 'NONE',  ( 98.15313185440923860, 83.25000000136559208, -4.458734125000016313 ) ) ;
#27448=CARTESIAN_POINT ( 'NONE',  ( 94.99999999999995737, 79.12500000273118417, -1.387778780781445676E-14 ) ) ;
#27450=CARTESIAN_POINT ( 'NONE',  ( 94.99999999999995737, 81.00000000000000000, -1.387778780781445676E-14 ) ) ;
#27451=CARTESIAN_POINT ( 'NONE',  ( 6.351932228771040023, 35.99999999999999289, 11.61660627739524543 ) ) ;
#27454=ORIENTED_EDGE ( 'NONE', *, *, #18072, .T. ) ;
#27455=AXIS2_PLACEMENT_3D ( 'NONE', #13366, #22374, #19950 ) ;
#27456=EDGE_CURVE ( 'NONE', #24582, #7335, #12647, .T. ) ;
#27458=CARTESIAN_POINT ( 'NONE',  ( 74.59884440882045453, 36.53515624999999289, 9.598844408820456309 ) ) ;
#27464=CARTESIAN_POINT ( 'NONE',  ( 124.5550856135277087, 39.31328125108394289, 13.14518615778179722 ) ) ;
#27465=CARTESIAN_POINT ( 'NONE',  ( 65.00000000000000000, 35.98945312608393010, 13.14518615778179544 ) ) ;
#27467=CARTESIAN_POINT ( 'NONE',  ( 13.14518615778179544, 36.18789062608393436, -1.609821015232357215E-15 ) ) ;
#27471=ADVANCED_FACE ( 'NONE', ( #21373 ), #12786, .T. ) ;
#27472=DIRECTION ( 'NONE',  ( -0.000000000000000000, 1.000000000000000000, -0.000000000000000000 ) ) ;
#27474=CARTESIAN_POINT ( 'NONE',  ( 104.9999999999999716, 82.56250000273119838, 2.071067811865462627 ) ) ;
#27478=B_SPLINE_CURVE_WITH_KNOTS ( 'NONE', 3,
 ( #12596, #10467, #19175, #6210, #25312, #23322, #27878, #12042, #8339, #17024, #5802, #12455, #21180, #25727, #9913, #18629, #7792, #16478, #25174, #22023, #8621, #19734, #21463, #6618, #218 ),
 .UNSPECIFIED., .F., .F.,
 ( 4, 2, 2, 2, 2, 2, 2, 1, 2, 2, 2, 2, 4 ),
 ( 0.000000000000000000, 0.001301161269048799847, 0.002602322538097599693, 0.005204645076195206325, 0.007806967614292812524, 0.01040929015239041959, 0.01171045142143921532, 0.01301161269048801104, 0.01431277395953680504, 0.01561393522858560076, 0.01821625776668319222, 0.01951741903573200876, 0.02081858030478082183 ),
 .UNSPECIFIED. ) ;
#27479=CARTESIAN_POINT ( 'NONE',  ( 133.0892609137966360, 35.99999999999997158, -13.21136010216379297 ) ) ;
#27485=DIRECTION ( 'NONE',  ( 0.000000000000000000, 0.000000000000000000, 1.000000000000000000 ) ) ;
#27490=CARTESIAN_POINT ( 'NONE',  ( 96.84719886470459471, 81.56250000136559208, 3.152801135295355994 ) ) ;
#27491=CARTESIAN_POINT ( 'NONE',  ( 74.29505027212704249, 39.66054687608393436, -9.295050272127046043 ) ) ;
#27497=CARTESIAN_POINT ( 'NONE',  ( 130.0000000000000000, 33.40976562608393863, -13.14518615778179544 ) ) ;
#27499=CARTESIAN_POINT ( 'NONE',  ( -3.797451868958014565, 54.08938259242987812, -15.00000000000000178 ) ) ;
#27500=CARTESIAN_POINT ( 'NONE',  ( 195.0000000000000000, -7.395377635281828788, -2.255140518769849538E-14 ) ) ;
#27502=CARTESIAN_POINT ( 'NONE',  ( 124.5550856135277087, 38.32109375108394289, 13.14518615778179722 ) ) ;
#27503=CARTESIAN_POINT ( 'NONE',  ( 70.62287287157786864, 36.88242187716787157, -13.57481594606304753 ) ) ;
#27505=CARTESIAN_POINT ( 'NONE',  ( 9.598844408820459861, 39.01562500216787299, 9.598844408820456309 ) ) ;
#27506=ORIENTED_EDGE ( 'NONE', *, *, #24474, .T. ) ;
#27510=CARTESIAN_POINT ( 'NONE',  ( 200.6228728715778686, 31.82226562716787654, 13.57481594606304576 ) ) ;
#27512=CARTESIAN_POINT ( 'NONE',  ( 143.1451861577818079, 36.98164062608393010, -1.609821015232357215E-15 ) ) ;
#27515=( BOUNDED_CURVE ( )  B_SPLINE_CURVE ( 2, ( #19059, #27767, #12625, #8225, #1831, #27360, #16915, #23484, #5690 ),
 .UNSPECIFIED., .F., .F. ) 
 B_SPLINE_CURVE_WITH_KNOTS ( ( 3, 2, 2, 2, 3 ),
 ( 0.1875000000000001388, 0.1979166666666667407, 0.2083333333333333703, 0.2187499999999999722, 0.2291666666666665741 ),
 .UNSPECIFIED. ) 
 CURVE ( )  GEOMETRIC_REPRESENTATION_ITEM ( )  RATIONAL_B_SPLINE_CURVE ( ( 0.9999999999999990008, 0.9238795325112877377, 1.000000000000000000, 0.9238795325112867385, 1.000000000000000000, 0.9238795325112867385, 1.000000000000000000, 0.9238795325112872936, 0.9999999999999994449 ) ) 
 REPRESENTATION_ITEM ( '' )  );
#27519=CARTESIAN_POINT ( 'NONE',  ( 204.5988444088204403, 39.11484374999999858, -9.598844408820458085 ) ) ;
#27529=CARTESIAN_POINT ( 'NONE',  ( 13.57481594606304753, 39.85898437499999858, -5.622872871577873077 ) ) ;
#27530=EDGE_LOOP ( 'NONE', ( #4423, #22430, #15590, #1159 ) ) ;
#27531=CARTESIAN_POINT ( 'NONE',  ( 104.4587341249999639, 81.18750000136559208, -1.442382525525748735E-14 ) ) ;
#27532=CIRCLE ( 'NONE', #13843, 11.57481594606304398 ) ;
#27535=VERTEX_POINT ( 'NONE', #8948 ) ;
#27536=CARTESIAN_POINT ( 'NONE',  ( 186.2451010467579522, 50.00000000000000000, -10.39041163856320793 ) ) ;
#27541=CARTESIAN_POINT ( 'NONE',  ( 200.6228728715778686, 39.75976562716787299, 13.57481594606304576 ) ) ;
#27544=CARTESIAN_POINT ( 'NONE',  ( 124.5550856135277087, 38.22187500108393721, -13.14518615778179722 ) ) ;
#27545=CARTESIAN_POINT ( 'NONE',  ( -13.14518615778179900, 39.90859375108394147, -5.444914386472297529 ) ) ;
#27546=AXIS2_PLACEMENT_3D ( 'NONE', #16864, #27165, #1223 ) ;
#27548=CARTESIAN_POINT ( 'NONE',  ( 74.59884440882045453, 38.91640624999999432, 9.598844408820456309 ) ) ;
#27549=CARTESIAN_POINT ( 'NONE',  ( 51.42518405393695957, 39.56132812716787583, 5.622872871577880183 ) ) ;
#27550=DIRECTION ( 'NONE',  ( 0.000000000000000000, 0.000000000000000000, -1.000000000000000000 ) ) ;
#27554=CARTESIAN_POINT ( 'NONE',  ( 104.4587341249999781, 81.25000000136559208, -1.846868145590750521 ) ) ;
#27563=EDGE_CURVE ( 'NONE', #12843, #25242, #17639, .T. ) ;
#27564=VECTOR ( 'NONE', #25506, 1000.000000000000000 ) ;
#27567=CARTESIAN_POINT ( 'NONE',  ( 51.85481384221820633, 39.11484375108393863, -5.444914386472297529 ) ) ;
#27572=CARTESIAN_POINT ( 'NONE',  ( -2.024627725537266443, 50.00000000051014126, -13.43320860980949227 ) ) ;
#27573=VECTOR ( 'NONE', #334, 1000.000000000000000 ) ;
#27574=CARTESIAN_POINT ( 'NONE',  ( 69.15728635496172672, 36.00000000000000000, -12.92256159328856135 ) ) ;
#27576=CARTESIAN_POINT ( 'NONE',  ( 143.5748159460630404, 33.60820312716787583, -5.622872871577873077 ) ) ;
#27577=CARTESIAN_POINT ( 'NONE',  ( 65.00000000000000000, 40.10703125216787157, -13.57481594606304576 ) ) ;
#27579=CARTESIAN_POINT ( 'NONE',  ( 185.7049497278729575, 38.27148437608393294, -9.295050272127046043 ) ) ;
#27584=CARTESIAN_POINT ( 'NONE',  ( 9.598844408820459861, 38.12265624999999858, 9.598844408820456309 ) ) ;
#27585=CARTESIAN_POINT ( 'NONE',  ( 74.59884440882045453, 39.80937500216786873, 9.598844408820456309 ) ) ;
#27588=AXIS2_PLACEMENT_3D ( 'NONE', #12032, #27867, #8327 ) ;
#27596=CARTESIAN_POINT ( 'NONE',  ( 116.8548138422182063, 38.42031250108393436, 5.444914386472304635 ) ) ;
#27598=CARTESIAN_POINT ( 'NONE',  ( 70.44491438647230552, 35.54296875108393294, -13.14518615778179900 ) ) ;
#27601=CARTESIAN_POINT ( 'NONE',  ( -9.295050272127046043, 34.10429687608393579, -9.295050272127046043 ) ) ;
#27602=CARTESIAN_POINT ( 'NONE',  ( 191.5797791878283647, 36.00000000000000711, -13.02105590829173565 ) ) ;
#27606=CARTESIAN_POINT ( 'NONE',  ( 116.4251840539369738, 40.25585937499999289, 5.622872871577880183 ) ) ;
#27608=DIRECTION ( 'NONE',  ( -0.000000000000000000, -1.000000000000000000, -0.000000000000000000 ) ) ;
#27609=CARTESIAN_POINT ( 'NONE',  ( 9.295050272127047819, 40.05742187608392868, 9.295050272127046043 ) ) ;
#27613=EDGE_CURVE ( 'NONE', #3340, #1089, #16794, .T. ) ;
#27616=CARTESIAN_POINT ( 'NONE',  ( 181.4251840539369596, 39.46210937716787726, -5.622872871577872189 ) ) ;
#27624=CARTESIAN_POINT ( 'NONE',  ( 195.0000000000000000, 36.53515625216787299, 13.57481594606304576 ) ) ;
#27625=CARTESIAN_POINT ( 'NONE',  ( 95.54126587499995082, 81.37500000136563472, -1.846868145590750077 ) ) ;
#27626=CARTESIAN_POINT ( 'NONE',  ( 70.44491438647230552, 37.03125000108393294, 13.14518615778179189 ) ) ;
#27631=CARTESIAN_POINT ( 'NONE',  ( 124.3771271284221314, 39.56132812499999574, 13.57481594606304753 ) ) ;
#27636=CARTESIAN_POINT ( 'NONE',  ( 95.54126587499996504, 80.43750000136559208, -1.387778780781445676E-14 ) ) ;
#27637=CARTESIAN_POINT ( 'NONE',  ( 135.4449143864723055, 39.21406250108392300, 13.14518615778179189 ) ) ;
#27638=CARTESIAN_POINT ( 'NONE',  ( 65.00000000000000000, 35.74140625216787015, 13.57481594606304576 ) ) ;
#27640=CARTESIAN_POINT ( 'NONE',  ( 2.493653234604083739E-15, 37.32890625216786873, 13.57481594606304576 ) ) ;
#27641=ORIENTED_EDGE ( 'NONE', *, *, #23271, .T. ) ;
#27646=CARTESIAN_POINT ( 'NONE',  ( 185.7049497278729575, 36.48554687608393721, -9.295050272127046043 ) ) ;
#27649=CARTESIAN_POINT ( 'NONE',  ( 116.8548138422182205, 38.12265625108393863, -5.444914386472297529 ) ) ;
#27651=DIRECTION ( 'NONE',  ( 0.000000000000000000, 0.000000000000000000, 1.000000000000000000 ) ) ;
#27655=CARTESIAN_POINT ( 'NONE',  ( 195.0000000000000000, 39.21406249999999716, -13.57481594606304576 ) ) ;
#27658=CARTESIAN_POINT ( 'NONE',  ( 65.00000000000000000, 39.56132812608393579, -13.14518615778179544 ) ) ;
#27663=CARTESIAN_POINT ( 'NONE',  ( 9.598844408820456309, 39.90859374999999432, -9.598844408820458085 ) ) ;
#27664=CARTESIAN_POINT ( 'NONE',  ( 120.7049497278729575, 40.65273437608393436, -9.295050272127046043 ) ) ;
#27666=CARTESIAN_POINT ( 'NONE',  ( 95.54126587499995082, 83.62500000136560629, -1.846868145590750077 ) ) ;
#27667=AXIS2_PLACEMENT_3D ( 'NONE', #1668, #7928, #6215 ) ;
#27669=EDGE_LOOP ( 'NONE', ( #8305, #19761 ) ) ;
#27670=ORIENTED_EDGE ( 'NONE', *, *, #2382, .F. ) ;
#27671=CARTESIAN_POINT ( 'NONE',  ( 131.6052718765765803, 53.60388944777321996, -15.00000000000000355 ) ) ;
#27672=EDGE_CURVE ( 'NONE', #9425, #21442, #1336, .T. ) ;
#27674=ORIENTED_EDGE ( 'NONE', *, *, #15225, .F. ) ;
#27678=CARTESIAN_POINT ( 'NONE',  ( 181.4251840539369596, 38.66835937716786731, -5.622872871577873077 ) ) ;
#27682=CARTESIAN_POINT ( 'NONE',  ( 116.8548138422182205, 39.11484375108393863, -5.444914386472297529 ) ) ;
#27683=CARTESIAN_POINT ( 'NONE',  ( -13.14518615778179544, 33.40976562608393863, 0.000000000000000000 ) ) ;
#27684=ORIENTED_EDGE ( 'NONE', *, *, #22737, .F. ) ;
#27685=CARTESIAN_POINT ( 'NONE',  ( 65.00000000000000000, 39.21406249999999716, -13.57481594606304576 ) ) ;
#27686=DIRECTION ( 'NONE',  ( 0.000000000000000000, -1.000000000000000000, 0.000000000000000000 ) ) ;
#27688=CARTESIAN_POINT ( 'NONE',  ( 204.4320061696341497, 36.00000000000001421, 9.391769196590237456 ) ) ;
#27693=CARTESIAN_POINT ( 'NONE',  ( 103.1528011352953342, 83.06250000136560629, 3.152801135295355106 ) ) ;
#27695=CARTESIAN_POINT ( 'NONE',  ( -13.14518615778179544, 40.75195312608393294, 0.000000000000000000 ) ) ;
#27697=ORIENTED_EDGE ( 'NONE', *, *, #9846, .F. ) ;
#27698=DIRECTION ( 'NONE',  ( 0.000000000000000000, 1.000000000000000000, 0.000000000000000000 ) ) ;
#27701=CARTESIAN_POINT ( 'NONE',  ( 181.9040934463640156, 35.99999999999999289, 1.137167824541468031 ) ) ;
#27705=CARTESIAN_POINT ( 'NONE',  ( 59.55508561352770158, 37.72578125108394431, 13.14518615778179722 ) ) ;
#27706=CARTESIAN_POINT ( 'NONE',  ( 97.92893218813449607, 83.31250000273118417, 4.999999999999981348 ) ) ;
#27708=CARTESIAN_POINT ( 'NONE',  ( 200.4449143864723055, 32.26875000108393721, 13.14518615778179189 ) ) ;
#27711=CARTESIAN_POINT ( 'NONE',  ( 120.4011555911795455, 37.92421874999999432, 9.598844408820459861 ) ) ;
#27712=CIRCLE ( 'NONE', #24080, 5.000000000000000888 ) ;
#27713=CARTESIAN_POINT ( 'NONE',  ( 139.5988444088204687, 36.63437500216787157, 9.598844408820456309 ) ) ;
#27715=CARTESIAN_POINT ( 'NONE',  ( 139.5988444088204403, 36.03906250216787299, -9.598844408820458085 ) ) ;
#27717=CARTESIAN_POINT ( 'NONE',  ( 55.70494972787295751, 39.26367187608393294, 9.295050272127047819 ) ) ;
#27719=CARTESIAN_POINT ( 'NONE',  ( 204.2950502721270425, 38.86679687608393863, -9.295050272127046043 ) ) ;
#27720=ORIENTED_EDGE ( 'NONE', *, *, #21918, .F. ) ;
#27722=ORIENTED_EDGE ( 'NONE', *, *, #3446, .F. ) ;
#27730=CARTESIAN_POINT ( 'NONE',  ( 6.106658654947462850, 36.00000000000003553, 11.74215035806574647 ) ) ;
#27732=CARTESIAN_POINT ( 'NONE',  ( 143.5748159460630688, 32.66562499999999858, -1.662435489736055892E-15 ) ) ;
#27733=VERTEX_POINT ( 'NONE', #26636 ) ;
#27737=CARTESIAN_POINT ( 'NONE',  ( 139.2950502721270425, 40.25585937608393294, 9.295050272127046043 ) ) ;
#27738=CARTESIAN_POINT ( 'NONE',  ( 59.55508561352770158, 38.32109375108394289, 13.14518615778179722 ) ) ;
#27739=CARTESIAN_POINT ( 'NONE',  ( 181.8548138422182205, 32.61601562608393579, 0.000000000000000000 ) ) ;
#27740=DIRECTION ( 'NONE',  ( 0.000000000000000000, -0.000000000000000000, 1.000000000000000000 ) ) ;
#27741=CARTESIAN_POINT ( 'NONE',  ( -8.049105076161786076E-16, 34.00507812608393721, -13.14518615778179544 ) ) ;
#27743=FACE_OUTER_BOUND ( 'NONE', #21462, .T. ) ;
#27747=CARTESIAN_POINT ( 'NONE',  ( 2.414731522848535132E-15, 38.37070312608393152, 13.14518615778179544 ) ) ;
#27748=CARTESIAN_POINT ( 'NONE',  ( -3.865414375413190218, 54.10683252460146520, 14.99999999999999289 ) ) ;
#27754=ORIENTED_EDGE ( 'NONE', *, *, #17170, .T. ) ;
#27760=CARTESIAN_POINT ( 'NONE',  ( 195.0000000000000000, 36.13828125216787157, -13.57481594606304576 ) ) ;
#27761=CARTESIAN_POINT ( 'NONE',  ( 98.15313185440925281, 79.62500000136560629, 4.458734124999987891 ) ) ;
#27762=CARTESIAN_POINT ( 'NONE',  ( 70.44491438647230552, 38.61875000108393152, 13.14518615778179189 ) ) ;
#27767=CARTESIAN_POINT ( 'NONE',  ( 135.6228728715779255, 39.16445312500000142, -13.57481594606299247 ) ) ;
#27769=CARTESIAN_POINT ( 'NONE',  ( 124.5550856135277087, 32.16953125108393152, 13.14518615778179722 ) ) ;
#27770=ORIENTED_EDGE ( 'NONE', *, *, #10559, .F. ) ;
#27773=CARTESIAN_POINT ( 'NONE',  ( 103.1528011352953342, 81.06250000136559208, -3.152801135295383084 ) ) ;
#27775=CARTESIAN_POINT ( 'NONE',  ( 74.59884440882045453, 36.63437500216787157, 9.598844408820456309 ) ) ;
#27777=CARTESIAN_POINT ( 'NONE',  ( -9.598844408820458085, 35.44375000216787441, -9.598844408820458085 ) ) ;
#27778=ORIENTED_EDGE ( 'NONE', *, *, #17150, .T. ) ;
#27780=CARTESIAN_POINT ( 'NONE',  ( 0.000000000000000000, 50.00000000000000000, 0.000000000000000000 ) ) ;
#27782=CARTESIAN_POINT ( 'NONE',  ( 208.1451861577818079, 36.18789062608393436, -1.609821015232357215E-15 ) ) ;
#27784=CARTESIAN_POINT ( 'NONE',  ( 143.1451861577818363, 39.31328125108392868, 5.444914386472293977 ) ) ;
#27785=EDGE_CURVE ( 'NONE', #28009, #439, #19043, .T. ) ;
#27786=DIRECTION ( 'NONE',  ( -0.000000000000000000, -1.000000000000000000, -0.000000000000000000 ) ) ;
#27787=CARTESIAN_POINT ( 'NONE',  ( 135.6228728715779539, 37.27929687499999289, 13.57481594606297115 ) ) ;
#27793=CARTESIAN_POINT ( 'NONE',  ( 181.4251840539369596, 38.56914062500000284, -5.622872871577873077 ) ) ;
#27795=CYLINDRICAL_SURFACE ( 'NONE', #15963, 5.000000000000004441 ) ;
#27797=CARTESIAN_POINT ( 'NONE',  ( 65.00000000000000000, 37.97382812608393721, -13.14518615778179544 ) ) ;
#27803=CARTESIAN_POINT ( 'NONE',  ( 2.493653234604083739E-15, 40.40468749999999432, 13.57481594606304576 ) ) ;
#27807=CARTESIAN_POINT ( 'NONE',  ( 101.8468681455906903, 82.37500000136562051, -4.458734125000016313 ) ) ;
#27809=VERTEX_POINT ( 'NONE', #26780 ) ;
#27810=EDGE_CURVE ( 'NONE', #2928, #2045, #18962, .T. ) ;
#27812=CARTESIAN_POINT ( 'NONE',  ( 70.44491438647230552, 34.15390625108393863, -13.14518615778179900 ) ) ;
#27814=CARTESIAN_POINT ( 'NONE',  ( 123.9209199794811980, 54.65154858643462177, -15.00000000000000178 ) ) ;
#27815=AXIS2_PLACEMENT_3D ( 'NONE', #20208, #15344, #2409 ) ;
#27820=CARTESIAN_POINT ( 'NONE',  ( 195.0000000000000000, 38.12265625216787157, 13.57481594606304576 ) ) ;
#27822=DIRECTION ( 'NONE',  ( -0.000000000000000000, 1.000000000000000000, -0.000000000000000000 ) ) ;
#27823=CARTESIAN_POINT ( 'NONE',  ( 198.9798144458085858, 50.00000000123236532, 13.01613927312799390 ) ) ;
#27824=CARTESIAN_POINT ( 'NONE',  ( 124.5550856135277087, 39.80937500108393579, -13.14518615778179722 ) ) ;
#27825=CARTESIAN_POINT ( 'NONE',  ( 2.414731522848535132E-15, 39.36289062608393152, 13.14518615778179544 ) ) ;
#27827=ORIENTED_EDGE ( 'NONE', *, *, #19570, .F. ) ;
#27828=CARTESIAN_POINT ( 'NONE',  ( 70.62287287157786864, 37.57695312499998863, -13.57481594606304753 ) ) ;
#27829=CARTESIAN_POINT ( 'NONE',  ( 9.598844408820459861, 38.22187500216787015, 9.598844408820456309 ) ) ;
#27830=CARTESIAN_POINT ( 'NONE',  ( 201.3519322287720854, 36.00000000000000711, 11.61660627739470186 ) ) ;
#27834=CARTESIAN_POINT ( 'NONE',  ( 95.54126587499996504, 83.62500000136560629, -1.846868145590750077 ) ) ;
#27836=CARTESIAN_POINT ( 'NONE',  ( -13.14518615778179189, 39.21406250108392300, 5.444914386472304635 ) ) ;
#27837=ADVANCED_FACE ( 'NONE', ( #23200 ), #5675, .T. ) ;
#27840=CARTESIAN_POINT ( 'NONE',  ( -13.57481594606304576, 40.65273437608393436, 0.000000000000000000 ) ) ;
#27842=CARTESIAN_POINT ( 'NONE',  ( 96.46446609406721961, 81.25000000273119838, 3.535533905932727539 ) ) ;
#27845=ORIENTED_EDGE ( 'NONE', *, *, #15166, .T. ) ;
#27846=CARTESIAN_POINT ( 'NONE',  ( 78.14518615778179367, 37.97382812608393721, -1.609821015232357215E-15 ) ) ;
#27847=DIRECTION ( 'NONE',  ( -0.000000000000000000, 1.000000000000000000, -0.000000000000000000 ) ) ;
#27849=EDGE_LOOP ( 'NONE', ( #20054, #9213, #17004 ) ) ;
#27853=CARTESIAN_POINT ( 'NONE',  ( 135.6228728715778971, 34.99726562716787726, 13.57481594606304576 ) ) ;
#27854=CARTESIAN_POINT ( 'NONE',  ( 70.44491438647230552, 40.20625000108394431, 13.14518615778179189 ) ) ;
#27855=CARTESIAN_POINT ( 'NONE',  ( 208.1451861577817795, 35.54296875108394715, 5.444914386472293977 ) ) ;
#27856=ORIENTED_EDGE ( 'NONE', *, *, #17865, .F. ) ;
#27861=DIRECTION ( 'NONE',  ( 0.000000000000000000, 3.469446951953611231E-16, -1.000000000000000000 ) ) ;
#27863=CARTESIAN_POINT ( 'NONE',  ( 104.4587341249999781, 83.87500000136560629, 1.846868145590721655 ) ) ;
#27865=CARTESIAN_POINT ( 'NONE',  ( 143.5748159460630688, 39.95820312716787726, -5.622872871577873966 ) ) ;
#27867=DIRECTION ( 'NONE',  ( -0.000000000000000000, 1.000000000000000000, 0.000000000000000000 ) ) ;
#27874=CARTESIAN_POINT ( 'NONE',  ( 120.7049497278729575, 36.88242187608393152, 9.295050272127047819 ) ) ;
#27875=CARTESIAN_POINT ( 'NONE',  ( 51.85481384221820633, 37.37851562608393863, 0.000000000000000000 ) ) ;
#27876=CARTESIAN_POINT ( 'NONE',  ( 185.7049497278729575, 31.92148437608393508, 9.295050272127047819 ) ) ;
#27878=CARTESIAN_POINT ( 'NONE',  ( 52.94344797029973648, 36.00000000000000000, 5.307619621752120764 ) ) ;
#27879=CARTESIAN_POINT ( 'NONE',  ( 5.444914386472297529, 35.54296875108393294, -13.14518615778179900 ) ) ;
#27880=CARTESIAN_POINT ( 'NONE',  ( 125.4951129136839825, 51.44650206076906329, -15.00000000000066258 ) ) ;
#27882=CARTESIAN_POINT ( 'NONE',  ( 96.46446609406721961, 81.87500000000000000, -3.535533905932755072 ) ) ;
#27883=CARTESIAN_POINT ( 'NONE',  ( 5.444914386472297529, 38.71796875108393721, -13.14518615778179900 ) ) ;
#27892=ORIENTED_EDGE ( 'NONE', *, *, #1010, .T. ) ;
#27896=AXIS2_PLACEMENT_3D ( 'NONE', #16166, #22883, #14581 ) ;
#27899=CARTESIAN_POINT ( 'NONE',  ( 98.15313185440925281, 80.25000000136559208, -4.458734125000016313 ) ) ;
#27900=CARTESIAN_POINT ( 'NONE',  ( 65.00000000000000000, 38.56914062608393579, 13.14518615778179544 ) ) ;
#27904=DIRECTION ( 'NONE',  ( -0.000000000000000000, 1.000000000000000000, -0.000000000000000000 ) ) ;
#27906=CARTESIAN_POINT ( 'NONE',  ( 124.3771271284221314, 40.85117187499999147, -13.57481594606304753 ) ) ;
#27908=CYLINDRICAL_SURFACE ( 'NONE', #22237, 13.57481594606304398 ) ;
#27910=CARTESIAN_POINT ( 'NONE',  ( 104.4587341249999781, 81.00000000136560629, -1.846868145590750299 ) ) ;
#27911=CARTESIAN_POINT ( 'NONE',  ( 143.1451861577818079, 39.41250000108393436, -5.444914386472297529 ) ) ;
#27912=CARTESIAN_POINT ( 'NONE',  ( 59.37712712842213136, 38.07304687716787583, 13.57481594606304753 ) ) ;
#27913=EDGE_CURVE ( 'NONE', #22062, #15169, #24981, .T. ) ;
#27915=CARTESIAN_POINT ( 'NONE',  ( 5.622872871577871301, 34.50117187716788436, -13.57481594606304753 ) ) ;
#27916=ORIENTED_EDGE ( 'NONE', *, *, #26236, .T. ) ;
#27919=( BOUNDED_CURVE ( )  B_SPLINE_CURVE ( 2, ( #13379, #22108, #2587, #22532, #15817, #22388, #9552, #20816, #3288 ),
 .UNSPECIFIED., .F., .T. ) 
 B_SPLINE_CURVE_WITH_KNOTS ( ( 3, 2, 2, 2, 3 ),
 ( 0.1875000000000001388, 0.1979166666666667407, 0.2083333333333333703, 0.2187499999999999722, 0.2291666666666665741 ),
 .UNSPECIFIED. ) 
 CURVE ( )  GEOMETRIC_REPRESENTATION_ITEM ( )  RATIONAL_B_SPLINE_CURVE ( ( 0.9999999999999990008, 0.9238795325112877377, 1.000000000000000000, 0.9238795325112867385, 1.000000000000000000, 0.9238795325112867385, 1.000000000000000000, 0.9238795325112872936, 0.9999999999999994449 ) ) 
 REPRESENTATION_ITEM ( '' )  );
#27920=CARTESIAN_POINT ( 'NONE',  ( 200.4449143864723055, 37.92421875108392726, -13.14518615778179900 ) ) ;
#27922=CARTESIAN_POINT ( 'NONE',  ( 130.0000000000000000, 38.37070312608393152, 13.14518615778179544 ) ) ;
#27924=CARTESIAN_POINT ( 'NONE',  ( 219.9999999999999716, 75.00000000000000000, 14.99999999999994316 ) ) ;
#27926=FACE_OUTER_BOUND ( 'NONE', #1461, .T. ) ;
#27928=CARTESIAN_POINT ( 'NONE',  ( 185.4011555911795597, 37.13046874999999147, 9.598844408820459861 ) ) ;
#27932=CARTESIAN_POINT ( 'NONE',  ( 51.85481384221819923, 38.91640625108393436, -5.444914386472297529 ) ) ;
#27936=CARTESIAN_POINT ( 'NONE',  ( 120.4011555911795455, 39.51171874999999289, 9.598844408820459861 ) ) ;
#27937=CARTESIAN_POINT ( 'NONE',  ( -13.57481594606304753, 39.36289062499999858, -5.622872871577873077 ) ) ;
#27938=CARTESIAN_POINT ( 'NONE',  ( 120.7049497278729575, 40.05742187608393579, 9.295050272127047819 ) ) ;
#27939=ORIENTED_EDGE ( 'NONE', *, *, #16296, .T. ) ;
#27940=CARTESIAN_POINT ( 'NONE',  ( 99.99999999999995737, 82.43750000136559208, -4.458734125000016313 ) ) ;
#27941=EDGE_CURVE ( 'NONE', #15622, #16261, #25053, .T. ) ;
#27942=LINE ( 'NONE', #16687, #22047 ) ;
#27943=ORIENTED_EDGE ( 'NONE', *, *, #16579, .F. ) ;
#27945=CARTESIAN_POINT ( 'NONE',  ( 74.29505027212704249, 33.90585937608393863, 9.295050272127046043 ) ) ;
#27946=ORIENTED_EDGE ( 'NONE', *, *, #27613, .F. ) ;
#27948=CARTESIAN_POINT ( 'NONE',  ( -13.57481594606304753, 36.98164062499999005, -5.622872871577872189 ) ) ;
#27952=CARTESIAN_POINT ( 'NONE',  ( 94.99999999999995737, 82.06250000273119838, -2.071067811865491493 ) ) ;
#27954=CARTESIAN_POINT ( 'NONE',  ( 195.0000000000000000, 38.91640625216786731, 13.57481594606304576 ) ) ;
#27957=CARTESIAN_POINT ( 'NONE',  ( 199.8584992904752937, 49.99999999891486624, 12.70434618648238256 ) ) ;
#27958=CARTESIAN_POINT ( 'NONE',  ( -12.68159279706118170, 36.04503594658365984, 5.908507747192915716 ) ) ;
#27959=CARTESIAN_POINT ( 'NONE',  ( 13.14518615778179900, 38.81718750108393579, -5.444914386472297529 ) ) ;
#27960=ORIENTED_EDGE ( 'NONE', *, *, #19455, .F. ) ;
#27961=CARTESIAN_POINT ( 'NONE',  ( 116.8548138422182063, 35.74140625108393721, -5.444914386472297529 ) ) ;
#27962=CARTESIAN_POINT ( 'NONE',  ( 51.42518405393695957, 37.82499999999999574, 0.000000000000000000 ) ) ;
#27963=CARTESIAN_POINT ( 'NONE',  ( 65.00000000000000000, 39.31328125216787583, -13.57481594606304576 ) ) ;
#27966=CARTESIAN_POINT ( 'NONE',  ( 96.46446609406721961, 84.00000000273119838, -3.535533905932755072 ) ) ;
#27972=CARTESIAN_POINT ( 'NONE',  ( 13.14518615778179544, 39.56132812608393579, -1.609821015232357215E-15 ) ) ;
#27974=ORIENTED_EDGE ( 'NONE', *, *, #9118, .F. ) ;
#27980=EDGE_CURVE ( 'NONE', #6018, #10602, #12338, .T. ) ;
#27981=CARTESIAN_POINT ( 'NONE',  ( 181.8548138422182205, 38.96601562608393721, 0.000000000000000000 ) ) ;
#27982=VERTEX_POINT ( 'NONE', #19042 ) ;
#27983=CARTESIAN_POINT ( 'NONE',  ( 130.0000000000000000, 36.13828125216787157, -13.57481594606304576 ) ) ;
#27991=EDGE_CURVE ( 'NONE', #22131, #18157, #21893, .T. ) ;
#27992=CARTESIAN_POINT ( 'NONE',  ( 139.5988444088204687, 35.04687500216787299, 9.598844408820456309 ) ) ;
#27993=CARTESIAN_POINT ( 'NONE',  ( 74.29505027212704249, 40.45429687608393721, -9.295050272127046043 ) ) ;
#27994=CARTESIAN_POINT ( 'NONE',  ( 99.99999999999995737, 84.25000000000000000, 4.999999999999990230 ) ) ;
#27995=CARTESIAN_POINT ( 'NONE',  ( 204.2950502721270425, 34.10429687608393579, -9.295050272127046043 ) ) ;
#27996=ORIENTED_EDGE ( 'NONE', *, *, #16960, .F. ) ;
#27997=ORIENTED_EDGE ( 'NONE', *, *, #25674, .T. ) ;
#27999=CARTESIAN_POINT ( 'NONE',  ( 94.99999999999995737, 84.00000000000000000, -1.387778780781445676E-14 ) ) ;
#28001=CARTESIAN_POINT ( 'NONE',  ( 101.8468681455907046, 82.75000000136560629, 4.458734124999987891 ) ) ;
#28002=CARTESIAN_POINT ( 'NONE',  ( 70.62287287157796811, 40.05742187716787583, -13.57481594606294095 ) ) ;
#28005=AXIS2_PLACEMENT_3D ( 'NONE', #9237, #8810, #2829 ) ;
#28009=VERTEX_POINT ( 'NONE', #10062 ) ;
#28014=CARTESIAN_POINT ( 'NONE',  ( 116.8548138422182063, 36.73359375108393010, -5.444914386472297529 ) ) ;
#28015=CARTESIAN_POINT ( 'NONE',  ( 78.14518615778179367, 36.13828125108393863, 5.444914386472293977 ) ) ;
#28016=CARTESIAN_POINT ( 'NONE',  ( 181.8548138422182205, 39.95820312608393010, 0.000000000000000000 ) ) ;
#28018=CARTESIAN_POINT ( 'NONE',  ( 13.14518615778179900, 36.23750000108393010, -5.444914386472297529 ) ) ;
#28019=CARTESIAN_POINT ( 'NONE',  ( 139.1801758136479918, 55.00000000000000000, -15.00000000000000000 ) ) ;
#28023=CARTESIAN_POINT ( 'NONE',  ( 13.14518615778179900, 39.41250000108393436, -5.444914386472297529 ) ) ;
#28026=CARTESIAN_POINT ( 'NONE',  ( 63.05267407791385637, 51.47162402671693116, 15.00000000000195399 ) ) ;
#28030=CARTESIAN_POINT ( 'NONE',  ( 78.45411265623080510, 36.00000000000001421, 0.6772748633563907550 ) ) ;
#28031=VERTEX_POINT ( 'NONE', #5812 ) ;
#28032=CARTESIAN_POINT ( 'NONE',  ( 9.180175813647995398, 55.00000000000000000, 9.999999999999994671 ) ) ;
#28035=DIRECTION ( 'NONE',  ( -0.000000000000000000, -1.000000000000000000, -0.000000000000000000 ) ) ;
#28036=CARTESIAN_POINT ( 'NONE',  ( 96.84719886470459471, 80.56250000136559208, -3.152801135295383084 ) ) ;
#28037=CARTESIAN_POINT ( 'NONE',  ( 55.70494972787295751, 37.47773437608393010, -9.295050272127046043 ) ) ;
#28039=CARTESIAN_POINT ( 'NONE',  ( -13.14518615778179189, 39.80937500108393579, 5.444914386472304635 ) ) ;
#28040=( BOUNDED_CURVE ( )  B_SPLINE_CURVE ( 2, ( #3841, #10374, #25225, #14649, #20683, #23096, #23368, #27787, #8111 ),
 .UNSPECIFIED., .F., .F. ) 
 B_SPLINE_CURVE_WITH_KNOTS ( ( 3, 2, 2, 2, 3 ),
 ( 0.3541666666666666852, 0.3645833333333332593, 0.3749999999999998890, 0.3854166666666665741, 0.3958333333333331483 ),
 .UNSPECIFIED. ) 
 CURVE ( )  GEOMETRIC_REPRESENTATION_ITEM ( )  RATIONAL_B_SPLINE_CURVE ( ( 1.000000000000000000, 0.9238795325112867385, 1.000000000000000000, 0.9238795325112867385, 1.000000000000000000, 0.9238795325112867385, 1.000000000000000000, 0.9238795325112879597, 0.9999999999999987788 ) ) 
 REPRESENTATION_ITEM ( '' )  );
#28041=VERTEX_POINT ( 'NONE', #18905 ) ;
#28045=CARTESIAN_POINT ( 'NONE',  ( 143.5748159460630404, 40.65273437499998721, -5.622872871577873077 ) ) ;
#28046=ORIENTED_EDGE ( 'NONE', *, *, #13761, .F. ) ;
#28049=CARTESIAN_POINT ( 'NONE',  ( 96.84719886470459471, 80.56250000136559208, 3.152801135295355994 ) ) ;
#28050=CARTESIAN_POINT ( 'NONE',  ( 139.2950502721270425, 36.28710937608393294, -9.295050272127046043 ) ) ;
#28051=CARTESIAN_POINT ( 'NONE',  ( 51.42518405393695957, 36.33671875216787583, 0.000000000000000000 ) ) ;
#28053=CARTESIAN_POINT ( 'NONE',  ( 13.57481594606304931, 36.68398437716788152, 5.622872871577869525 ) ) ;
#28054=AXIS2_PLACEMENT_3D ( 'NONE', #19444, #15290, #24007 ) ;
#28057=CARTESIAN_POINT ( 'NONE',  ( 181.8548138422181921, 38.22187500108393010, 5.444914386472304635 ) ) ;
#28059=ORIENTED_EDGE ( 'NONE', *, *, #24347, .F. ) ;
#28060=DIRECTION ( 'NONE',  ( 1.156482317317871478E-16, 0.000000000000000000, 1.000000000000000000 ) ) ;
#28062=DIRECTION ( 'NONE',  ( 0.000000000000000000, -1.000000000000000000, 0.000000000000000000 ) ) ;
#28063=CARTESIAN_POINT ( 'NONE',  ( 65.00000000000000000, -7.395377635281828788, -7.517135062566165128E-15 ) ) ;
#28064=CIRCLE ( 'NONE', #24874, 13.57481594606304398 ) ;
#28067=CARTESIAN_POINT ( 'NONE',  ( 189.3771271284221314, 38.46992187499999716, -13.57481594606304753 ) ) ;
#28070=CARTESIAN_POINT ( 'NONE',  ( 70.44491438647230552, 38.42031250108393436, 13.14518615778179189 ) ) ;
#28077=CARTESIAN_POINT ( 'NONE',  ( -9.598844408820454532, 37.92421874999999432, 9.598844408820459861 ) ) ;
#28078=CARTESIAN_POINT ( 'NONE',  ( 124.5550856135277087, 40.60312500108393863, -13.14518615778179900 ) ) ;
#28080=CARTESIAN_POINT ( 'NONE',  ( 97.92893218813451028, 82.81250000000001421, -5.000000000000018652 ) ) ;
#28083=( BOUNDED_CURVE ( )  B_SPLINE_CURVE ( 2, ( #18677, #18538, #10231, #25089, #20955, #18941, #16249 ),
 .UNSPECIFIED., .F., .T. ) 
 B_SPLINE_CURVE_WITH_KNOTS ( ( 3, 2, 2, 3 ),
 ( 0.7500000000000006661, 0.7750000000000004663, 0.8000000000000002665, 0.8250000005912452306 ),
 .UNSPECIFIED. ) 
 CURVE ( )  GEOMETRIC_REPRESENTATION_ITEM ( )  RATIONAL_B_SPLINE_CURVE ( ( 0.9999999999999980016, 0.9238795325112887369, 1.000000000000000000, 0.9238795325112867385, 1.000000000000000000, 0.9238795325112867385, 1.000000000000000000 ) ) 
 REPRESENTATION_ITEM ( '' )  );
#28085=CARTESIAN_POINT ( 'NONE',  ( 55.70494972787295751, 35.09648437608393579, -9.295050272127046043 ) ) ;
#28086=ORIENTED_EDGE ( 'NONE', *, *, #15861, .F. ) ;
#28087=AXIS2_PLACEMENT_3D ( 'NONE', #27003, #13571, #26716 ) ;
#28088=CARTESIAN_POINT ( 'NONE',  ( -5.622872871577736298, 36.88242187499999858, -13.57481594606318254 ) ) ;
#28091=CYLINDRICAL_SURFACE ( 'NONE', #25715, 5.000000000000000888 ) ;
#28093=CARTESIAN_POINT ( 'NONE',  ( 181.4251840539369596, 37.13046875216787868, 0.000000000000000000 ) ) ;
#28096=CARTESIAN_POINT ( 'NONE',  ( 197.5295839951739651, 49.99999999938382444, 13.34625891065862291 ) ) ;
#28097=CARTESIAN_POINT ( 'NONE',  ( 116.8548138422182205, 39.16445312608393436, 0.000000000000000000 ) ) ;
#28098=ORIENTED_EDGE ( 'NONE', *, *, #6036, .F. ) ;
#28099=CARTESIAN_POINT ( 'NONE',  ( -9.295050272127046043, 38.27148437608393294, -9.295050272127046043 ) ) ;
#28100=CARTESIAN_POINT ( 'NONE',  ( 135.4449143864723055, 36.03906250108394005, 13.14518615778179189 ) ) ;
#28101=CARTESIAN_POINT ( 'NONE',  ( 65.00000000000000000, 36.43593749999999432, 13.57481594606304576 ) ) ;
#28102=CARTESIAN_POINT ( 'NONE',  ( 74.18017581364799184, 50.00000000000000000, 9.999999999999985789 ) ) ;
#28107=CARTESIAN_POINT ( 'NONE',  ( 13.57481594606304576, 39.11484375216787157, -1.662435489736055892E-15 ) ) ;
#28111=CARTESIAN_POINT ( 'NONE',  ( -8.049105076161786076E-16, 40.55351562608393579, -13.14518615778179544 ) ) ;
#28112=ORIENTED_EDGE ( 'NONE', *, *, #23634, .T. ) ;
#28115=FACE_OUTER_BOUND ( 'NONE', #26020, .T. ) ;
#28117=CARTESIAN_POINT ( 'NONE',  ( 200.4449143864723055, 38.71796875108393721, -13.14518615778179900 ) ) ;
#28118=ORIENTED_EDGE ( 'NONE', *, *, #6873, .T. ) ;
#28119=CARTESIAN_POINT ( 'NONE',  ( 65.00000000000000000, 36.18789062608393436, 13.14518615778179544 ) ) ;
#28120=DIRECTION ( 'NONE',  ( 0.000000000000000000, 0.000000000000000000, -1.000000000000000000 ) ) ;
#28122=B_SPLINE_CURVE_WITH_KNOTS ( 'NONE', 3,
 ( #17259, #25959, #15101, #4023, #19123, #4301, #6564, #3744, #27830, #8151, #21126, #1612, #10270, #18979, #27688, #16844, #6022, #6156, #14685, #23405, #739, #2866, #6846, #13680, #22114, #24384, #17540, #10970, #26532, #24244, #595 ),
 .UNSPECIFIED., .F., .F.,
 ( 4, 2, 2, 2, 2, 2, 2, 2, 2, 2, 1, 2, 2, 2, 2, 4 ),
 ( 1.256496749369840159E-15, 0.001647793485001787040, 0.003295586970002317272, 0.004943380455002847722, 0.005767277197503111429, 0.006591173940003375135, 0.008238967425003898212, 0.009886760910004423891, 0.01318234788000547872, 0.01483014136500602695, 0.01647793485000657518, 0.01812572833500712341, 0.01977352182000766817, 0.02306910879000876810, 0.02471690227500932674, 0.02636469576000988191 ),
 .UNSPECIFIED. ) ;
#28127=CARTESIAN_POINT ( 'NONE',  ( 130.0000000000000000, 32.96328125216787441, -13.57481594606304576 ) ) ;
#28128=CARTESIAN_POINT ( 'NONE',  ( 204.5988444088204403, 40.70234374999999716, -9.598844408820458085 ) ) ;
#28129=CARTESIAN_POINT ( 'NONE',  ( 189.3771271284222166, 40.85117187499999147, -13.57481594606315412 ) ) ;
#28131=CARTESIAN_POINT ( 'NONE',  ( 200.4449143864723055, 33.36015625108393579, -13.14518615778179900 ) ) ;
#28132=ORIENTED_EDGE ( 'NONE', *, *, #9309, .F. ) ;
#28139=CARTESIAN_POINT ( 'NONE',  ( 181.8548138422182205, 39.75976562608393294, 0.000000000000000000 ) ) ;
#28145=EDGE_CURVE ( 'NONE', #26695, #24077, #21758, .T. ) ;
#28147=VERTEX_POINT ( 'NONE', #12609 ) ;
#28151=CARTESIAN_POINT ( 'NONE',  ( 116.8548138422182063, 37.52734375108393294, -5.444914386472297529 ) ) ;
#28152=CARTESIAN_POINT ( 'NONE',  ( 51.85481384221819923, 32.56640625108394005, -5.444914386472297529 ) ) ;
#28154=CARTESIAN_POINT ( 'NONE',  ( 200.4449143864723055, 38.12265625108393152, -13.14518615778179900 ) ) ;
#28156=CARTESIAN_POINT ( 'NONE',  ( 5.444914386472302859, 33.65781250108393152, 13.14518615778179189 ) ) ;
#28157=CARTESIAN_POINT ( 'NONE',  ( 121.7985538123451477, 50.69246985423282581, -14.99999999999510791 ) ) ;
#28161=CARTESIAN_POINT ( 'NONE',  ( 13.14518615778179900, 34.65000000108393152, -5.444914386472297529 ) ) ;
#28164=CARTESIAN_POINT ( 'NONE',  ( 102.0710678118654897, 79.81250000273122680, -4.999999999999968914 ) ) ;
#28169=CARTESIAN_POINT ( 'NONE',  ( 99.99999999999995737, 85.00000000000000000, -3.000000000000018208 ) ) ;
#28171=CARTESIAN_POINT ( 'NONE',  ( 126.1360747348882825, 54.10645156199843342, 14.99999999999996803 ) ) ;
#28174=CARTESIAN_POINT ( 'NONE',  ( 101.8468681455906903, 80.37500000136562051, -4.458734125000016313 ) ) ;
#28175=CARTESIAN_POINT ( 'NONE',  ( 59.55508561352770158, 34.55078125108393294, 13.14518615778179722 ) ) ;
#28179=CARTESIAN_POINT ( 'NONE',  ( 2.493653234604083739E-15, 40.40468749999999432, 13.57481594606304576 ) ) ;
#28181=CARTESIAN_POINT ( 'NONE',  ( 120.7049497278729575, 31.92148437608393508, -9.295050272127046043 ) ) ;
#28187=CARTESIAN_POINT ( 'NONE',  ( 116.8548138422182063, 35.04687500108393294, 5.444914386472304635 ) ) ;
#28188=CARTESIAN_POINT ( 'NONE',  ( 55.40115559117954547, 32.46718750216787441, 9.598844408820459861 ) ) ;
#28190=VECTOR ( 'NONE', #25187, 1000.000000000000000 ) ;
#28191=CARTESIAN_POINT ( 'NONE',  ( -13.57481594606304753, 35.49335937716787015, -5.622872871577873077 ) ) ;
#28192=AXIS2_PLACEMENT_3D ( 'NONE', #23581, #1787, #10733 ) ;
#28195=CARTESIAN_POINT ( 'NONE',  ( 181.8548138422181921, 37.42812500108393436, 5.444914386472304635 ) ) ;
#28197=CARTESIAN_POINT ( 'NONE',  ( 143.1451861577818363, 36.13828125108393152, 5.444914386472293977 ) ) ;
#28198=EDGE_LOOP ( 'NONE', ( #19056, #11237, #27348, #26216 ) ) ;
#28199=CARTESIAN_POINT ( 'NONE',  ( 189.3771271284221598, 38.07304687716787583, 13.57481594606308128 ) ) ;
#28201=CARTESIAN_POINT ( 'NONE',  ( 0.000000000000000000, 50.00000000000000000, 0.000000000000000000 ) ) ;
#28203=CARTESIAN_POINT ( 'NONE',  ( 116.4251840539369596, 40.30546875216787583, 0.000000000000000000 ) ) ;
ENDSEC;
END-ISO-10303-21;
